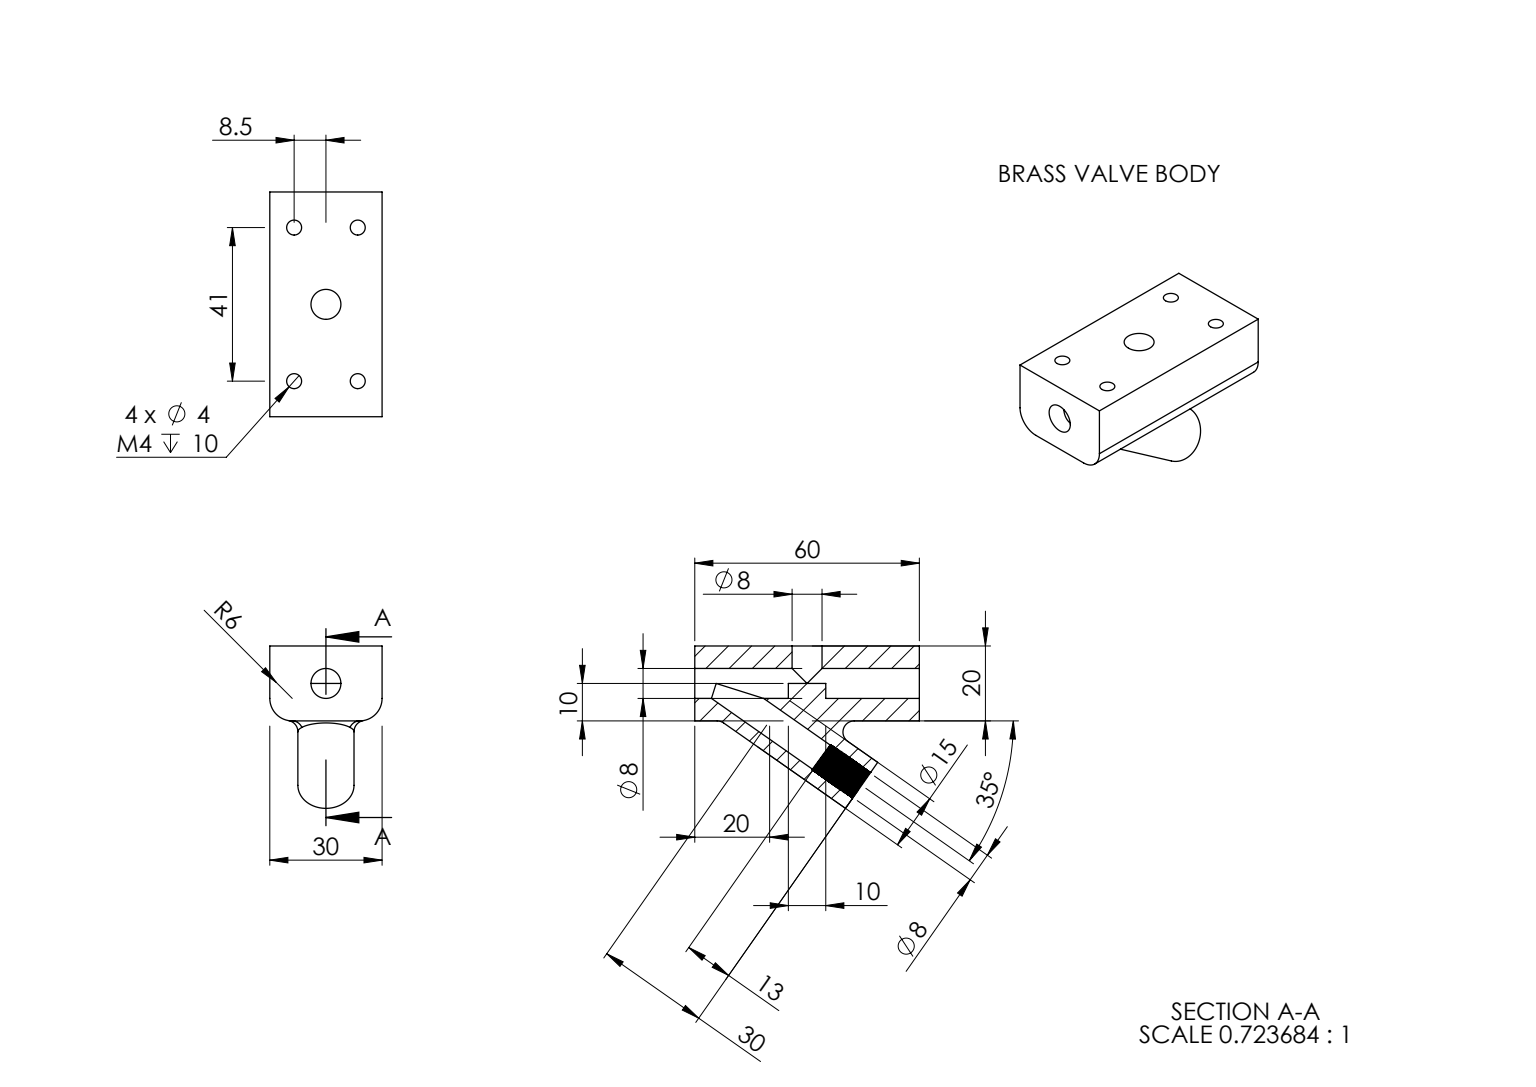
ISO-10303-21;
HEADER;
FILE_DESCRIPTION (('STEP AP214'),
    '1' );
FILE_NAME ('Brass Valve Body.step',
    '2026-10-25T16:39:07',
    ( '' ),
    ( '' ),
    'SwSTEP 2.0',
    'SolidWorks 2026',
    '' );
FILE_SCHEMA (( 'AUTOMOTIVE_DESIGN' ));
ENDSEC;

DATA;
#2=CARTESIAN_POINT ( 'NONE',  ( 2.000000000000004441, -20.45500799277048287, -10.97077568596606056 ) ) ;
#7=CARTESIAN_POINT ( 'NONE',  ( 9.986002763741593569, -9.918550557884699970, 7.302443594976057106 ) ) ;
#8=CARTESIAN_POINT ( 'NONE',  ( 2.121784821875004390, -19.91118585227123816, -10.56187548683408828 ) ) ;
#10=CARTESIAN_POINT ( 'NONE',  ( 3.579096709490575479E-14, -22.86967407583208711, -1.406012196336041020 ) ) ;
#12=ORIENTED_EDGE ( 'NONE', *, *, #11357, .T. ) ;
#15=EDGE_CURVE ( 'NONE', #13968, #17116, #3305, .T. ) ;
#18=FACE_OUTER_BOUND ( 'NONE', #18196, .T. ) ;
#22=CARTESIAN_POINT ( 'NONE',  ( 4.243569643750000786, -23.22272928460757413, -8.884014471503119736 ) ) ;
#27=CARTESIAN_POINT ( 'NONE',  ( -5.330712181944245322E-15, -26.55907985683728967, -5.105836667743160362 ) ) ;
#30=ADVANCED_FACE ( 'NONE', ( #12002 ), #4961, .F. ) ;
#35=CARTESIAN_POINT ( 'NONE',  ( -4.243569643750000786, -19.99636183013295820, -4.276284222377527477 ) ) ;
#38=ORIENTED_EDGE ( 'NONE', *, *, #726, .T. ) ;
#45=ORIENTED_EDGE ( 'NONE', *, *, #5518, .T. ) ;
#46=CARTESIAN_POINT ( 'NONE',  ( -4.243569643750000786, -20.54484429739364515, -5.059598364728879361 ) ) ;
#49=CARTESIAN_POINT ( 'NONE',  ( -2.121784821874996396, -23.22358977219849407, -15.29247854260303718 ) ) ;
#50=( BOUNDED_CURVE ( )  B_SPLINE_CURVE ( 2, ( #611, #13389, #3391, #8936, #1817, #3112, #11902, #16101, #955 ),
 .UNSPECIFIED., .F., .F. ) 
 B_SPLINE_CURVE_WITH_KNOTS ( ( 3, 2, 2, 2, 3 ),
 ( 0.3879310344827586188, 0.3908045977011494476, 0.3965517241379310498, 0.4022988505747126520, 0.4051724137931034808 ),
 .UNSPECIFIED. ) 
 CURVE ( )  GEOMETRIC_REPRESENTATION_ITEM ( )  RATIONAL_B_SPLINE_CURVE ( ( 0.9330127018922194093, 0.9330127018922194093, 1.000000000000000000, 0.8660254037844387076, 1.000000000000000000, 0.8660254037844387076, 1.000000000000000000, 0.9330127018922187432, 0.9330127018922194093 ) ) 
 REPRESENTATION_ITEM ( '' )  );
#53=DIRECTION ( 'NONE',  ( -0.000000000000000000, -0.5735764363510414965, -0.8191520442889950182 ) ) ;
#54=CARTESIAN_POINT ( 'NONE',  ( 4.243569643750003451, -22.48482328119956009, -12.10166559521431573 ) ) ;
#57=CARTESIAN_POINT ( 'NONE',  ( -1.999999999999996225, -18.15353254261686899, -7.683928109263233885 ) ) ;
#61=VECTOR ( 'NONE', #15535, 1000.000000000000000 ) ;
#62=EDGE_CURVE ( 'NONE', #4590, #2518, #8726, .T. ) ;
#63=AXIS2_PLACEMENT_3D ( 'NONE', #11586, #12802, #2984 ) ;
#64=CARTESIAN_POINT ( 'NONE',  ( 3.999999999999996447, -25.24891187463481046, -7.751385191667569785 ) ) ;
#66=EDGE_LOOP ( 'NONE', ( #4791, #2042, #17064, #10532, #9168 ) ) ;
#67=CARTESIAN_POINT ( 'NONE',  ( 2.121784821875004390, -20.71777771588989125, -11.71380804911548701 ) ) ;
#68=CARTESIAN_POINT ( 'NONE',  ( -4.000000000000000888, -26.36843755307278414, -13.37655146490396341 ) ) ;
#72=CARTESIAN_POINT ( 'NONE',  ( 1.071796769724485232, -23.37436616782919074, -2.126787201540221162 ) ) ;
#73=DIRECTION ( 'NONE',  ( -0.000000000000000000, 1.000000000000000000, -0.000000000000000000 ) ) ;
#74=AXIS2_PLACEMENT_3D ( 'NONE', #11287, #9899, #17353 ) ;
#78=CARTESIAN_POINT ( 'NONE',  ( 4.243569643749996345, -23.73478956620236957, -5.343822230353133307 ) ) ;
#79=ADVANCED_FACE ( 'NONE', ( #10984 ), #15448, .F. ) ;
#82=ORIENTED_EDGE ( 'NONE', *, *, #14672, .T. ) ;
#83=ORIENTED_EDGE ( 'NONE', *, *, #13971, .F. ) ;
#84=DIRECTION ( 'NONE',  ( -0.000000000000000000, 1.000000000000000000, -0.000000000000000000 ) ) ;
#89=CARTESIAN_POINT ( 'NONE',  ( 3.999999999999996447, -27.63642379165096941, -11.16110557702727668 ) ) ;
#93=CARTESIAN_POINT ( 'NONE',  ( 1.999999999999994449, -26.47440569391090648, -7.488412793402255296 ) ) ;
#94=VERTEX_POINT ( 'NONE', #4123 ) ;
#95=CARTESIAN_POINT ( 'NONE',  ( 0.000000000000000000, 5.977523610840987267, 32.81826849749789687 ) ) ;
#97=CARTESIAN_POINT ( 'NONE',  ( 9.570744302495992173, -9.974069202854233041, -0.5947597794661263482 ) ) ;
#98=CARTESIAN_POINT ( 'NONE',  ( -4.243569643749998122, -21.36634923031502353, -10.50431910885077791 ) ) ;
#101=CARTESIAN_POINT ( 'NONE',  ( 1.071796769724504328, -22.85814737511324424, -1.389550361680131685 ) ) ;
#102=CARTESIAN_POINT ( 'NONE',  ( 4.000000000000000888, -19.98022999250811793, -4.253245570628513939 ) ) ;
#103=EDGE_CURVE ( 'NONE', #5353, #12502, #9927, .T. ) ;
#104=ORIENTED_EDGE ( 'NONE', *, *, #5539, .F. ) ;
#105=EDGE_LOOP ( 'NONE', ( #9337, #11121, #10529, #10635, #17849 ) ) ;
#110=EDGE_LOOP ( 'NONE', ( #10063, #7100, #15621, #8878 ) ) ;
#112=CARTESIAN_POINT ( 'NONE',  ( 4.243569643750000786, -23.48083868096554028, -9.252632891433169249 ) ) ;
#116=CARTESIAN_POINT ( 'NONE',  ( 4.898587196589413815E-16, 2.700915433685006750, 35.11257424290206330 ) ) ;
#117=VECTOR ( 'NONE', #8182, 1000.000000000000000 ) ;
#118=CARTESIAN_POINT ( 'NONE',  ( -2.121784821874996396, -19.38421250137371388, -9.809279546143578443 ) ) ;
#119=CARTESIAN_POINT ( 'NONE',  ( -2.526502195916607629, -15.31622431266957207, -9.916727303590223030 ) ) ;
#120=CARTESIAN_POINT ( 'NONE',  ( -5.577813053751546416E-15, -24.16022105762193206, -3.249104295986281699 ) ) ;
#122=CARTESIAN_POINT ( 'NONE',  ( 4.243569643749996345, -22.92819770258371292, -4.191889668071731911 ) ) ;
#123=CARTESIAN_POINT ( 'NONE',  ( 1.071796769724485454, -21.36111765121935235, -13.19914471043622228 ) ) ;
#125=ORIENTED_EDGE ( 'NONE', *, *, #9998, .T. ) ;
#127=CARTESIAN_POINT ( 'NONE',  ( -5.577813053751546416E-15, -25.38624068961733826, -5.000041789647243107 ) ) ;
#129=CYLINDRICAL_SURFACE ( 'NONE', #10158, 6.000000000000000000 ) ;
#133=CARTESIAN_POINT ( 'NONE',  ( 2.121784821875004390, -17.62046495959427261, -7.290387009954915953 ) ) ;
#135=CARTESIAN_POINT ( 'NONE',  ( -4.000000000000000888, -19.85117529432912775, -4.068936360663492735 ) ) ;
#138=CARTESIAN_POINT ( 'NONE',  ( -4.243569643749998122, -23.17311500482080433, -13.08464804836111206 ) ) ;
#143=LINE ( 'NONE', #14051, #16513 ) ;
#144=CARTESIAN_POINT ( 'NONE',  ( 4.243569643749996345, -26.79983864795324422, -9.721165967022450616 ) ) ;
#146=CARTESIAN_POINT ( 'NONE',  ( -1.999999999999996225, -17.37920435354295989, -6.578072849473089789 ) ) ;
#150=EDGE_CURVE ( 'NONE', #12707, #13230, #14438, .T. ) ;
#151=CARTESIAN_POINT ( 'NONE',  ( 0.000000000000000000, 5.977523610840987267, 32.81826849749789687 ) ) ;
#157=CARTESIAN_POINT ( 'NONE',  ( -2.121784821874996396, -21.44908767223746437, -12.75822690558396033 ) ) ;
#159=VERTEX_POINT ( 'NONE', #2476 ) ;
#161=CARTESIAN_POINT ( 'NONE',  ( 3.999999999999995559, 2.343145750507624747, 2.343145750507618086 ) ) ;
#162=CARTESIAN_POINT ( 'NONE',  ( -5.577813053751546416E-15, -26.16056887869124381, -6.105897049437384538 ) ) ;
#163=CARTESIAN_POINT ( 'NONE',  ( 1.071796769724485232, -25.37471398889850605, -4.983579954991325778 ) ) ;
#164=CARTESIAN_POINT ( 'NONE',  ( -5.577813053751546416E-15, -29.06429958842333505, -10.25285427465718868 ) ) ;
#166=CARTESIAN_POINT ( 'NONE',  ( 2.121784821874994176, -23.98544242790896774, -3.566046559362932467 ) ) ;
#171=CYLINDRICAL_SURFACE ( 'NONE', #7169, 2.000000000000001776 ) ;
#172=LINE ( 'NONE', #7581, #17268 ) ;
#177=VERTEX_POINT ( 'NONE', #8106 ) ;
#179=CARTESIAN_POINT ( 'NONE',  ( -3.999999999999997335, -21.07824655387797819, -9.847693641197304615 ) ) ;
#180=ORIENTED_EDGE ( 'NONE', *, *, #14181, .F. ) ;
#184=CARTESIAN_POINT ( 'NONE',  ( -9.604277560388482016, -9.971758527880211886, 12.06915245473052778 ) ) ;
#185=CARTESIAN_POINT ( 'NONE',  ( 4.243569643750003451, -19.90372931761987019, -8.415481395913838369 ) ) ;
#194=CARTESIAN_POINT ( 'NONE',  ( 1.533898589781675205E-14, -27.70922525683905846, -8.317607569017670954 ) ) ;
#199=CARTESIAN_POINT ( 'NONE',  ( 4.730628863548789710E-15, -18.62809540513275408, -10.86517747810410306 ) ) ;
#203=FACE_OUTER_BOUND ( 'NONE', #11493, .T. ) ;
#205=DIRECTION ( 'NONE',  ( 0.000000000000000000, 0.8191520442889952403, -0.5735764363510413855 ) ) ;
#206=CARTESIAN_POINT ( 'NONE',  ( -4.243569643750005227, -25.11137301344485451, -7.309787136646725081 ) ) ;
#207=EDGE_CURVE ( 'NONE', #12141, #13551, #11942, .T. ) ;
#208=CYLINDRICAL_SURFACE ( 'NONE', #2997, 2.000000000000001776 ) ;
#211=CARTESIAN_POINT ( 'NONE',  ( -4.371749249414769167, -10.00000000000000178, -10.94697576041360954 ) ) ;
#212=DIRECTION ( 'NONE',  ( 0.000000000000000000, 0.8191520442889952403, -0.5735764363510413855 ) ) ;
#214=VECTOR ( 'NONE', #7659, 1000.000000000000000 ) ;
#215=CARTESIAN_POINT ( 'NONE',  ( 4.730628863548789710E-15, -16.82132963062697684, -8.284848538593767131 ) ) ;
#217=CARTESIAN_POINT ( 'NONE',  ( 2.000000000000004441, -17.68033198262726913, -7.008127672724814516 ) ) ;
#218=VERTEX_POINT ( 'NONE', #12642 ) ;
#220=CARTESIAN_POINT ( 'NONE',  ( 4.243569643749996345, -28.60660442245902146, -12.30149490653278121 ) ) ;
#223=CARTESIAN_POINT ( 'NONE',  ( -8.999999999999996447, -10.00000000000000000, 15.14468620625656925 ) ) ;
#224=DIRECTION ( 'NONE',  ( -6.162975822039154730E-33, 0.5735764363510414965, 0.8191520442889950182 ) ) ;
#227=ORIENTED_EDGE ( 'NONE', *, *, #6831, .F. ) ;
#228=CARTESIAN_POINT ( 'NONE',  ( 2.121784821875004390, -17.36235556323629936, -6.921768590024867329 ) ) ;
#230=CARTESIAN_POINT ( 'NONE',  ( 3.064182432158234271, -21.85725826261086624, -2.451265441397198153 ) ) ;
#233=CARTESIAN_POINT ( 'NONE',  ( 4.243569643749997233, -27.57416683702714622, -10.82702122681259205 ) ) ;
#235=CYLINDRICAL_SURFACE ( 'NONE', #4146, 4.000000000000000000 ) ;
#236=DIRECTION ( 'NONE',  ( 0.000000000000000000, 0.8191520442889952403, -0.5735764363510413855 ) ) ;
#237=CARTESIAN_POINT ( 'NONE',  ( -4.243569643750000786, -24.64233096457639505, -10.91141578111838584 ) ) ;
#240=CARTESIAN_POINT ( 'NONE',  ( -5.279047395330986450E-15, -24.40900471032784935, -2.525555542035599288 ) ) ;
#244=VERTEX_POINT ( 'NONE', #11334 ) ;
#246=FACE_OUTER_BOUND ( 'NONE', #4639, .T. ) ;
#248=CARTESIAN_POINT ( 'NONE',  ( 1.071796769724504328, -26.66526097068834034, -6.826672054641570675 ) ) ;
#251=CARTESIAN_POINT ( 'NONE',  ( 2.121784821874994176, -27.34086458056255964, -8.358086018453551702 ) ) ;
#257=CARTESIAN_POINT ( 'NONE',  ( 4.243569643750003451, -23.54952454117618288, -13.62221657742576397 ) ) ;
#259=CYLINDRICAL_SURFACE ( 'NONE', #5612, 4.000000000000000000 ) ;
#261=CARTESIAN_POINT ( 'NONE',  ( -4.243569643749997233, -19.84995652671195998, -8.338685891761748792 ) ) ;
#267=ADVANCED_FACE ( 'NONE', ( #8551 ), #11828, .T. ) ;
#269=VERTEX_POINT ( 'NONE', #1927 ) ;
#271=CARTESIAN_POINT ( 'NONE',  ( 4.898587196589413815E-16, 2.700915433685006750, 35.11257424290206330 ) ) ;
#280=CARTESIAN_POINT ( 'NONE',  ( -4.000000000000004441, -24.81872954737152170, -7.137021158450828295 ) ) ;
#281=ORIENTED_EDGE ( 'NONE', *, *, #17408, .F. ) ;
#285=CARTESIAN_POINT ( 'NONE',  ( -9.667409818421043965, -9.963321348641603237, 0.1620040674102612710 ) ) ;
#287=CARTESIAN_POINT ( 'NONE',  ( 4.243569643749997233, -22.92819770258370582, -4.191889668071731911 ) ) ;
#288=AXIS2_PLACEMENT_3D ( 'NONE', #11365, #11189, #12854 ) ;
#292=ORIENTED_EDGE ( 'NONE', *, *, #6272, .T. ) ;
#299=CARTESIAN_POINT ( 'NONE',  ( -1.071796769724494114, -29.59204508185809956, -11.00655294917319971 ) ) ;
#300=CARTESIAN_POINT ( 'NONE',  ( 4.730628863548789710E-15, -19.14431419784869348, -11.60241431796419853 ) ) ;
#305=CARTESIAN_POINT ( 'NONE',  ( -4.000000000000000888, -27.07823839235225094, -14.39025211870482934 ) ) ;
#306=CARTESIAN_POINT ( 'NONE',  ( 4.243569643750003451, -20.19410238852258743, -8.830177118335141628 ) ) ;
#307=DIRECTION ( 'NONE',  ( -0.000000000000000000, -0.5735764363510414965, -0.8191520442889950182 ) ) ;
#308=CARTESIAN_POINT ( 'NONE',  ( -4.193264170084745501, -10.00000000000000178, -2.677076674081568797 ) ) ;
#312=ORIENTED_EDGE ( 'NONE', *, *, #6152, .T. ) ;
#313=CARTESIAN_POINT ( 'NONE',  ( -5.330712181944245322E-15, -24.20383161507082193, -1.742193585881474771 ) ) ;
#315=FACE_OUTER_BOUND ( 'NONE', #13052, .T. ) ;
#316=DIRECTION ( 'NONE',  ( 0.000000000000000000, 0.000000000000000000, 1.000000000000000000 ) ) ;
#317=VERTEX_POINT ( 'NONE', #16194 ) ;
#320=CARTESIAN_POINT ( 'NONE',  ( 2.121784821874994176, -29.88969486959749844, -11.99819291526277532 ) ) ;
#324=CARTESIAN_POINT ( 'NONE',  ( 3.820650143297091184, -10.00000000000057376, -3.109998371641698345 ) ) ;
#326=CARTESIAN_POINT ( 'NONE',  ( -2.121784821874996396, -17.57744672686793308, -7.228950606633243403 ) ) ;
#329=CARTESIAN_POINT ( 'NONE',  ( 2.121784821874994176, -29.66384914778427628, -11.67565179782398310 ) ) ;
#330=( BOUNDED_CURVE ( )  B_SPLINE_CURVE ( 2, ( #8971, #16213, #4605, #6375, #1755, #13228, #14645, #544, #6189 ),
 .UNSPECIFIED., .F., .T. ) 
 B_SPLINE_CURVE_WITH_KNOTS ( ( 3, 2, 2, 2, 3 ),
 ( 0.2844827586206896686, 0.2873563218390804419, 0.2931034482758620441, 0.2988505747126437018, 0.3017241379310345306 ),
 .UNSPECIFIED. ) 
 CURVE ( )  GEOMETRIC_REPRESENTATION_ITEM ( )  RATIONAL_B_SPLINE_CURVE ( ( 0.9330127018922194093, 0.9330127018922200755, 1.000000000000000000, 0.8660254037844387076, 1.000000000000000000, 0.8660254037844387076, 1.000000000000000000, 0.9330127018922187432, 0.9330127018922194093 ) ) 
 REPRESENTATION_ITEM ( '' )  );
#332=CARTESIAN_POINT ( 'NONE',  ( 4.730628863548789710E-15, -20.95107997235447073, -14.18274325747453268 ) ) ;
#333=LINE ( 'NONE', #8939, #3459 ) ;
#336=CARTESIAN_POINT ( 'NONE',  ( 4.243569643750000786, -24.77138566275538523, -11.09572499108340793 ) ) ;
#337=EDGE_CURVE ( 'NONE', #1667, #17584, #9315, .T. ) ;
#339=CARTESIAN_POINT ( 'NONE',  ( -3.999999999999997335, -18.81978933645070384, -6.622282467816152263 ) ) ;
#342=EDGE_CURVE ( 'NONE', #5337, #15144, #10613, .T. ) ;
#349=ORIENTED_EDGE ( 'NONE', *, *, #16662, .F. ) ;
#350=CARTESIAN_POINT ( 'NONE',  ( 4.243569643749997233, -25.54155534070815392, -7.924151169863465682 ) ) ;
#352=ORIENTED_EDGE ( 'NONE', *, *, #16895, .T. ) ;
#355=CARTESIAN_POINT ( 'NONE',  ( -2.121784821875005722, -27.90010160600482081, -9.156759261635325942 ) ) ;
#357=CARTESIAN_POINT ( 'NONE',  ( -14.99999999999999645, 10.00000000000000000, -30.00000000000000000 ) ) ;
#358=CARTESIAN_POINT ( 'NONE',  ( 3.999999999999996447, -24.47458368556090491, -6.645529931877427465 ) ) ;
#359=CARTESIAN_POINT ( 'NONE',  ( -4.243569643749997233, -19.07562833763805088, -7.232830631971606472 ) ) ;
#362=DIRECTION ( 'NONE',  ( 0.000000000000000000, 0.8191520442889952403, -0.5735764363510413855 ) ) ;
#364=ORIENTED_EDGE ( 'NONE', *, *, #9762, .T. ) ;
#365=CARTESIAN_POINT ( 'NONE',  ( -3.999999999999997335, -18.56167994009273059, -6.253664047886104527 ) ) ;
#366=FACE_OUTER_BOUND ( 'NONE', #5608, .T. ) ;
#373=CARTESIAN_POINT ( 'NONE',  ( 4.713407268011036227E-15, -18.45518598442047420, -10.12789282444123451 ) ) ;
#381=CARTESIAN_POINT ( 'NONE',  ( 9.178358240570380744, -10.00000000000000000, -2.937375903338058869 ) ) ;
#383=CARTESIAN_POINT ( 'NONE',  ( -4.243569643750004339, -23.78856235711027267, -5.420617734505230878 ) ) ;
#387=ORIENTED_EDGE ( 'NONE', *, *, #14732, .T. ) ;
#397=CARTESIAN_POINT ( 'NONE',  ( -2.121784821875005722, -23.99619698609053842, -3.581405660193354379 ) ) ;
#400=CARTESIAN_POINT ( 'NONE',  ( 1.999999999999994449, -22.66729209833581749, -2.051291100440815640 ) ) ;
#402=CARTESIAN_POINT ( 'NONE',  ( 4.730628863548789710E-15, -18.91846847603547133, -11.27987320052540809 ) ) ;
#403=DIRECTION ( 'NONE',  ( -1.000000000000000000, 0.000000000000000000, 0.000000000000000000 ) ) ;
#405=VECTOR ( 'NONE', #13165, 1000.000000000000000 ) ;
#407=FACE_OUTER_BOUND ( 'NONE', #5763, .T. ) ;
#408=FACE_OUTER_BOUND ( 'NONE', #14459, .T. ) ;
#412=CARTESIAN_POINT ( 'NONE',  ( -6.938893903907228378E-15, 6.938893903907228378E-15, 30.00000000000000000 ) ) ;
#413=( NAMED_UNIT ( * ) SI_UNIT ( $, .STERADIAN. ) SOLID_ANGLE_UNIT ( ) );
#416=CARTESIAN_POINT ( 'NONE',  ( -2.121784821874996396, -22.44926158312459208, -14.18662328281289398 ) ) ;
#418=VECTOR ( 'NONE', #12172, 1000.000000000000000 ) ;
#419=DIRECTION ( 'NONE',  ( -0.000000000000000000, -0.5735764363510414965, -0.8191520442889950182 ) ) ;
#421=ORIENTED_EDGE ( 'NONE', *, *, #3365, .T. ) ;
#423=CARTESIAN_POINT ( 'NONE',  ( -2.121784821874996396, -24.03018163581715072, -16.44441110488443769 ) ) ;
#425=CARTESIAN_POINT ( 'NONE',  ( -4.243569643750004339, -27.66020330247980041, -10.94989403345594425 ) ) ;
#428=CARTESIAN_POINT ( 'NONE',  ( 4.730628863548789710E-15, -20.95107997235447073, -14.18274325747453268 ) ) ;
#430=CARTESIAN_POINT ( 'NONE',  ( -2.000000000000005773, -23.74274791649401095, -3.587201183482685352 ) ) ;
#432=ORIENTED_EDGE ( 'NONE', *, *, #4382, .T. ) ;
#434=CARTESIAN_POINT ( 'NONE',  ( -1.661723472263481630E-14, -21.09148155414254688, -12.81406445585025544 ) ) ;
#435=CARTESIAN_POINT ( 'NONE',  ( -1.999999999999996225, -22.79950167706030228, -14.31905966800409402 ) ) ;
#438=( BOUNDED_CURVE ( )  B_SPLINE_CURVE ( 2, ( #16331, #7967, #17558, #7596, #9268, #13622, #17653, #13255, #13442 ),
 .UNSPECIFIED., .F., .T. ) 
 B_SPLINE_CURVE_WITH_KNOTS ( ( 3, 2, 2, 2, 3 ),
 ( 0.5603448275862069616, 0.5632183908045976795, 0.5689655172413793371, 0.5747126436781608838, 0.5775862068965517127 ),
 .UNSPECIFIED. ) 
 CURVE ( )  GEOMETRIC_REPRESENTATION_ITEM ( )  RATIONAL_B_SPLINE_CURVE ( ( 0.9330127018922194093, 0.9330127018922206306, 1.000000000000000000, 0.8660254037844387076, 1.000000000000000000, 0.8660254037844387076, 1.000000000000000000, 0.9330127018922194093, 0.9330127018922194093 ) ) 
 REPRESENTATION_ITEM ( '' )  );
#439=ORIENTED_EDGE ( 'NONE', *, *, #5539, .T. ) ;
#440=CARTESIAN_POINT ( 'NONE',  ( -4.243569643750000786, -24.15837584640520674, -10.22025624374954766 ) ) ;
#446=CARTESIAN_POINT ( 'NONE',  ( -2.121784821875005722, -29.19064858779466221, -10.99985136128556462 ) ) ;
#447=CARTESIAN_POINT ( 'NONE',  ( -1.071796769724491671, -22.11239243885559347, -14.27207630091453261 ) ) ;
#448=DIRECTION ( 'NONE',  ( -0.000000000000000000, -0.5735764363510414965, -0.8191520442889950182 ) ) ;
#449=CARTESIAN_POINT ( 'NONE',  ( 2.000000000000004441, -19.68067980369657377, -9.864920426175917356 ) ) ;
#450=CARTESIAN_POINT ( 'NONE',  ( 2.121784821874994176, -24.75977061698287329, -4.671901819153075230 ) ) ;
#451=VERTEX_POINT ( 'NONE', #17514 ) ;
#453=CARTESIAN_POINT ( 'NONE',  ( 1.071796769724485232, -25.63282338525647575, -5.352198374921374402 ) ) ;
#455=ORIENTED_EDGE ( 'NONE', *, *, #6941, .T. ) ;
#457=DIRECTION ( 'NONE',  ( 0.000000000000000000, 0.8191520442889952403, -0.5735764363510413855 ) ) ;
#458=DIRECTION ( 'NONE',  ( 0.000000000000000000, 0.8191520442889952403, -0.5735764363510413855 ) ) ;
#463=ORIENTED_EDGE ( 'NONE', *, *, #2191, .T. ) ;
#465=CARTESIAN_POINT ( 'NONE',  ( -5.279047395330986450E-15, -26.40935253139716110, -5.382348295486703016 ) ) ;
#470=CARTESIAN_POINT ( 'NONE',  ( -4.243569643750000786, -21.28690881192279960, -6.119376322027766157 ) ) ;
#472=CARTESIAN_POINT ( 'NONE',  ( 1.071796769724495224, -16.65062116698148031, -6.471858545706086652 ) ) ;
#476=CARTESIAN_POINT ( 'NONE',  ( 4.253155871621279616, -10.96494312749350186, 19.45022984308079472 ) ) ;
#478=DIRECTION ( 'NONE',  ( -0.000000000000000000, -0.5735764363510414965, -0.8191520442889950182 ) ) ;
#479=CARTESIAN_POINT ( 'NONE',  ( 4.898587196589417759E-16, -3.999999999999993339, 25.54267522293723758 ) ) ;
#485=CARTESIAN_POINT ( 'NONE',  ( 4.730628863548789710E-15, -16.82132963062697684, -8.284848538593767131 ) ) ;
#488=CARTESIAN_POINT ( 'NONE',  ( 4.243569643749997233, -28.89697749336173871, -12.71619062895408803 ) ) ;
#489=CARTESIAN_POINT ( 'NONE',  ( -4.000000000000004441, -28.17415170002511360, -11.92906061754144886 ) ) ;
#491=ADVANCED_FACE ( 'NONE', ( #892 ), #2289, .F. ) ;
#492=CARTESIAN_POINT ( 'NONE',  ( -4.243569643750000786, -21.83539127918348299, -6.902690464379118040 ) ) ;
#495=CARTESIAN_POINT ( 'NONE',  ( -0.3267727178421339085, -10.00000000000000178, -5.052762561669631225 ) ) ;
#496=FACE_OUTER_BOUND ( 'NONE', #17631, .T. ) ;
#499=ORIENTED_EDGE ( 'NONE', *, *, #6216, .T. ) ;
#500=CARTESIAN_POINT ( 'NONE',  ( 2.121784821874994176, -22.92074116793234140, -2.045495577151484223 ) ) ;
#501=CARTESIAN_POINT ( 'NONE',  ( -6.428571428571423496, -11.73421655796351892, 14.25837509840161310 ) ) ;
#502=DIRECTION ( 'NONE',  ( -0.000000000000000000, 1.000000000000000000, -0.000000000000000000 ) ) ;
#503=ORIENTED_EDGE ( 'NONE', *, *, #11462, .F. ) ;
#505=( NAMED_UNIT ( * ) SI_UNIT ( $, .STERADIAN. ) SOLID_ANGLE_UNIT ( ) );
#506=EDGE_CURVE ( 'NONE', #17004, #8682, #13300, .T. ) ;
#507=CIRCLE ( 'NONE', #12335, 4.000000000000000000 ) ;
#508=CARTESIAN_POINT ( 'NONE',  ( -4.243569643750000786, -26.19098734272420614, -13.12312630069867225 ) ) ;
#511=CARTESIAN_POINT ( 'NONE',  ( 4.757769075324610242, -14.90261145393154862, -7.125238870422657911 ) ) ;
#514=CARTESIAN_POINT ( 'NONE',  ( 2.121784821875004390, -23.29887167946958115, -15.39999224841596437 ) ) ;
#517=CARTESIAN_POINT ( 'NONE',  ( 2.121784821875004390, -21.20173283406107956, -12.40496758648432518 ) ) ;
#519=CARTESIAN_POINT ( 'NONE',  ( -1.071796769724486786, -16.95020451169621722, -6.899707902313577002 ) ) ;
#522=CARTESIAN_POINT ( 'NONE',  ( -5.330712181944245322E-15, -27.81736316408238707, -6.902851464902143519 ) ) ;
#523=CARTESIAN_POINT ( 'NONE',  ( -5.577813053751546416E-15, -25.96698683212770931, -5.829433235496615850 ) ) ;
#529=CARTESIAN_POINT ( 'NONE',  ( 2.000000000000004441, -22.58441051342866857, -14.01187765139572150 ) ) ;
#530=CARTESIAN_POINT ( 'NONE',  ( 1.071796769724504328, -23.63247556418714979, -2.495405621470275559 ) ) ;
#534=CARTESIAN_POINT ( 'NONE',  ( 4.243569643750000786, -22.99688356279435197, -8.561473354064329300 ) ) ;
#536=ORIENTED_EDGE ( 'NONE', *, *, #1348, .T. ) ;
#540=CARTESIAN_POINT ( 'NONE',  ( -4.243569643749997233, -23.97970686843945742, -14.23658061064251257 ) ) ;
#541=CARTESIAN_POINT ( 'NONE',  ( 1.999999999999994449, -29.57171845020653222, -11.91183383256282724 ) ) ;
#542=DIRECTION ( 'NONE',  ( -1.000000000000000000, -0.000000000000000000, -0.000000000000000000 ) ) ;
#544=CARTESIAN_POINT ( 'NONE',  ( -1.071796769724486564, -28.23697075027383008, -9.071306243533678426 ) ) ;
#545=CARTESIAN_POINT ( 'NONE',  ( 4.243569643750000786, -20.15768020285669593, -4.506670734833804204 ) ) ;
#547=CARTESIAN_POINT ( 'NONE',  ( -4.000000000000000888, -23.52923419313512454, -9.321748845673438311 ) ) ;
#548=EDGE_CURVE ( 'NONE', #8360, #17559, #7326, .T. ) ;
#549=CARTESIAN_POINT ( 'NONE',  ( 4.000000000000000888, -22.88396070224021273, -8.400202795848317194 ) ) ;
#553=( BOUNDED_CURVE ( )  B_SPLINE_CURVE ( 2, ( #11093, #6833, #15203, #6742, #11181, #13792, #1101, #18087, #9699 ),
 .UNSPECIFIED., .F., .T. ) 
 B_SPLINE_CURVE_WITH_KNOTS ( ( 3, 2, 2, 2, 3 ),
 ( 0.9051724137931034253, 0.9080459770114942541, 0.9137931034482759118, 0.9195402298850574585, 0.9224137931034482873 ),
 .UNSPECIFIED. ) 
 CURVE ( )  GEOMETRIC_REPRESENTATION_ITEM ( )  RATIONAL_B_SPLINE_CURVE ( ( 0.9330127018922194093, 0.9330127018922194093, 1.000000000000000000, 0.8660254037844387076, 1.000000000000000000, 0.8660254037844387076, 1.000000000000000000, 0.9330127018922194093, 0.9330127018922194093 ) ) 
 REPRESENTATION_ITEM ( '' )  );
#556=DIRECTION ( 'NONE',  ( 0.000000000000000000, 0.8191520442889952403, -0.5735764363510413855 ) ) ;
#560=EDGE_CURVE ( 'NONE', #14256, #10497, #11069, .T. ) ;
#566=CARTESIAN_POINT ( 'NONE',  ( 4.713407268011036227E-15, -18.97140477713641005, -10.86512966430133176 ) ) ;
#570=CARTESIAN_POINT ( 'NONE',  ( 1.071796769724485454, -20.52226211235100806, -12.00113484465680358 ) ) ;
#571=CARTESIAN_POINT ( 'NONE',  ( -4.243569643749998122, -19.55958345580924629, -7.923990169340444645 ) ) ;
#574=CARTESIAN_POINT ( 'NONE',  ( 3.999999999999996447, -28.41075198072487140, -12.26696083681741989 ) ) ;
#576=ORIENTED_EDGE ( 'NONE', *, *, #8996, .F. ) ;
#577=CARTESIAN_POINT ( 'NONE',  ( 2.531783071939769592, -10.67720498481739355, 21.39218517664858510 ) ) ;
#578=CARTESIAN_POINT ( 'NONE',  ( 0.000000000000000000, 5.977523610840987267, 32.81826849749789687 ) ) ;
#581=ORIENTED_EDGE ( 'NONE', *, *, #2191, .F. ) ;
#584=CARTESIAN_POINT ( 'NONE',  ( 4.243569643749996345, -23.18630709894168263, -4.560508088001781424 ) ) ;
#587=CARTESIAN_POINT ( 'NONE',  ( 4.243569643749997233, -28.38075870064580286, -11.97895378909399078 ) ) ;
#588=CARTESIAN_POINT ( 'NONE',  ( 1.999999999999994449, -29.31360905384856608, -11.54321541263277950 ) ) ;
#589=VECTOR ( 'NONE', #2601, 1000.000000000000000 ) ;
#590=CARTESIAN_POINT ( 'NONE',  ( 2.121784821875004390, -18.13668375231020846, -8.027623849815011425 ) ) ;
#595=ORIENTED_EDGE ( 'NONE', *, *, #1110, .F. ) ;
#598=CARTESIAN_POINT ( 'NONE',  ( 4.299564228933482956E-15, -17.41342265533655009, -7.561251970840314307 ) ) ;
#600=ORIENTED_EDGE ( 'NONE', *, *, #8861, .F. ) ;
#604=CARTESIAN_POINT ( 'NONE',  ( 4.730628863548789710E-15, -22.24162695414431212, -16.02583535712476959 ) ) ;
#607=CARTESIAN_POINT ( 'NONE',  ( 2.121784821875004390, -22.00832469767973620, -13.55690014876572569 ) ) ;
#609=EDGE_CURVE ( 'NONE', #1376, #8485, #13946, .T. ) ;
#611=CARTESIAN_POINT ( 'NONE',  ( 4.299564228933482956E-15, -21.02695420434810814, -12.72190984986098172 ) ) ;
#613=CARTESIAN_POINT ( 'NONE',  ( 2.121784821874994176, -27.05049150965984595, -7.943390296032248443 ) ) ;
#615=ADVANCED_FACE ( 'NONE', ( #13762 ), #4118, .F. ) ;
#618=CARTESIAN_POINT ( 'NONE',  ( 4.243569643749996345, -25.25118226980542602, -7.509455447442161535 ) ) ;
#619=ORIENTED_EDGE ( 'NONE', *, *, #1520, .F. ) ;
#620=CYLINDRICAL_SURFACE ( 'NONE', #17533, 4.000000000000000000 ) ;
#621=CARTESIAN_POINT ( 'NONE',  ( 2.610817454768295409, -22.11373505648317916, -1.875566028523329098 ) ) ;
#625=DIRECTION ( 'NONE',  ( -0.000000000000000000, -0.5735764363510414965, -0.8191520442889950182 ) ) ;
#627=AXIS2_PLACEMENT_3D ( 'NONE', #9610, #15282, #8214 ) ;
#632=CARTESIAN_POINT ( 'NONE',  ( 4.243569643750000786, -22.48066477007841613, -7.824236514204232940 ) ) ;
#637=CARTESIAN_POINT ( 'NONE',  ( -4.243569643750005227, -26.91813878795063886, -9.890116076157061897 ) ) ;
#638=CARTESIAN_POINT ( 'NONE',  ( -6.158835246850665095E-15, -22.12391913957442213, -14.28853813557044639 ) ) ;
#639=B_SPLINE_CURVE_WITH_KNOTS ( 'NONE', 1,
 ( #5800, #5891 ),
 .UNSPECIFIED., .F., .F.,
 ( 2, 2 ),
 ( 0.000000000000000000, 1.000000000000000000 ),
 .UNSPECIFIED. ) ;
#640=AXIS2_PLACEMENT_3D ( 'NONE', #16166, #307, #1699 ) ;
#641=CARTESIAN_POINT ( 'NONE',  ( 7.381087143211832569, -10.35722647083040826, 4.976872143527621084 ) ) ;
#642=CARTESIAN_POINT ( 'NONE',  ( -4.243569643750000786, -26.96531553179811169, -14.22898156048881724 ) ) ;
#643=ORIENTED_EDGE ( 'NONE', *, *, #13613, .T. ) ;
#645=CARTESIAN_POINT ( 'NONE',  ( 1.999999999999994449, -26.02271425098940938, -6.843330559531437984 ) ) ;
#647=ORIENTED_EDGE ( 'NONE', *, *, #2644, .T. ) ;
#649=CYLINDRICAL_SURFACE ( 'NONE', #8066, 4.000000000000000000 ) ;
#656=CARTESIAN_POINT ( 'NONE',  ( -2.000000000000005773, -24.45254875577348130, -4.600901837283550400 ) ) ;
#657=ORIENTED_EDGE ( 'NONE', *, *, #883, .F. ) ;
#661=CARTESIAN_POINT ( 'NONE',  ( -2.121784821875005722, -23.22186879701663642, -2.475550400403212503 ) ) ;
#662=( BOUNDED_CURVE ( )  B_SPLINE_CURVE ( 2, ( #13922, #1231, #6865, #12609, #13733, #12521, #9559, #14007, #12431 ),
 .UNSPECIFIED., .F., .F. ) 
 B_SPLINE_CURVE_WITH_KNOTS ( ( 3, 2, 2, 2, 3 ),
 ( 0.3534482758620690057, 0.3563218390804597790, 0.3620689655172413812, 0.3678160919540229834, 0.3706896551724138122 ),
 .UNSPECIFIED. ) 
 CURVE ( )  GEOMETRIC_REPRESENTATION_ITEM ( )  RATIONAL_B_SPLINE_CURVE ( ( 0.9330127018922194093, 0.9330127018922200755, 1.000000000000000000, 0.8660254037844387076, 1.000000000000000000, 0.8660254037844387076, 1.000000000000000000, 0.9330127018922187432, 0.9330127018922194093 ) ) 
 REPRESENTATION_ITEM ( '' )  );
#663=CARTESIAN_POINT ( 'NONE',  ( 2.121784821874994176, -27.34086458056255964, -8.358086018453551702 ) ) ;
#665=CARTESIAN_POINT ( 'NONE',  ( 2.170367169212293224, -29.75460566901168491, -12.32900594437920816 ) ) ;
#666=EDGE_LOOP ( 'NONE', ( #3881, #11701, #9259, #14886 ) ) ;
#667=CARTESIAN_POINT ( 'NONE',  ( -4.772237607920192026, -11.09252097142725901, 18.58920227068528419 ) ) ;
#670=CARTESIAN_POINT ( 'NONE',  ( 2.121784821875004390, -24.07319986854348670, -16.50584750820610580 ) ) ;
#671=EDGE_LOOP ( 'NONE', ( #1237, #16466, #3525, #5028 ) ) ;
#673=CARTESIAN_POINT ( 'NONE',  ( 3.939448708636003271, -26.33660243321148897, -14.75747596281047436 ) ) ;
#674=CARTESIAN_POINT ( 'NONE',  ( -5.330712181944245322E-15, -24.97815980414473103, -2.848048845671618423 ) ) ;
#679=CARTESIAN_POINT ( 'NONE',  ( -4.243569643750000786, -26.99757920634285924, -14.27505886298007276 ) ) ;
#680=CARTESIAN_POINT ( 'NONE',  ( -2.000000000000005773, -28.58229909750097875, -10.49879655616431506 ) ) ;
#682=CARTESIAN_POINT ( 'NONE',  ( 4.243569643750000786, -21.96444597736247673, -7.086999674344137468 ) ) ;
#684=EDGE_CURVE ( 'NONE', #10458, #6378, #13728, .T. ) ;
#687=CARTESIAN_POINT ( 'NONE',  ( 3.999999999999997780, -28.14205403674597861, -13.39922821167334810 ) ) ;
#689=CARTESIAN_POINT ( 'NONE',  ( 1.999999999999994449, -25.50649545827347353, -6.106093719671341624 ) ) ;
#690=ORIENTED_EDGE ( 'NONE', *, *, #8744, .T. ) ;
#691=EDGE_LOOP ( 'NONE', ( #11697, #16402, #8918, #16963 ) ) ;
#693=CARTESIAN_POINT ( 'NONE',  ( 4.000000000000003553, -18.84129845210892640, -6.653000668470220980 ) ) ;
#695=ORIENTED_EDGE ( 'NONE', *, *, #6775, .F. ) ;
#697=CARTESIAN_POINT ( 'NONE',  ( 4.243569643750003451, -23.00104207391549593, -12.83890243507441120 ) ) ;
#700=CARTESIAN_POINT ( 'NONE',  ( -0.5181399714674771451, -9.999999999997587707, -3.173488174254735839 ) ) ;
#701=CIRCLE ( 'NONE', #17888, 2.000000000000001776 ) ;
#702=CARTESIAN_POINT ( 'NONE',  ( -4.243569643750000786, -25.19081343183707844, -11.69472992346973861 ) ) ;
#703=CARTESIAN_POINT ( 'NONE',  ( 2.121784821874994176, -27.30860090601781209, -8.312008715962296179 ) ) ;
#704=CARTESIAN_POINT ( 'NONE',  ( -6.938893903907228378E-15, 6.938893903907228378E-15, -4.999999999999997335 ) ) ;
#705=CARTESIAN_POINT ( 'NONE',  ( -4.000000000000004441, -22.04405353722830085, -3.174373145209581804 ) ) ;
#707=CARTESIAN_POINT ( 'NONE',  ( -2.121784821875005722, -26.31918155331226217, -6.898971439563784003 ) ) ;
#710=CARTESIAN_POINT ( 'NONE',  ( -3.999999999999997335, -17.78735175101882859, -5.147808788095962207 ) ) ;
#712=EDGE_LOOP ( 'NONE', ( #2767, #16521, #3729, #8436, #3326, #6869 ) ) ;
#714=CARTESIAN_POINT ( 'NONE',  ( 4.000000000000000888, -23.91639828767208442, -9.874676475568506362 ) ) ;
#715=ADVANCED_FACE ( 'NONE', ( #15445, #17962, #11152, #8375, #10887, #18056 ), #6533, .F. ) ;
#717=CARTESIAN_POINT ( 'NONE',  ( 9.000000000000005329, -12.99999999999999822, -3.713574246709343996 ) ) ;
#718=EDGE_CURVE ( 'NONE', #4345, #7195, #15626, .T. ) ;
#720=CARTESIAN_POINT ( 'NONE',  ( 2.121784821874994176, -25.53409880605677884, -5.777757078943218438 ) ) ;
#726=EDGE_CURVE ( 'NONE', #17169, #13482, #4570, .T. ) ;
#727=CARTESIAN_POINT ( 'NONE',  ( 3.999999999999996447, -23.44214610012902966, -5.171056252157234745 ) ) ;
#731=CARTESIAN_POINT ( 'NONE',  ( 7.143010269575600368, -13.70175065102395706, 0.6871907070005838225 ) ) ;
#733=CARTESIAN_POINT ( 'NONE',  ( 2.121784821875004390, -17.10424616687832966, -6.553150170094818705 ) ) ;
#737=CARTESIAN_POINT ( 'NONE',  ( 2.000000000000004441, -20.26142594620695192, -10.69431187202529010 ) ) ;
#740=CARTESIAN_POINT ( 'NONE',  ( -4.000000000000000888, -21.39983167247694240, -6.280646880243780039 ) ) ;
#748=CARTESIAN_POINT ( 'NONE',  ( -5.279047395330986450E-15, -25.89313373868122881, -4.645111455626608432 ) ) ;
#749=ORIENTED_EDGE ( 'NONE', *, *, #8614, .F. ) ;
#750=LINE ( 'NONE', #16234, #7968 ) ;
#753=CARTESIAN_POINT ( 'NONE',  ( -2.121784821874996396, -16.77085486324927999, -6.077018044351843784 ) ) ;
#754=CARTESIAN_POINT ( 'NONE',  ( 2.121784821875004390, -21.23399650860583066, -12.45104488897558248 ) ) ;
#755=EDGE_CURVE ( 'NONE', #12418, #4334, #3095, .T. ) ;
#756=CARTESIAN_POINT ( 'NONE',  ( 3.999999999999993339, 7.428752623566170548E-15, -30.00000000000000000 ) ) ;
#758=CARTESIAN_POINT ( 'NONE',  ( -2.978814741686234946, -10.00000000000083844, 22.09987478886784018 ) ) ;
#761=CARTESIAN_POINT ( 'NONE',  ( 4.243569643749996345, -28.38075870064580286, -11.97895378909399078 ) ) ;
#762=ORIENTED_EDGE ( 'NONE', *, *, #13111, .F. ) ;
#765=CARTESIAN_POINT ( 'NONE',  ( 4.243569643750003451, -19.64561992126190049, -8.046862975983790633 ) ) ;
#768=CARTESIAN_POINT ( 'NONE',  ( 4.243569643750003451, -23.80763393753414903, -13.99083499735581171 ) ) ;
#769=CARTESIAN_POINT ( 'NONE',  ( 3.999999999999996447, -27.83000583821450036, -11.43756939096804714 ) ) ;
#770=CARTESIAN_POINT ( 'NONE',  ( 4.243569643750000786, -21.19011778828857118, -5.981144414553994260 ) ) ;
#773=CARTESIAN_POINT ( 'NONE',  ( 4.000000000000000888, -26.94918369417327142, -14.20594290873980192 ) ) ;
#774=FACE_OUTER_BOUND ( 'NONE', #8330, .T. ) ;
#778=EDGE_CURVE ( 'NONE', #16888, #7294, #3002, .T. ) ;
#780=CARTESIAN_POINT ( 'NONE',  ( 6.428571428571432378, -14.26578344203647752, -2.827263138854379410 ) ) ;
#781=ORIENTED_EDGE ( 'NONE', *, *, #883, .T. ) ;
#783=CARTESIAN_POINT ( 'NONE',  ( -2.121784821874996396, -21.93304279040865623, -13.44938644295279850 ) ) ;
#787=CARTESIAN_POINT ( 'NONE',  ( 5.562324373799151900, -10.00000000000000000, -9.830817939999416666 ) ) ;
#788=CARTESIAN_POINT ( 'NONE',  ( -2.121784821874996396, -22.73963465402730577, -14.60131900523419901 ) ) ;
#792=CARTESIAN_POINT ( 'NONE',  ( -1.071796769724496334, -29.52751773206367147, -10.91439834318392244 ) ) ;
#794=AXIS2_PLACEMENT_3D ( 'NONE', #18164, #18343, #14049 ) ;
#795=CARTESIAN_POINT ( 'NONE',  ( 4.243569643750000786, -23.73894807732350998, -9.621251311363216985 ) ) ;
#796=ORIENTED_EDGE ( 'NONE', *, *, #7337, .T. ) ;
#803=CARTESIAN_POINT ( 'NONE',  ( -2.000000000000005773, -22.90389237762567021, -2.389191317703265316 ) ) ;
#807=CARTESIAN_POINT ( 'NONE',  ( -4.243569643749998122, -20.10806592306992613, -8.707304311691796528 ) ) ;
#810=ORIENTED_EDGE ( 'NONE', *, *, #506, .F. ) ;
#813=EDGE_CURVE ( 'NONE', #18256, #8328, #1525, .T. ) ;
#814=CARTESIAN_POINT ( 'NONE',  ( -2.072127310227394492, -24.23032511484031915, -16.43161913306204980 ) ) ;
#815=CARTESIAN_POINT ( 'NONE',  ( 7.710291887657668930, -10.24552755907163970, 9.424636009669162817 ) ) ;
#816=CARTESIAN_POINT ( 'NONE',  ( -2.000000000000005773, -24.51707610556791650, -4.693056443272829448 ) ) ;
#817=CARTESIAN_POINT ( 'NONE',  ( 2.121784821874994176, -23.21111423883506220, -2.460191299572788814 ) ) ;
#819=ORIENTED_EDGE ( 'NONE', *, *, #9426, .F. ) ;
#821=CARTESIAN_POINT ( 'NONE',  ( -4.000000000000004441, -24.36703810445001750, -6.491938924580010983 ) ) ;
#825=CIRCLE ( 'NONE', #3186, 2.000000000000001776 ) ;
#826=ORIENTED_EDGE ( 'NONE', *, *, #2587, .F. ) ;
#834=CARTESIAN_POINT ( 'NONE',  ( -5.279047395330986450E-15, -24.60258675689138386, -2.802019355976369752 ) ) ;
#836=TOROIDAL_SURFACE ( 'NONE', #2897, 4.400000000000002132, 0.4000000000000000222 ) ;
#840=ADVANCED_FACE ( 'NONE', ( #315 ), #18327, .F. ) ;
#841=DIRECTION ( 'NONE',  ( -0.3258630558627232943, 0.000000000000000000, 0.9454169814551713902 ) ) ;
#843=CARTESIAN_POINT ( 'NONE',  ( 4.243569643750003451, -18.61318233583002879, -6.572389296263599689 ) ) ;
#845=CARTESIAN_POINT ( 'NONE',  ( 4.243569643750003451, -22.77519635210228088, -12.51636131763562076 ) ) ;
#846=CARTESIAN_POINT ( 'NONE',  ( 4.299564228933482956E-15, -23.15635672500629738, -15.76301181529063555 ) ) ;
#848=CARTESIAN_POINT ( 'NONE',  ( 6.903430137609765538, -10.00000000000000178, 15.77881270003217828 ) ) ;
#850=FACE_OUTER_BOUND ( 'NONE', #998, .T. ) ;
#851=VERTEX_POINT ( 'NONE', #6424 ) ;
#853=AXIS2_PLACEMENT_3D ( 'NONE', #2448, #17847, #13464 ) ;
#854=CARTESIAN_POINT ( 'NONE',  ( -4.243569643750000786, -20.51258062284889760, -5.013521062237622949 ) ) ;
#857=CARTESIAN_POINT ( 'NONE',  ( 2.000000000000004441, -22.00366437091829397, -13.18248620554634698 ) ) ;
#858=ORIENTED_EDGE ( 'NONE', *, *, #7727, .T. ) ;
#859=CARTESIAN_POINT ( 'NONE',  ( -4.243569643749997233, -19.84995652671195998, -8.338685891761748792 ) ) ;
#865=CARTESIAN_POINT ( 'NONE',  ( 1.071796769724485232, -25.95546013140888064, -5.812971400840699410 ) ) ;
#869=CARTESIAN_POINT ( 'NONE',  ( 3.579096709490575479E-14, -24.93454924669583406, -4.354959555776423130 ) ) ;
#874=SURFACE_SIDE_STYLE ('',( #12074 ) ) ;
#875=CARTESIAN_POINT ( 'NONE',  ( -4.243569643749997233, -22.65689621210486138, -12.34741120850101836 ) ) ;
#880=CARTESIAN_POINT ( 'NONE',  ( -1.006530391518317247, -10.00000000000122213, -4.211315095027532429 ) ) ;
#881=CARTESIAN_POINT ( 'NONE',  ( -4.243569643750000786, -25.70703222455301784, -12.43196676332983408 ) ) ;
#883=EDGE_CURVE ( 'NONE', #15966, #8825, #1892, .T. ) ;
#886=CARTESIAN_POINT ( 'NONE',  ( -4.000000000000000888, -20.17381204048153265, -4.529709386582819519 ) ) ;
#887=DIRECTION ( 'NONE',  ( -0.000000000000000000, 1.000000000000000000, -0.000000000000000000 ) ) ;
#888=CARTESIAN_POINT ( 'NONE',  ( -4.243569643749997233, -20.85013043759908413, -9.767082268990684213 ) ) ;
#890=ADVANCED_FACE ( 'NONE', ( #11889 ), #10502, .F. ) ;
#892=FACE_OUTER_BOUND ( 'NONE', #14880, .T. ) ;
#899=DIRECTION ( 'NONE',  ( 0.000000000000000000, 0.8191520442889952403, -0.5735764363510413855 ) ) ;
#901=CARTESIAN_POINT ( 'NONE',  ( 4.730628863548789710E-15, -19.17657787239343747, -11.64849162045545405 ) ) ;
#911=CARTESIAN_POINT ( 'NONE',  ( 4.730628863548789710E-15, -23.01595514321822122, -17.13169061691491279 ) ) ;
#913=CARTESIAN_POINT ( 'NONE',  ( 2.000000000000004441, -20.51953534256492162, -11.06293029195533784 ) ) ;
#916=ORIENTED_EDGE ( 'NONE', *, *, #8515, .T. ) ;
#918=CARTESIAN_POINT ( 'NONE',  ( -5.577813053751546416E-15, -28.80619019206536535, -9.884235854727139170 ) ) ;
#925=CARTESIAN_POINT ( 'NONE',  ( 4.000000000000003553, -18.58318905575096025, -6.284382248540171467 ) ) ;
#926=ORIENTED_EDGE ( 'NONE', *, *, #4785, .F. ) ;
#930=( BOUNDED_CURVE ( )  B_SPLINE_CURVE ( 2, ( #9246, #10541, #11939, #16216, #3511, #3596, #2401, #14834, #16403 ),
 .UNSPECIFIED., .F., .T. ) 
 B_SPLINE_CURVE_WITH_KNOTS ( ( 3, 2, 2, 2, 3 ),
 ( 0.5086206896551724865, 0.5114942528735632044, 0.5172413793103448620, 0.5229885057471264087, 0.5258620689655172376 ),
 .UNSPECIFIED. ) 
 CURVE ( )  GEOMETRIC_REPRESENTATION_ITEM ( )  RATIONAL_B_SPLINE_CURVE ( ( 0.9330127018922194093, 0.9330127018922206306, 1.000000000000000000, 0.8660254037844387076, 1.000000000000000000, 0.8660254037844387076, 1.000000000000000000, 0.9330127018922194093, 0.9330127018922194093 ) ) 
 REPRESENTATION_ITEM ( '' )  );
#931=LINE ( 'NONE', #5180, #9055 ) ;
#932=CARTESIAN_POINT ( 'NONE',  ( 4.243569643750000786, -20.64163532102788778, -5.197830272202643265 ) ) ;
#933=CARTESIAN_POINT ( 'NONE',  ( 4.243569643749996345, -26.57399292614002562, -9.398624849583658403 ) ) ;
#934=CARTESIAN_POINT ( 'NONE',  ( 2.659568448039375088, -29.44477373260542663, -12.53330527340647471 ) ) ;
#937=CARTESIAN_POINT ( 'NONE',  ( -3.772879157352762913, -10.00000000000000178, -12.59063537424807677 ) ) ;
#938=CARTESIAN_POINT ( 'NONE',  ( -2.000000000000005773, -25.48498634120535655, -6.075375517003743120 ) ) ;
#939=CARTESIAN_POINT ( 'NONE',  ( -4.000000000000004441, -24.62514750080798720, -6.860557344510057831 ) ) ;
#943=CARTESIAN_POINT ( 'NONE',  ( 2.000000000000004441, -24.13306689157648321, -16.22358817097600436 ) ) ;
#947=EDGE_CURVE ( 'NONE', #14660, #16355, #5656, .T. ) ;
#948=CARTESIAN_POINT ( 'NONE',  ( -4.000000000000000888, -24.49714442877256459, -10.70406791940435198 ) ) ;
#949=ORIENTED_EDGE ( 'NONE', *, *, #17401, .F. ) ;
#950=EDGE_CURVE ( 'NONE', #1446, #1376, #14215, .T. ) ;
#951=CARTESIAN_POINT ( 'NONE',  ( 4.243569643749996345, -21.92802379169658877, -2.763493290842798267 ) ) ;
#955=CARTESIAN_POINT ( 'NONE',  ( 1.533898589781675205E-14, -27.45111586048108521, -7.948989149087622330 ) ) ;
#961=EDGE_LOOP ( 'NONE', ( #16910, #10250, #7255 ) ) ;
#962=ORIENTED_EDGE ( 'NONE', *, *, #14291, .T. ) ;
#967=CARTESIAN_POINT ( 'NONE',  ( 7.406012110500714840, -12.49260087798120367, 8.584195667863683710 ) ) ;
#971=CARTESIAN_POINT ( 'NONE',  ( 4.243569643750003451, -22.74293267755752623, -12.47028401514436169 ) ) ;
#975=CYLINDRICAL_SURFACE ( 'NONE', #13734, 4.000000000000000000 ) ;
#977=CARTESIAN_POINT ( 'NONE',  ( 4.243569643750000786, -26.09419631908997772, -12.98489439322490213 ) ) ;
#983=CARTESIAN_POINT ( 'NONE',  ( 4.243569643750003451, -19.38751052490393434, -7.678244556053742897 ) ) ;
#985=VERTEX_POINT ( 'NONE', #501 ) ;
#986=CARTESIAN_POINT ( 'NONE',  ( -1.071796769724487675, -23.59652146720896582, -16.39163221450554531 ) ) ;
#988=CARTESIAN_POINT ( 'NONE',  ( 3.064181913176683203, -21.66367673124435100, -2.174801284911689336 ) ) ;
#994=FACE_OUTER_BOUND ( 'NONE', #4572, .T. ) ;
#995=ORIENTED_EDGE ( 'NONE', *, *, #17161, .F. ) ;
#996=CARTESIAN_POINT ( 'NONE',  ( -2.121784821874996396, -18.09366551958387248, -7.966187446493337987 ) ) ;
#998=EDGE_LOOP ( 'NONE', ( #10590, #3435, #5889, #4242 ) ) ;
#1000=CARTESIAN_POINT ( 'NONE',  ( 4.243569643750003451, -25.06591724477924288, -15.78784979451479309 ) ) ;
#1001=CARTESIAN_POINT ( 'NONE',  ( 3.220835151890553583, -25.02781588011482938, -15.95816000315516270 ) ) ;
#1003=CARTESIAN_POINT ( 'NONE',  ( 10.00272540370463226, -9.915619283365160186, 6.515181925709914168 ) ) ;
#1005=CARTESIAN_POINT ( 'NONE',  ( 2.121784821875004390, -23.78282679764076590, -16.09115178578480254 ) ) ;
#1008=CARTESIAN_POINT ( 'NONE',  ( -4.000000000000004441, -24.10892870809205135, -6.123320504649964136 ) ) ;
#1012=CARTESIAN_POINT ( 'NONE',  ( -1.071796769724486786, -17.91811474733365372, -8.282026976044495115 ) ) ;
#1019=EDGE_CURVE ( 'NONE', #5846, #2315, #17393, .T. ) ;
#1020=CARTESIAN_POINT ( 'NONE',  ( -4.000000000000004441, -22.49574498014980151, -3.819455379080400004 ) ) ;
#1024=DIRECTION ( 'NONE',  ( 0.000000000000000000, 0.000000000000000000, 1.000000000000000000 ) ) ;
#1025=CARTESIAN_POINT ( 'NONE',  ( 4.730628863548789710E-15, -16.30511083791103744, -7.547611698733672547 ) ) ;
#1026=CARTESIAN_POINT ( 'NONE',  ( -4.243569643750005227, -24.33704482437095251, -6.203931876856584537 ) ) ;
#1035=CARTESIAN_POINT ( 'NONE',  ( -1.999999999999996225, -24.09004865885014723, -16.16215176765433270 ) ) ;
#1039=CARTESIAN_POINT ( 'NONE',  ( 4.000000000000003553, -23.22915819019439709, -12.91951380728103160 ) ) ;
#1040=( BOUNDED_CURVE ( )  B_SPLINE_CURVE ( 2, ( #17747, #2068, #2251, #9184, #3626, #939, #15037, #13627, #3540 ),
 .UNSPECIFIED., .F., .T. ) 
 B_SPLINE_CURVE_WITH_KNOTS ( ( 3, 2, 2, 2, 3 ),
 ( 0.5603448275862069616, 0.5632183908045976795, 0.5689655172413793371, 0.5747126436781608838, 0.5775862068965517127 ),
 .UNSPECIFIED. ) 
 CURVE ( )  GEOMETRIC_REPRESENTATION_ITEM ( )  RATIONAL_B_SPLINE_CURVE ( ( 0.9330127018922194093, 0.9330127018922206306, 1.000000000000000000, 0.8660254037844387076, 1.000000000000000000, 0.8660254037844387076, 1.000000000000000000, 0.9330127018922194093, 0.9330127018922194093 ) ) 
 REPRESENTATION_ITEM ( '' )  );
#1042=CARTESIAN_POINT ( 'NONE',  ( -4.243569643749997233, -18.30130014856414533, -6.126975372181463264 ) ) ;
#1044=CARTESIAN_POINT ( 'NONE',  ( 8.500000000000019540, 0.000000000000000000, -20.49999999999998934 ) ) ;
#1045=CARTESIAN_POINT ( 'NONE',  ( -5.330712181944246111E-15, -28.33358195679832292, -7.640088304762238103 ) ) ;
#1046=CARTESIAN_POINT ( 'NONE',  ( 1.999999999999994449, -29.05549965749059638, -11.17459699270273354 ) ) ;
#1047=EDGE_CURVE ( 'NONE', #3748, #10497, #9446, .T. ) ;
#1048=ADVANCED_FACE ( 'NONE', ( #15059 ), #13745, .F. ) ;
#1049=CARTESIAN_POINT ( 'NONE',  ( 3.999999999999996447, -23.24856405356550226, -4.894592438216466057 ) ) ;
#1051=CARTESIAN_POINT ( 'NONE',  ( 0.000000000000000000, 5.977523610840987267, 32.81826849749789687 ) ) ;
#1052=VERTEX_POINT ( 'NONE', #12255 ) ;
#1057=CARTESIAN_POINT ( 'NONE',  ( 3.999999999999996447, -26.02324006370871956, -8.857240451457712993 ) ) ;
#1060=CARTESIAN_POINT ( 'NONE',  ( 2.121784821875004390, -21.45984223041904926, -12.77358600641437469 ) ) ;
#1064=DIRECTION ( 'NONE',  ( -0.000000000000000000, -0.5735764363510414965, -0.8191520442889950182 ) ) ;
#1066=CARTESIAN_POINT ( 'NONE',  ( -2.121784821875005722, -27.38388281328888141, -8.419522421775232246 ) ) ;
#1069=CARTESIAN_POINT ( 'NONE',  ( -1.071796769724505882, -17.46642330441216018, -7.636944742173667144 ) ) ;
#1072=CARTESIAN_POINT ( 'NONE',  ( 2.121784821875004390, -19.39496705955529876, -9.824638646973991030 ) ) ;
#1084=CARTESIAN_POINT ( 'NONE',  ( -5.330712181944246111E-15, -25.52664227140541087, -3.631362988022969862 ) ) ;
#1087=DIRECTION ( 'NONE',  ( -0.000000000000000000, -0.5735764363510414965, -0.8191520442889950182 ) ) ;
#1089=CARTESIAN_POINT ( 'NONE',  ( 4.243569643749997233, -28.60660442245902502, -12.30149490653278121 ) ) ;
#1090=FACE_OUTER_BOUND ( 'NONE', #15810, .T. ) ;
#1092=CARTESIAN_POINT ( 'NONE',  ( -4.243569643750005227, -28.43453149155370241, -12.05574929324608924 ) ) ;
#1094=FACE_OUTER_BOUND ( 'NONE', #5867, .T. ) ;
#1095=CARTESIAN_POINT ( 'NONE',  ( 1.999999999999994449, -25.24838606191550028, -5.737475299741293888 ) ) ;
#1097=ORIENTED_EDGE ( 'NONE', *, *, #8515, .F. ) ;
#1098=CARTESIAN_POINT ( 'NONE',  ( 1.071796769724495224, -22.90977402936716345, -15.41085523001650515 ) ) ;
#1101=CARTESIAN_POINT ( 'NONE',  ( -2.000000000000005773, -23.16200177398363991, -2.757809737633313940 ) ) ;
#1105=CARTESIAN_POINT ( 'NONE',  ( 4.243569643749997233, -27.34832111521393117, -10.50448010937379983 ) ) ;
#1107=CARTESIAN_POINT ( 'NONE',  ( 4.000000000000000888, -21.27077697429796288, -6.096337670278750842 ) ) ;
#1110=EDGE_CURVE ( 'NONE', #3352, #16039, #15735, .T. ) ;
#1116=CARTESIAN_POINT ( 'NONE',  ( -2.121784821875005722, -26.09333583149904001, -6.576430322124992678 ) ) ;
#1117=EDGE_CURVE ( 'NONE', #15867, #2086, #9221, .T. ) ;
#1120=ORIENTED_EDGE ( 'NONE', *, *, #4909, .T. ) ;
#1121=CARTESIAN_POINT ( 'NONE',  ( 4.000000000000000888, -24.17450768403005767, -10.24329489549855410 ) ) ;
#1122=DIRECTION ( 'NONE',  ( -1.000000000000000000, -0.000000000000000000, 8.673617379884034239E-17 ) ) ;
#1124=ADVANCED_FACE ( 'NONE', ( #3731 ), #12345, .F. ) ;
#1128=CARTESIAN_POINT ( 'NONE',  ( 4.243569643750000786, -20.12541652831194838, -4.460593432342547793 ) ) ;
#1131=VECTOR ( 'NONE', #12180, 1000.000000000000000 ) ;
#1132=CARTESIAN_POINT ( 'NONE',  ( 4.000000000000000888, -24.36808973059358863, -10.51975870943932456 ) ) ;
#1133=ORIENTED_EDGE ( 'NONE', *, *, #8853, .T. ) ;
#1134=CARTESIAN_POINT ( 'NONE',  ( 4.243569643749996345, -22.44424258441252817, -3.500730130702893739 ) ) ;
#1137=CARTESIAN_POINT ( 'NONE',  ( 4.243569643749997233, -26.02551045887933867, -8.615310707232305631 ) ) ;
#1139=CARTESIAN_POINT ( 'NONE',  ( 1.999999999999994449, -24.21594847648362858, -4.263001620021102944 ) ) ;
#1142=EDGE_LOOP ( 'NONE', ( #18109, #926 ) ) ;
#1145=CARTESIAN_POINT ( 'NONE',  ( -5.000000000000001776, 0.000000000000000000, -4.999999999999999112 ) ) ;
#1146=CARTESIAN_POINT ( 'NONE',  ( 1.743066579297358403E-15, -23.41446612136426708, -16.13163023522068684 ) ) ;
#1149=CARTESIAN_POINT ( 'NONE',  ( 4.243569643749996345, -26.02551045887933867, -8.615310707232305631 ) ) ;
#1151=( BOUNDED_CURVE ( )  B_SPLINE_CURVE ( 2, ( #12526, #8775, #13048, #4610, #15508, #1758, #16816, #5484, #4088 ),
 .UNSPECIFIED., .F., .F. ) 
 B_SPLINE_CURVE_WITH_KNOTS ( ( 3, 2, 2, 2, 3 ),
 ( 0.8189655172413793371, 0.8218390804597701660, 0.8275862068965517127, 0.8333333333333333703, 0.8362068965517241992 ),
 .UNSPECIFIED. ) 
 CURVE ( )  GEOMETRIC_REPRESENTATION_ITEM ( )  RATIONAL_B_SPLINE_CURVE ( ( 0.9330127018922194093, 0.9330127018922194093, 1.000000000000000000, 0.8660254037844387076, 1.000000000000000000, 0.8660254037844387076, 1.000000000000000000, 0.9330127018922180770, 0.9330127018922194093 ) ) 
 REPRESENTATION_ITEM ( '' )  );
#1155=CARTESIAN_POINT ( 'NONE',  ( 4.243569643749996345, -26.31588352978205592, -9.030006429653610667 ) ) ;
#1158=CARTESIAN_POINT ( 'NONE',  ( -0.6435590302262776952, -15.45066141473203203, -10.82404826198590797 ) ) ;
#1159=CARTESIAN_POINT ( 'NONE',  ( -6.158835246850665095E-15, -22.31750118613795664, -14.56500194951122218 ) ) ;
#1163=CARTESIAN_POINT ( 'NONE',  ( 4.730628863548789710E-15, -17.59565781970087883, -9.390703798383910339 ) ) ;
#1164=CARTESIAN_POINT ( 'NONE',  ( -4.000000000000000888, -26.82012899599428124, -14.02163369877478161 ) ) ;
#1170=CARTESIAN_POINT ( 'NONE',  ( -1.071796769724505882, -16.88567716190178913, -6.807553296324296177 ) ) ;
#1174=CARTESIAN_POINT ( 'NONE',  ( -4.243569643750000786, -20.80295369375161130, -5.428216784658927985 ) ) ;
#1176=EDGE_CURVE ( 'NONE', #10810, #317, #16342, .T. ) ;
#1180=CARTESIAN_POINT ( 'NONE',  ( 9.184850993605147944E-16, -10.54254386713301628, 22.30101802474215589 ) ) ;
#1185=CARTESIAN_POINT ( 'NONE',  ( 4.000000000000003553, -24.51970517198423849, -14.76260590693127028 ) ) ;
#1187=CARTESIAN_POINT ( 'NONE',  ( 4.243569643750000786, -26.06193264454523018, -12.93881709073364661 ) ) ;
#1188=ORIENTED_EDGE ( 'NONE', *, *, #10509, .T. ) ;
#1190=CARTESIAN_POINT ( 'NONE',  ( -1.999999999999996225, -18.92786073169077454, -8.789783369053376205 ) ) ;
#1193=DIRECTION ( 'NONE',  ( -0.000000000000000000, -0.000000000000000000, -1.000000000000000000 ) ) ;
#1198=AXIS2_PLACEMENT_3D ( 'NONE', #6842, #12492, #1297 ) ;
#1201=CARTESIAN_POINT ( 'NONE',  ( -2.121784821875005722, -28.67442979507872636, -10.26261452142547093 ) ) ;
#1203=CARTESIAN_POINT ( 'NONE',  ( -1.999999999999996225, -17.31467700374852470, -6.485918243483816958 ) ) ;
#1206=CARTESIAN_POINT ( 'NONE',  ( 9.184850993605147944E-16, -8.516114662390016576, 25.19505885429991565 ) ) ;
#1210=CARTESIAN_POINT ( 'NONE',  ( -4.243569643750000786, -22.60971946825739209, -8.008545724169261248 ) ) ;
#1211=ORIENTED_EDGE ( 'NONE', *, *, #1576, .T. ) ;
#1214=CARTESIAN_POINT ( 'NONE',  ( 4.713407268011036227E-15, -20.32647910872069730, -12.80037636994084416 ) ) ;
#1220=CARTESIAN_POINT ( 'NONE',  ( 2.121784821874994176, -22.92074116793234140, -2.045495577151484223 ) ) ;
#1225=CARTESIAN_POINT ( 'NONE',  ( -3.999999999999997335, -23.40123112109970194, -13.16525942056773246 ) ) ;
#1226=ORIENTED_EDGE ( 'NONE', *, *, #6652, .T. ) ;
#1228=CARTESIAN_POINT ( 'NONE',  ( -4.000000000000000888, -25.59410936399887504, -12.27069620511382197 ) ) ;
#1231=CARTESIAN_POINT ( 'NONE',  ( -1.071796769724496334, -21.07995485342371822, -12.79760262119433634 ) ) ;
#1232=CARTESIAN_POINT ( 'NONE',  ( -4.243569643750000786, -22.31934639735467840, -7.593850001747957990 ) ) ;
#1237=ORIENTED_EDGE ( 'NONE', *, *, #11288, .F. ) ;
#1241=CARTESIAN_POINT ( 'NONE',  ( 5.810221930991194676E-16, -23.67257551772224033, -16.50024865515073458 ) ) ;
#1244=CARTESIAN_POINT ( 'NONE',  ( -4.243569643750005227, -26.62776571704792161, -9.475420353735755086 ) ) ;
#1247=AXIS2_PLACEMENT_3D ( 'NONE', #6874, #3823, #12532 ) ;
#1251=CARTESIAN_POINT ( 'NONE',  ( 4.243569643750003451, -22.00086816302836823, -11.41050605784547578 ) ) ;
#1253=CARTESIAN_POINT ( 'NONE',  ( 0.2621597573826395799, -10.00000000000313527, -3.075850967169316164 ) ) ;
#1257=( BOUNDED_CURVE ( )  B_SPLINE_CURVE ( 2, ( #7907, #5128, #10784, #13475, #10511, #6434, #13296, #13562, #10602 ),
 .UNSPECIFIED., .F., .T. ) 
 B_SPLINE_CURVE_WITH_KNOTS ( ( 3, 2, 2, 2, 3 ),
 ( 0.4224137931034482873, 0.4252873563218390607, 0.4310344827586206629, 0.4367816091954023205, 0.4396551724137931494 ),
 .UNSPECIFIED. ) 
 CURVE ( )  GEOMETRIC_REPRESENTATION_ITEM ( )  RATIONAL_B_SPLINE_CURVE ( ( 0.9330127018922194093, 0.9330127018922200755, 1.000000000000000000, 0.8660254037844387076, 1.000000000000000000, 0.8660254037844387076, 1.000000000000000000, 0.9330127018922187432, 0.9330127018922194093 ) ) 
 REPRESENTATION_ITEM ( '' )  );
#1258=CARTESIAN_POINT ( 'NONE',  ( 2.121784821874994176, -25.24372573515406515, -5.363061356521914291 ) ) ;
#1259=CARTESIAN_POINT ( 'NONE',  ( -2.000000000000005773, -24.77518550192588620, -5.061674863202877184 ) ) ;
#1262=CARTESIAN_POINT ( 'NONE',  ( 2.000000000000004441, -17.61580463283282683, -6.915973066735536356 ) ) ;
#1268=CARTESIAN_POINT ( 'NONE',  ( -4.243569643749998122, -19.07562833763805443, -7.232830631971606472 ) ) ;
#1272=CARTESIAN_POINT ( 'NONE',  ( -4.243569643750000786, -26.96531553179811169, -14.22898156048881724 ) ) ;
#1273=DIRECTION ( 'NONE',  ( -0.000000000000000000, 1.000000000000000000, -0.000000000000000000 ) ) ;
#1276=CARTESIAN_POINT ( 'NONE',  ( 2.121784821875004390, -22.49227981585092095, -14.24805968613456564 ) ) ;
#1281=CARTESIAN_POINT ( 'NONE',  ( 4.000000000000000888, -21.59341372045036778, -6.557110696198077626 ) ) ;
#1284=ADVANCED_FACE ( 'NONE', ( #18 ), #3076, .F. ) ;
#1286=CARTESIAN_POINT ( 'NONE',  ( 4.000000000000003553, -24.32612312542070754, -14.48614209299050160 ) ) ;
#1289=DIRECTION ( 'NONE',  ( -0.000000000000000000, 1.000000000000000000, -0.000000000000000000 ) ) ;
#1292=CARTESIAN_POINT ( 'NONE',  ( 4.243569643750000786, -25.06175873365810247, -11.51042071350471119 ) ) ;
#1295=ORIENTED_EDGE ( 'NONE', *, *, #5587, .F. ) ;
#1297=DIRECTION ( 'NONE',  ( 0.000000000000000000, 0.000000000000000000, -1.000000000000000000 ) ) ;
#1298=AXIS2_PLACEMENT_3D ( 'NONE', #17832, #10842, #2608 ) ;
#1299=CARTESIAN_POINT ( 'NONE',  ( -6.428571428571425272, -14.26578344203648285, -2.827263138854410496 ) ) ;
#1301=CARTESIAN_POINT ( 'NONE',  ( -4.243569643750000786, -22.86782886461536179, -8.377164144099308984 ) ) ;
#1304=ORIENTED_EDGE ( 'NONE', *, *, #755, .F. ) ;
#1305=CARTESIAN_POINT ( 'NONE',  ( 2.000000000000004441, -21.81008232435476657, -12.90602239160557829 ) ) ;
#1306=CARTESIAN_POINT ( 'NONE',  ( -7.056670106005028309, -10.00000000000000178, -9.351700598554243626 ) ) ;
#1307=VECTOR ( 'NONE', #10874, 1000.000000000000000 ) ;
#1312=CARTESIAN_POINT ( 'NONE',  ( 4.000000000000003553, -24.58423252177867369, -14.85476051292054578 ) ) ;
#1315=CARTESIAN_POINT ( 'NONE',  ( -4.000000000000000888, -23.72281623969865905, -9.598212659614208775 ) ) ;
#1316=ORIENTED_EDGE ( 'NONE', *, *, #9101, .F. ) ;
#1317=CARTESIAN_POINT ( 'NONE',  ( -4.243569643749997233, -17.78508135584820948, -5.389738532321366904 ) ) ;
#1320=CARTESIAN_POINT ( 'NONE',  ( 2.121784821874994176, -25.24372573515406515, -5.363061356521914291 ) ) ;
#1321=EDGE_CURVE ( 'NONE', #16039, #851, #11329, .T. ) ;
#1329=CARTESIAN_POINT ( 'NONE',  ( -4.000000000000000888, -21.91605046519287825, -7.017883720103874623 ) ) ;
#1330=CARTESIAN_POINT ( 'NONE',  ( -2.000000000000005773, -24.25896670920994680, -4.324438023342780824 ) ) ;
#1331=CARTESIAN_POINT ( 'NONE',  ( 4.299564228933482956E-15, -23.34993877156982833, -16.03947562923141135 ) ) ;
#1334=CARTESIAN_POINT ( 'NONE',  ( -4.243569643750000786, -22.57745579371264455, -7.962468421678005726 ) ) ;
#1337=CARTESIAN_POINT ( 'NONE',  ( -1.999999999999996225, -18.41164193897483869, -8.052546529193282510 ) ) ;
#1338=FACE_OUTER_BOUND ( 'NONE', #14567, .T. ) ;
#1339=CARTESIAN_POINT ( 'NONE',  ( 2.121784821875004390, -20.97588711224786095, -12.08242646904553474 ) ) ;
#1340=CARTESIAN_POINT ( 'NONE',  ( -2.237551826324946980, -10.00000000000000178, -12.18738508574780788 ) ) ;
#1343=CARTESIAN_POINT ( 'NONE',  ( -2.121784821875005722, -24.25430638244851167, -3.950024080123402559 ) ) ;
#1345=CARTESIAN_POINT ( 'NONE',  ( 0.000000000000000000, -27.20729309053124112, -14.57456132866985499 ) ) ;
#1348=EDGE_CURVE ( 'NONE', #13645, #17584, #18248, .T. ) ;
#1349=CARTESIAN_POINT ( 'NONE',  ( 4.000000000000000888, -23.40017949495614857, -9.137439635708412666 ) ) ;
#1354=CARTESIAN_POINT ( 'NONE',  ( 4.730628863548789710E-15, -17.62792149424562993, -9.436781100875167638 ) ) ;
#1357=CARTESIAN_POINT ( 'NONE',  ( 4.730628863548789710E-15, -23.01595514321822122, -17.13169061691491279 ) ) ;
#1358=( BOUNDED_SURFACE ( )  B_SPLINE_SURFACE ( 3, 2, ( 
 ( #8163, #7221, #8517 ),
 ( #15960, #11481, #15767 ),
 ( #3253, #11575, #17175 ),
 ( #11302, #14476, #5929 ),
 ( #285, #1494, #17270 ),
 ( #1587, #4352, #12791 ),
 ( #12877, #4629, #7408 ),
 ( #8892, #10278, #4542 ),
 ( #10184, #10002, #11671 ),
 ( #15861, #3158, #12970 ),
 ( #8795, #1872, #3066 ),
 ( #184, #8605, #14570 ),
 ( #1777, #2885, #12699 ),
 ( #5658, #4449, #15583 ) ),
 .UNSPECIFIED., .F., .F., .F. ) 
 B_SPLINE_SURFACE_WITH_KNOTS ( ( 4, 2, 2, 2, 2, 2, 4 ),
 ( 3, 3 ),
 ( -6.505213034913026604E-18, 0.002393516659216048982, 0.004787033318432104903, 0.007180549977648160824, 0.009574066636864216745, 0.01436109995529632859, 0.01914813327372844043 ),
 ( 0.000000000000000000, 1.000000000000000000 ),
 .UNSPECIFIED. ) 
 GEOMETRIC_REPRESENTATION_ITEM ( )  RATIONAL_B_SPLINE_SURFACE ( (
 ( 1.000000000000000000, 0.5376207706124455088, 1.000000000000000000),
 ( 1.000000000000000000, 0.5651826551449234959, 1.000000000000000000),
 ( 1.000000000000000000, 0.5897230234043094876, 1.000000000000000000),
 ( 1.000000000000000000, 0.6342462738084541085, 1.000000000000000000),
 ( 1.000000000000000000, 0.6542286737548208553, 1.000000000000000000),
 ( 1.000000000000000000, 0.6905470569484681853, 1.000000000000000000),
 ( 1.000000000000000000, 0.7068761916927887023, 1.000000000000000000),
 ( 1.000000000000000000, 0.7364394504874743896, 1.000000000000000000),
 ( 1.000000000000000000, 0.7497141571645004055, 1.000000000000000000),
 ( 1.000000000000000000, 0.7850493443857002873, 1.000000000000000000),
 ( 1.000000000000000000, 0.8026900302402008025, 1.000000000000000000),
 ( 1.000000000000000000, 0.8290821779924412160, 1.000000000000000000),
 ( 1.000000000000000000, 0.8377883503405891830, 1.000000000000000000),
 ( 1.000000000000000000, 0.8431867568967628124, 1.000000000000000000) ) ) 
 REPRESENTATION_ITEM ( '' )  SURFACE ( )  );
#1363=CARTESIAN_POINT ( 'NONE',  ( -5.330712181944245322E-15, -30.39845712766207342, -10.58903566420261910 ) ) ;
#1364=ORIENTED_EDGE ( 'NONE', *, *, #17337, .T. ) ;
#1366=CARTESIAN_POINT ( 'NONE',  ( -5.279047395330986450E-15, -25.69955169211769785, -4.368647641685837968 ) ) ;
#1373=CARTESIAN_POINT ( 'NONE',  ( 1.071796769724495224, -20.00604331963507221, -11.26389800479670633 ) ) ;
#1375=AXIS2_PLACEMENT_3D ( 'NONE', #18143, #16652, #18230 ) ;
#1376=VERTEX_POINT ( 'NONE', #4637 ) ;
#1377=CARTESIAN_POINT ( 'NONE',  ( 4.243569643750000786, -26.09419631908997772, -12.98489439322490213 ) ) ;
#1379=AXIS2_PLACEMENT_3D ( 'NONE', #16611, #13985, #13803 ) ;
#1387=CARTESIAN_POINT ( 'NONE',  ( 2.121784821874994176, -26.30842699513068439, -6.883612338733362535 ) ) ;
#1390=ORIENTED_EDGE ( 'NONE', *, *, #6483, .T. ) ;
#1391=VECTOR ( 'NONE', #1629, 1000.000000000000000 ) ;
#1392=CARTESIAN_POINT ( 'NONE',  ( -4.000000000000004441, -26.17380387895579830, -9.072267864090346023 ) ) ;
#1398=CARTESIAN_POINT ( 'NONE',  ( 3.999999999999996447, -28.41075198072487851, -12.26696083681741989 ) ) ;
#1401=CARTESIAN_POINT ( 'NONE',  ( -2.000000000000005773, -26.77553332299520150, -7.918467616653980024 ) ) ;
#1405=FACE_OUTER_BOUND ( 'NONE', #13425, .T. ) ;
#1406=ADVANCED_FACE ( 'NONE', ( #7601 ), #11772, .F. ) ;
#1409=CARTESIAN_POINT ( 'NONE',  ( 3.999999999999993339, 0.000000000000000000, 5.000000000000000888 ) ) ;
#1410=CARTESIAN_POINT ( 'NONE',  ( -2.121784821875005722, -25.80296276059631921, -6.161734599703687643 ) ) ;
#1412=CARTESIAN_POINT ( 'NONE',  ( 4.000000000000000888, -22.30321455972984168, -7.570811349998943562 ) ) ;
#1415=ORIENTED_EDGE ( 'NONE', *, *, #14028, .F. ) ;
#1420=CARTESIAN_POINT ( 'NONE',  ( 4.299564228933482956E-15, -17.73605940148895854, -8.022024996759636650 ) ) ;
#1426=CARTESIAN_POINT ( 'NONE',  ( 4.243569643750000786, -22.70651049189163828, -8.146777631643026041 ) ) ;
#1429=CARTESIAN_POINT ( 'NONE',  ( -1.071796769724505882, -17.98264209712809958, -8.374181582033761728 ) ) ;
#1431=CARTESIAN_POINT ( 'NONE',  ( 2.121784821874994176, -25.79220820241474854, -6.146375498873266174 ) ) ;
#1433=CARTESIAN_POINT ( 'NONE',  ( 2.599319604203554679, -24.48737926485759431, -15.99075565718284153 ) ) ;
#1434=EDGE_CURVE ( 'NONE', #7294, #8864, #1775, .T. ) ;
#1437=CARTESIAN_POINT ( 'NONE',  ( -5.330712181944245322E-15, -24.97815980414473103, -2.848048845671618423 ) ) ;
#1444=PLANE ( 'NONE',  #8387 ) ;
#1445=DIRECTION ( 'NONE',  ( 1.000000000000000000, 0.000000000000000000, 0.000000000000000000 ) ) ;
#1446=VERTEX_POINT ( 'NONE', #7416 ) ;
#1447=CARTESIAN_POINT ( 'NONE',  ( 4.243569643750000786, -20.15768020285669593, -4.506670734833804204 ) ) ;
#1451=CARTESIAN_POINT ( 'NONE',  ( 2.121784821875004390, -22.49227981585092095, -14.24805968613456564 ) ) ;
#1457=CARTESIAN_POINT ( 'NONE',  ( -2.121784821875005722, -27.35161913874413386, -8.373445119283974947 ) ) ;
#1458=VERTEX_POINT ( 'NONE', #15872 ) ;
#1460=CARTESIAN_POINT ( 'NONE',  ( 1.999999999999994449, -23.18351089105175333, -2.788527940300912444 ) ) ;
#1462=EDGE_LOOP ( 'NONE', ( #3760, #12477, #9504, #5010 ) ) ;
#1463=CARTESIAN_POINT ( 'NONE',  ( 3.276967058447619152, -25.10900663730464188, -15.57833582608148326 ) ) ;
#1469=CARTESIAN_POINT ( 'NONE',  ( 4.243569643749997233, -26.57399292614001851, -9.398624849583658403 ) ) ;
#1472=ORIENTED_EDGE ( 'NONE', *, *, #17613, .F. ) ;
#1474=FACE_OUTER_BOUND ( 'NONE', #8392, .T. ) ;
#1476=CARTESIAN_POINT ( 'NONE',  ( -4.243569643750005227, -23.82082603165501666, -5.466695036996486401 ) ) ;
#1477=ORIENTED_EDGE ( 'NONE', *, *, #3659, .F. ) ;
#1479=ORIENTED_EDGE ( 'NONE', *, *, #10509, .F. ) ;
#1480=EDGE_LOOP ( 'NONE', ( #17026, #9744, #18292, #16872 ) ) ;
#1486=CARTESIAN_POINT ( 'NONE',  ( -1.999999999999996225, -23.83193926249218109, -15.79353334772428497 ) ) ;
#1489=CARTESIAN_POINT ( 'NONE',  ( -1.999999999999996225, -20.92820855276008629, -11.64657612250448437 ) ) ;
#1490=ORIENTED_EDGE ( 'NONE', *, *, #1047, .F. ) ;
#1492=FACE_OUTER_BOUND ( 'NONE', #1480, .T. ) ;
#1494=CARTESIAN_POINT ( 'NONE',  ( -6.270298154903644949, -10.34439663368850937, 0.7558933527348972170 ) ) ;
#1495=CARTESIAN_POINT ( 'NONE',  ( 2.121784821875004390, -19.65307645591326846, -10.19325706690404054 ) ) ;
#1497=CARTESIAN_POINT ( 'NONE',  ( -1.071796769724496334, -23.13931017290888903, -1.791092450922006529 ) ) ;
#1502=CARTESIAN_POINT ( 'NONE',  ( -2.000000000000005773, -26.00120513392129240, -6.812612356863837704 ) ) ;
#1510=CARTESIAN_POINT ( 'NONE',  ( -2.121784821875005722, -25.54485336423835307, -5.793116179773641683 ) ) ;
#1515=CARTESIAN_POINT ( 'NONE',  ( 3.999999999999996447, -26.86209560257706030, -10.05525031723713347 ) ) ;
#1516=EDGE_CURVE ( 'NONE', #8485, #2986, #3660, .T. ) ;
#1517=CARTESIAN_POINT ( 'NONE',  ( 4.243569643749996345, -23.99289896256033572, -5.712440650283179266 ) ) ;
#1519=( BOUNDED_CURVE ( )  B_SPLINE_CURVE ( 3, ( #14527, #7181, #8944, #5886 ),
 .UNSPECIFIED., .F., .F. ) 
 B_SPLINE_CURVE_WITH_KNOTS ( ( 4, 4 ),
 ( 0.000000000000000000, 1.029696800837752058 ),
 .UNSPECIFIED. ) 
 CURVE ( )  GEOMETRIC_REPRESENTATION_ITEM ( )  RATIONAL_B_SPLINE_CURVE ( ( 1.000000000000000000, 0.9135782535825734962, 0.9135782535825734962, 1.000000000000000000 ) ) 
 REPRESENTATION_ITEM ( '' )  );
#1520=EDGE_CURVE ( 'NONE', #6047, #10458, #5547, .T. ) ;
#1521=CARTESIAN_POINT ( 'NONE',  ( -8.511038526056534437, -10.00000000000000178, -5.033916384140056266 ) ) ;
#1523=CARTESIAN_POINT ( 'NONE',  ( -14.99999999999999645, 10.00000000000000000, 30.00000000000000000 ) ) ;
#1524=CARTESIAN_POINT ( 'NONE',  ( 2.121784821875004390, -17.58820128504952152, -7.244309707463659542 ) ) ;
#1525=LINE ( 'NONE', #7342, #6209 ) ;
#1527=EDGE_LOOP ( 'NONE', ( #16504, #13644, #6239, #8457 ) ) ;
#1529=CARTESIAN_POINT ( 'NONE',  ( 2.121784821874994176, -29.63158547323952874, -11.62957449533272580 ) ) ;
#1535=CARTESIAN_POINT ( 'NONE',  ( 2.121784821874994176, -23.21111423883506220, -2.460191299572788814 ) ) ;
#1537=CARTESIAN_POINT ( 'NONE',  ( 4.243569643749996345, -28.89697749336173871, -12.71619062895408803 ) ) ;
#1539=CARTESIAN_POINT ( 'NONE',  ( 4.730628863548789710E-15, -21.98351755778634953, -15.65721693719472185 ) ) ;
#1542=CARTESIAN_POINT ( 'NONE',  ( -1.661723472263481630E-14, -21.34959095050052014, -13.18268287578030318 ) ) ;
#1543=DIRECTION ( 'NONE',  ( 0.000000000000000000, 0.000000000000000000, 1.000000000000000000 ) ) ;
#1544=CARTESIAN_POINT ( 'NONE',  ( -4.243569643750005227, -26.11154692433198576, -8.738183513875661390 ) ) ;
#1545=DIRECTION ( 'NONE',  ( -0.000000000000000000, -0.5735764363510414965, -0.8191520442889950182 ) ) ;
#1546=CARTESIAN_POINT ( 'NONE',  ( 4.000000000000003553, -18.38960700918742575, -6.007918434599401891 ) ) ;
#1548=VERTEX_POINT ( 'NONE', #2430 ) ;
#1555=CARTESIAN_POINT ( 'NONE',  ( -2.121784821874996396, -20.67475948316355883, -11.65237164579381535 ) ) ;
#1558=ORIENTED_EDGE ( 'NONE', *, *, #10050, .T. ) ;
#1562=VECTOR ( 'NONE', #1193, 1000.000000000000000 ) ;
#1563=CARTESIAN_POINT ( 'NONE',  ( -1.999999999999996225, -23.05761107341827199, -14.68767808793413998 ) ) ;
#1566=CARTESIAN_POINT ( 'NONE',  ( -2.121784821874996396, -18.09366551958387248, -7.966187446493337987 ) ) ;
#1570=ORIENTED_EDGE ( 'NONE', *, *, #1434, .T. ) ;
#1571=ORIENTED_EDGE ( 'NONE', *, *, #3061, .F. ) ;
#1576=EDGE_CURVE ( 'NONE', #17808, #9317, #9237, .T. ) ;
#1582=CARTESIAN_POINT ( 'NONE',  ( 4.713407268011036227E-15, -19.22951417349437619, -11.23374808423137949 ) ) ;
#1584=CARTESIAN_POINT ( 'NONE',  ( 0.000000000000000000, 5.977523610840987267, 32.81826849749789687 ) ) ;
#1587=CARTESIAN_POINT ( 'NONE',  ( -9.829077985114366811, -9.943001520064436605, 1.739096673092067613 ) ) ;
#1588=CARTESIAN_POINT ( 'NONE',  ( 4.730628863548789710E-15, -18.36998600877478793, -10.49655905817405355 ) ) ;
#1591=VERTEX_POINT ( 'NONE', #11027 ) ;
#1594=CARTESIAN_POINT ( 'NONE',  ( 4.299564228933482956E-15, -19.99451661891623289, -11.24743617014079078 ) ) ;
#1596=CARTESIAN_POINT ( 'NONE',  ( -1.999999999999996225, -18.66975133533280484, -8.421164949123328469 ) ) ;
#1599=CARTESIAN_POINT ( 'NONE',  ( 4.243569643749996345, -24.21874468437355432, -6.034981767721971480 ) ) ;
#1605=CARTESIAN_POINT ( 'NONE',  ( -4.243569643749997233, -21.14050350850180138, -10.18177799141198747 ) ) ;
#1606=DIRECTION ( 'NONE',  ( -0.000000000000000000, -0.5735764363510414965, -0.8191520442889950182 ) ) ;
#1609=CARTESIAN_POINT ( 'NONE',  ( -3.973088838427990765, -15.08697326462699095, -8.369503528064965892 ) ) ;
#1611=CARTESIAN_POINT ( 'NONE',  ( -4.000000000000004441, -26.62549532187730250, -9.717350097961160671 ) ) ;
#1612=CARTESIAN_POINT ( 'NONE',  ( 2.121784821875004390, -17.33009188869154826, -6.875691287533610918 ) ) ;
#1613=DIRECTION ( 'NONE',  ( 0.000000000000000000, 0.5150380737757255245, 0.8571673013836856869 ) ) ;
#1617=CARTESIAN_POINT ( 'NONE',  ( -4.243569643750005227, -28.69264088791166856, -12.42436771317613875 ) ) ;
#1620=CARTESIAN_POINT ( 'NONE',  ( 6.428571428571432378, -14.26578344203647930, -2.827263138854372748 ) ) ;
#1622=CARTESIAN_POINT ( 'NONE',  ( 4.243569643749997233, -22.18613318805455847, -3.132111710772846891 ) ) ;
#1624=CARTESIAN_POINT ( 'NONE',  ( 4.243569643750003451, -25.09818091932399398, -15.83392709700605039 ) ) ;
#1625=( BOUNDED_CURVE ( )  B_SPLINE_CURVE ( 2, ( #4738, #13167, #10097, #5937, #11680, #4638, #6123, #10289, #11587 ),
 .UNSPECIFIED., .F., .T. ) 
 B_SPLINE_CURVE_WITH_KNOTS ( ( 3, 2, 2, 2, 3 ),
 ( 0.07758620689655172653, 0.08045977011494252762, 0.08620689655172414367, 0.09195402298850574585, 0.09482758620689656082 ),
 .UNSPECIFIED. ) 
 CURVE ( )  GEOMETRIC_REPRESENTATION_ITEM ( )  RATIONAL_B_SPLINE_CURVE ( ( 0.9330127018922194093, 0.9330127018922194093, 1.000000000000000000, 0.8660254037844387076, 1.000000000000000000, 0.8660254037844387076, 1.000000000000000000, 0.9330127018922191873, 0.9330127018922194093 ) ) 
 REPRESENTATION_ITEM ( '' )  );
#1626=EDGE_CURVE ( 'NONE', #13968, #11829, #7434, .T. ) ;
#1627=EDGE_CURVE ( 'NONE', #14839, #14660, #13202, .T. ) ;
#1628=CARTESIAN_POINT ( 'NONE',  ( 2.121784821875004390, -23.26660800492483006, -15.35391494592470885 ) ) ;
#1629=DIRECTION ( 'NONE',  ( -0.000000000000000000, -0.5735764363510414965, -0.8191520442889950182 ) ) ;
#1630=CARTESIAN_POINT ( 'NONE',  ( -3.999999999999997335, -22.69143028182022803, -12.15155876676686830 ) ) ;
#1632=CARTESIAN_POINT ( 'NONE',  ( -2.121784821875005722, -27.60972853510210001, -8.742063539214022683 ) ) ;
#1633=CARTESIAN_POINT ( 'NONE',  ( -5.577813053751546416E-15, -28.74166284227092305, -9.792081248737861898 ) ) ;
#1634=CARTESIAN_POINT ( 'NONE',  ( -5.279047395330986450E-15, -24.66711410668581550, -2.894173961965647912 ) ) ;
#1636=ORIENTED_EDGE ( 'NONE', *, *, #15905, .T. ) ;
#1638=DIRECTION ( 'NONE',  ( 0.000000000000000000, 0.000000000000000000, 1.000000000000000000 ) ) ;
#1640=CARTESIAN_POINT ( 'NONE',  ( 4.299564228933482956E-15, -19.99451661891623289, -11.24743617014079078 ) ) ;
#1644=CARTESIAN_POINT ( 'NONE',  ( -5.330712181944246111E-15, -28.36584563134307047, -7.686165607253494514 ) ) ;
#1649=CARTESIAN_POINT ( 'NONE',  ( 4.000000000000000888, -22.81943335244577398, -8.308048189859038146 ) ) ;
#1650=CARTESIAN_POINT ( 'NONE',  ( 2.121784821874994176, -28.11519276963646519, -9.463941278243694910 ) ) ;
#1654=CARTESIAN_POINT ( 'NONE',  ( 4.243569643750003451, -19.67788359580665869, -8.092940278475046156 ) ) ;
#1656=CARTESIAN_POINT ( 'NONE',  ( 0.000000000000000000, 9.254131787996968228, 30.52396275209373044 ) ) ;
#1659=AXIS2_PLACEMENT_3D ( 'NONE', #14303, #16924, #205 ) ;
#1660=CARTESIAN_POINT ( 'NONE',  ( -1.071796769724486786, -17.20831390805418337, -7.268326322243626514 ) ) ;
#1665=AXIS2_PLACEMENT_3D ( 'NONE', #17115, #2921, #11522 ) ;
#1667=VERTEX_POINT ( 'NONE', #15754 ) ;
#1669=ADVANCED_FACE ( 'NONE', ( #8685 ), #18281, .F. ) ;
#1670=CARTESIAN_POINT ( 'NONE',  ( -5.279047395330986450E-15, -27.18368072047107020, -6.488203555276846224 ) ) ;
#1671=VERTEX_POINT ( 'NONE', #4813 ) ;
#1672=EDGE_CURVE ( 'NONE', #11075, #3556, #12208, .T. ) ;
#1676=CARTESIAN_POINT ( 'NONE',  ( 2.121784821874994176, -24.21128814972218990, -3.888587676801722903 ) ) ;
#1685=CARTESIAN_POINT ( 'NONE',  ( -2.000000000000005773, -28.90493584365338720, -10.95956958208364007 ) ) ;
#1688=EDGE_LOOP ( 'NONE', ( #4787, #12072, #16035, #6829 ) ) ;
#1691=CARTESIAN_POINT ( 'NONE',  ( -2.121784821874996396, -19.86816761954490573, -10.50043908351241662 ) ) ;
#1695=CARTESIAN_POINT ( 'NONE',  ( -2.121784821874996396, -23.51396284310121487, -15.70717426502434044 ) ) ;
#1697=CARTESIAN_POINT ( 'NONE',  ( -3.999999999999997335, -25.20799689560547918, -15.74558836007806839 ) ) ;
#1698=CARTESIAN_POINT ( 'NONE',  ( -4.243569643750005227, -24.85326361708688836, -6.941168716716678233 ) ) ;
#1699=DIRECTION ( 'NONE',  ( 0.000000000000000000, 0.8191520442889952403, -0.5735764363510413855 ) ) ;
#1700=EDGE_CURVE ( 'NONE', #8879, #3333, #8420, .T. ) ;
#1702=CARTESIAN_POINT ( 'NONE',  ( -2.220605816132459776, -15.34963770581800624, -10.14223552587114874 ) ) ;
#1707=CARTESIAN_POINT ( 'NONE',  ( 4.243569643750003451, -18.09696354311409294, -5.835152456403505106 ) ) ;
#1708=CARTESIAN_POINT ( 'NONE',  ( 2.000000000000004441, -21.81008232435476657, -12.90602239160557829 ) ) ;
#1709=CARTESIAN_POINT ( 'NONE',  ( 4.299564228933482956E-15, -19.47829782620029704, -10.51019933028069708 ) ) ;
#1712=CARTESIAN_POINT ( 'NONE',  ( -5.330712181944245322E-15, -30.39845712766207342, -10.58903566420261910 ) ) ;
#1715=DIRECTION ( 'NONE',  ( -1.000000000000000000, 0.000000000000000000, 0.000000000000000000 ) ) ;
#1716=CARTESIAN_POINT ( 'NONE',  ( 4.193264170086575149, -10.00000000000000533, -2.677076674082570218 ) ) ;
#1718=CARTESIAN_POINT ( 'NONE',  ( 2.121784821874994176, -22.95300484247709250, -2.091572879642740634 ) ) ;
#1721=CARTESIAN_POINT ( 'NONE',  ( -4.243569643750005227, -28.72490456245641965, -12.47044501566739427 ) ) ;
#1722=AXIS2_PLACEMENT_3D ( 'NONE', #17321, #4585, #17511 ) ;
#1723=CARTESIAN_POINT ( 'NONE',  ( -1.999999999999996225, -22.28328288434436644, -13.58182282814399855 ) ) ;
#1724=CARTESIAN_POINT ( 'NONE',  ( -4.243569643749998122, -23.94744319389470988, -14.19050330815125704 ) ) ;
#1725=CARTESIAN_POINT ( 'NONE',  ( 1.999999999999994449, -22.60276474854137874, -1.959136494451539035 ) ) ;
#1728=CARTESIAN_POINT ( 'NONE',  ( 4.730628863548789710E-15, -20.17675178328056873, -13.07688799768438948 ) ) ;
#1730=CARTESIAN_POINT ( 'NONE',  ( -5.279047395330986450E-15, -24.15089531396988320, -2.156937122105551108 ) ) ;
#1740=( BOUNDED_CURVE ( )  B_SPLINE_CURVE ( 2, ( #10773, #865, #689, #6334, #6420, #12159, #6604, #9107, #15143 ),
 .UNSPECIFIED., .F., .T. ) 
 B_SPLINE_CURVE_WITH_KNOTS ( ( 3, 2, 2, 2, 3 ),
 ( 0.5775862068965517127, 0.5804597701149425415, 0.5862068965517240882, 0.5919540229885057459, 0.5948275862068965747 ),
 .UNSPECIFIED. ) 
 CURVE ( )  GEOMETRIC_REPRESENTATION_ITEM ( )  RATIONAL_B_SPLINE_CURVE ( ( 0.9330127018922194093, 0.9330127018922194093, 1.000000000000000000, 0.8660254037844387076, 1.000000000000000000, 0.8660254037844387076, 1.000000000000000000, 0.9330127018922194093, 0.9330127018922194093 ) ) 
 REPRESENTATION_ITEM ( '' )  );
#1741=ORIENTED_EDGE ( 'NONE', *, *, #14309, .T. ) ;
#1743=CARTESIAN_POINT ( 'NONE',  ( -4.243569643750004339, -26.14381059887672976, -8.784260816366916913 ) ) ;
#1744=EDGE_CURVE ( 'NONE', #11984, #10307, #172, .T. ) ;
#1751=CARTESIAN_POINT ( 'NONE',  ( -3.999999999999997335, -20.62655511095648109, -9.202611407326488191 ) ) ;
#1752=CARTESIAN_POINT ( 'NONE',  ( 4.243569643750003451, -23.80763393753414903, -13.99083499735581171 ) ) ;
#1754=LINE ( 'NONE', #357, #10644 ) ;
#1755=CARTESIAN_POINT ( 'NONE',  ( -4.000000000000000888, -25.01336322148850044, -11.44130475926444745 ) ) ;
#1756=CARTESIAN_POINT ( 'NONE',  ( -4.243569643749997233, -19.59184713035399383, -7.970067471831701056 ) ) ;
#1758=CARTESIAN_POINT ( 'NONE',  ( 4.000000000000003553, -19.09940784846689610, -7.021619088400267827 ) ) ;
#1759=CARTESIAN_POINT ( 'NONE',  ( 4.898587196589413815E-16, 2.700915433685006750, 35.11257424290206330 ) ) ;
#1772=CARTESIAN_POINT ( 'NONE',  ( -2.000000000000005773, -24.96876754848942070, -5.338138677143647648 ) ) ;
#1774=LINE ( 'NONE', #3156, #12675 ) ;
#1775=( BOUNDED_CURVE ( )  B_SPLINE_CURVE ( 3, ( #11679, #6405, #4737, #8900 ),
 .UNSPECIFIED., .F., .F. ) 
 B_SPLINE_CURVE_WITH_KNOTS ( ( 4, 4 ),
 ( 2.111895852752043279, 4.171289454427544285 ),
 .UNSPECIFIED. ) 
 CURVE ( )  GEOMETRIC_REPRESENTATION_ITEM ( )  RATIONAL_B_SPLINE_CURVE ( ( 1.000000000000000000, 0.6767191690918086255, 0.6767191690918086255, 1.000000000000000000 ) ) 
 REPRESENTATION_ITEM ( '' )  );
#1777=CARTESIAN_POINT ( 'NONE',  ( -9.350946484394057734, -10.00000000000000178, 13.61740000484205915 ) ) ;
#1778=VECTOR ( 'NONE', #10163, 1000.000000000000000 ) ;
#1779=CARTESIAN_POINT ( 'NONE',  ( 4.243569643749997233, -23.44441649529964877, -4.929126507931827383 ) ) ;
#1790=CARTESIAN_POINT ( 'NONE',  ( 2.121784821875004390, -18.62063887048139321, -8.718783387183849598 ) ) ;
#1793=CARTESIAN_POINT ( 'NONE',  ( -5.330712181944246111E-15, -30.68883019856478711, -11.00373138662392236 ) ) ;
#1794=FACE_OUTER_BOUND ( 'NONE', #15943, .T. ) ;
#1795=EDGE_CURVE ( 'NONE', #2086, #16968, #8361, .T. ) ;
#1796=CARTESIAN_POINT ( 'NONE',  ( -4.243569643750000786, -23.12593826097332794, -8.745782564029356720 ) ) ;
#1797=DIRECTION ( 'NONE',  ( -0.000000000000000000, 1.000000000000000000, -0.000000000000000000 ) ) ;
#1805=CARTESIAN_POINT ( 'NONE',  ( 4.000000000000000888, -25.65863671238343358, -12.36285080908956502 ) ) ;
#1806=VERTEX_POINT ( 'NONE', #4812 ) ;
#1808=CARTESIAN_POINT ( 'NONE',  ( -5.330712181944245322E-15, -29.88223833494613402, -9.851798824342527183 ) ) ;
#1811=ADVANCED_FACE ( 'NONE', ( #6100 ), #17256, .F. ) ;
#1812=CARTESIAN_POINT ( 'NONE',  ( 5.679766210340737587, -14.60833734475391665, -5.139172057956870709 ) ) ;
#1816=CARTESIAN_POINT ( 'NONE',  ( 4.243569643750000786, -26.35230571544794387, -13.35351281315494987 ) ) ;
#1817=CARTESIAN_POINT ( 'NONE',  ( -4.000000000000000888, -24.23903503241459845, -10.33544949947430425 ) ) ;
#1818=CARTESIAN_POINT ( 'NONE',  ( -4.243569643750004339, -28.17642209519573271, -11.68713087331604150 ) ) ;
#1821=CARTESIAN_POINT ( 'NONE',  ( 3.999999999999996447, -27.89453318800893555, -11.52972399695732442 ) ) ;
#1822=CARTESIAN_POINT ( 'NONE',  ( -4.243569643749997233, -22.91500560846283463, -12.71602962843106432 ) ) ;
#1823=LINE ( 'NONE', #15822, #7712 ) ;
#1824=CARTESIAN_POINT ( 'NONE',  ( 2.000000000000004441, -17.16411318991132617, -6.270890832864717268 ) ) ;
#1827=ORIENTED_EDGE ( 'NONE', *, *, #4057, .F. ) ;
#1829=LINE ( 'NONE', #11726, #3633 ) ;
#1831=CARTESIAN_POINT ( 'NONE',  ( 2.000000000000004441, -23.35873870250257767, -15.11773291118586293 ) ) ;
#1832=LINE ( 'NONE', #7558, #4246 ) ;
#1834=VERTEX_POINT ( 'NONE', #9162 ) ;
#1835=CARTESIAN_POINT ( 'NONE',  ( 4.243569643750000786, -23.77121175186825752, -9.667328613854474284 ) ) ;
#1837=ORIENTED_EDGE ( 'NONE', *, *, #4785, .T. ) ;
#1839=CARTESIAN_POINT ( 'NONE',  ( -3.706921591972381904E-14, -18.18775084441045209, -8.667107230630458403 ) ) ;
#1841=EDGE_CURVE ( 'NONE', #8838, #17169, #10437, .T. ) ;
#1842=CARTESIAN_POINT ( 'NONE',  ( -2.121784821874996396, -22.99774405038527547, -14.96993742516424497 ) ) ;
#1844=CARTESIAN_POINT ( 'NONE',  ( 5.040478647146456659, -10.97734431112249887, 19.36653379754666560 ) ) ;
#1847=CARTESIAN_POINT ( 'NONE',  ( -2.121784821875005722, -25.06089824606716476, -5.101956642404802622 ) ) ;
#1848=ORIENTED_EDGE ( 'NONE', *, *, #15782, .F. ) ;
#1849=CARTESIAN_POINT ( 'NONE',  ( -1.661723472263481630E-14, -20.31715336506863423, -11.70820919606011579 ) ) ;
#1850=FACE_OUTER_BOUND ( 'NONE', #1901, .T. ) ;
#1853=ORIENTED_EDGE ( 'NONE', *, *, #3887, .F. ) ;
#1855=( BOUNDED_CURVE ( )  B_SPLINE_CURVE ( 2, ( #3393, #9033, #1725, #7358, #9220 ),
 .UNSPECIFIED., .F., .T. ) 
 B_SPLINE_CURVE_WITH_KNOTS ( ( 3, 2, 3 ),
 ( 0.9913793103448276245, 0.9942528735632183423, 0.9961881965693012431 ),
 .UNSPECIFIED. ) 
 CURVE ( )  GEOMETRIC_REPRESENTATION_ITEM ( )  RATIONAL_B_SPLINE_CURVE ( ( 0.9330127018922194093, 0.9330127018922206306, 1.000000000000000000, 0.9548845634181245545, 0.9401540307727882517 ) ) 
 REPRESENTATION_ITEM ( '' )  );
#1856=CARTESIAN_POINT ( 'NONE',  ( 4.000000000000000888, -24.17450768403005767, -10.24329489549855410 ) ) ;
#1863=CONICAL_SURFACE ( 'NONE', #11899, 2.000000000000001776, 1.029744260000000189 ) ;
#1864=ORIENTED_EDGE ( 'NONE', *, *, #10960, .T. ) ;
#1866=CARTESIAN_POINT ( 'NONE',  ( -3.999999999999997335, -20.30391836480407619, -8.741838381407161407 ) ) ;
#1868=AXIS2_PLACEMENT_3D ( 'NONE', #10362, #2044, #8979 ) ;
#1872=CARTESIAN_POINT ( 'NONE',  ( -7.736359789466761505, -10.27164672540018309, 8.681487574489553438 ) ) ;
#1873=CARTESIAN_POINT ( 'NONE',  ( -4.243569643750004339, -23.27234356439432972, -4.683380894645134518 ) ) ;
#1879=CARTESIAN_POINT ( 'NONE',  ( -4.000000000000003553, -2.343145750507614533, 25.02027108472330141 ) ) ;
#1883=CARTESIAN_POINT ( 'NONE',  ( -1.661723472263481630E-14, -21.54317299706404754, -13.45914668972107897 ) ) ;
#1888=CARTESIAN_POINT ( 'NONE',  ( -4.243569643749997233, -19.81769285216720888, -8.292608589270493269 ) ) ;
#1891=CARTESIAN_POINT ( 'NONE',  ( 4.243569643750003451, -24.58196212660805458, -15.09669025714595314 ) ) ;
#1892=( BOUNDED_CURVE ( )  B_SPLINE_CURVE ( 2, ( #13286, #17587, #9206, #3560, #1995, #693, #16358, #9113, #598 ),
 .UNSPECIFIED., .F., .F. ) 
 B_SPLINE_CURVE_WITH_KNOTS ( ( 3, 2, 2, 2, 3 ),
 ( 0.8534482758620689502, 0.8563218390804597790, 0.8620689655172413257, 0.8678160919540229834, 0.8706896551724138122 ),
 .UNSPECIFIED. ) 
 CURVE ( )  GEOMETRIC_REPRESENTATION_ITEM ( )  RATIONAL_B_SPLINE_CURVE ( ( 0.9330127018922194093, 0.9330127018922194093, 1.000000000000000000, 0.8660254037844387076, 1.000000000000000000, 0.8660254037844387076, 1.000000000000000000, 0.9330127018922194093, 0.9330127018922194093 ) ) 
 REPRESENTATION_ITEM ( '' )  );
#1893=CARTESIAN_POINT ( 'NONE',  ( -5.279047395330986450E-15, -30.28099347676669240, -10.91162459443741817 ) ) ;
#1894=CARTESIAN_POINT ( 'NONE',  ( 4.243569643750003451, -19.93599299216462484, -8.461558698405095669 ) ) ;
#1899=CARTESIAN_POINT ( 'NONE',  ( 1.999999999999994449, -23.11898354125731458, -2.696373334311634284 ) ) ;
#1901=EDGE_LOOP ( 'NONE', ( #7877, #7597, #7826, #3052 ) ) ;
#1903=CARTESIAN_POINT ( 'NONE',  ( 4.243569643750000786, -19.86730713195397868, -4.091975012412500945 ) ) ;
#1905=CARTESIAN_POINT ( 'NONE',  ( -8.500000000000005329, 0.000000000000000000, 20.49999999999999645 ) ) ;
#1906=ORIENTED_EDGE ( 'NONE', *, *, #62, .F. ) ;
#1908=CARTESIAN_POINT ( 'NONE',  ( 4.730628863548789710E-15, -21.72540816142837983, -15.28859851726467589 ) ) ;
#1913=CARTESIAN_POINT ( 'NONE',  ( 4.242943609565477558, -15.02914320863476405, -7.979206348031381957 ) ) ;
#1916=CARTESIAN_POINT ( 'NONE',  ( -4.243569643749997233, -24.75403505751336297, -15.34243587043265755 ) ) ;
#1919=CARTESIAN_POINT ( 'NONE',  ( 4.730628863548789710E-15, -19.91864238692259903, -12.70826957775434174 ) ) ;
#1920=DIRECTION ( 'NONE',  ( -0.000000000000000000, 1.000000000000000000, -0.000000000000000000 ) ) ;
#1925=CARTESIAN_POINT ( 'NONE',  ( 2.121784821874994176, -26.27616332058593684, -6.837535036242106123 ) ) ;
#1927=CARTESIAN_POINT ( 'NONE',  ( 4.299564228933482956E-15, -17.21984060877302269, -7.284788156899542066 ) ) ;
#1928=ADVANCED_FACE ( 'NONE', ( #366 ), #649, .F. ) ;
#1930=CARTESIAN_POINT ( 'NONE',  ( 0.000000000000000000, 9.254131787996968228, 30.52396275209373044 ) ) ;
#1934=CARTESIAN_POINT ( 'NONE',  ( 4.713407268011036227E-15, -22.90757307230037654, -16.48656056924132329 ) ) ;
#1938=CARTESIAN_POINT ( 'NONE',  ( 4.243569643749997233, -25.28344594435018777, -7.555532749933419723 ) ) ;
#1940=EDGE_LOOP ( 'NONE', ( #7830, #2785, #12942 ) ) ;
#1943=CARTESIAN_POINT ( 'NONE',  ( -4.243569643749997233, -22.94726928300758217, -12.76210693092232162 ) ) ;
#1944=CARTESIAN_POINT ( 'NONE',  ( 4.000000000000000888, -26.69107429781530527, -13.83732448880975419 ) ) ;
#1946=CARTESIAN_POINT ( 'NONE',  ( -6.158835246850665095E-15, -22.12391913957442569, -14.28853813557044639 ) ) ;
#1947=CARTESIAN_POINT ( 'NONE',  ( -4.243569643749997233, -18.30130014856414533, -6.126975372181463264 ) ) ;
#1949=CARTESIAN_POINT ( 'NONE',  ( -4.000000000000007105, 6.938893903907228378E-15, 30.00000000000000000 ) ) ;
#1950=CARTESIAN_POINT ( 'NONE',  ( -3.999999999999997335, -21.14277390367241694, -9.939848247186581887 ) ) ;
#1951=CARTESIAN_POINT ( 'NONE',  ( -5.577813053751546416E-15, -28.54808079570739920, -9.515617434797091434 ) ) ;
#1952=ORIENTED_EDGE ( 'NONE', *, *, #1019, .F. ) ;
#1954=CARTESIAN_POINT ( 'NONE',  ( 0.000000000000000000, 5.977523610840987267, 32.81826849749789687 ) ) ;
#1955=DIRECTION ( 'NONE',  ( -0.000000000000000000, -0.5735764363510414965, -0.8191520442889950182 ) ) ;
#1961=CARTESIAN_POINT ( 'NONE',  ( 3.999999999999996447, -23.95836489284496906, -5.908293092017330217 ) ) ;
#1962=ORIENTED_EDGE ( 'NONE', *, *, #12426, .F. ) ;
#1963=ADVANCED_FACE ( 'NONE', ( #13238 ), #3428, .T. ) ;
#1966=FACE_OUTER_BOUND ( 'NONE', #11914, .T. ) ;
#1967=CARTESIAN_POINT ( 'NONE',  ( -4.243569643750004339, -23.01423416803636002, -4.314762474715088558 ) ) ;
#1968=( BOUNDED_CURVE ( )  B_SPLINE_CURVE ( 2, ( #638, #447, #17626, #6088, #14544, #11738, #10351, #11931, #3321 ),
 .UNSPECIFIED., .F., .T. ) 
 B_SPLINE_CURVE_WITH_KNOTS ( ( 3, 2, 2, 2, 3 ),
 ( 0.2155172413793103592, 0.2183908045977011603, 0.2241379310344827624, 0.2298850574712643646, 0.2327586206896551657 ),
 .UNSPECIFIED. ) 
 CURVE ( )  GEOMETRIC_REPRESENTATION_ITEM ( )  RATIONAL_B_SPLINE_CURVE ( ( 0.9330127018922192983, 0.9330127018922196314, 1.000000000000000000, 0.8660254037844387076, 1.000000000000000000, 0.8660254037844387076, 1.000000000000000000, 0.9330127018922194093, 0.9330127018922194093 ) ) 
 REPRESENTATION_ITEM ( '' )  );
#1979=CARTESIAN_POINT ( 'NONE',  ( 4.243569643749996345, -23.96063528801558462, -5.666363347791923744 ) ) ;
#1981=EDGE_CURVE ( 'NONE', #9801, #3352, #13338, .T. ) ;
#1983=CARTESIAN_POINT ( 'NONE',  ( -4.243569643750004339, -28.46679516609844995, -12.10182659573734476 ) ) ;
#1985=CARTESIAN_POINT ( 'NONE',  ( 4.713407268011036227E-15, -21.81060813707406609, -14.91993228353185508 ) ) ;
#1987=CARTESIAN_POINT ( 'NONE',  ( -4.243569643750005227, -23.30460723893907371, -4.729458197136391817 ) ) ;
#1989=FACE_OUTER_BOUND ( 'NONE', #3979, .T. ) ;
#1990=CARTESIAN_POINT ( 'NONE',  ( -4.000000000000004441, -27.39982351095120805, -10.82320535775130743 ) ) ;
#1992=DIRECTION ( 'NONE',  ( 0.000000000000000000, 0.8191520442889952403, -0.5735764363510413855 ) ) ;
#1994=EDGE_LOOP ( 'NONE', ( #11832, #10181, #7563, #17488 ) ) ;
#1995=CARTESIAN_POINT ( 'NONE',  ( 4.000000000000000888, -20.75455818158202703, -5.359100830418656258 ) ) ;
#1996=ORIENTED_EDGE ( 'NONE', *, *, #3630, .F. ) ;
#1999=VECTOR ( 'NONE', #2736, 1000.000000000000000 ) ;
#2000=CARTESIAN_POINT ( 'NONE',  ( 4.243569643749996345, -28.09038562974308562, -11.56425806667268752 ) ) ;
#2003=CARTESIAN_POINT ( 'NONE',  ( 1.848264997552677702, -9.999999999999433342, -4.668605916318575133 ) ) ;
#2005=CARTESIAN_POINT ( 'NONE',  ( 4.243569643750000786, -25.31986813001606862, -11.87903913343475892 ) ) ;
#2007=CARTESIAN_POINT ( 'NONE',  ( -1.071796769724481457, -21.85428304249762022, -13.90345788098448665 ) ) ;
#2009=CARTESIAN_POINT ( 'NONE',  ( -2.121784821875005722, -27.60972853510210001, -8.742063539214022683 ) ) ;
#2010=CARTESIAN_POINT ( 'NONE',  ( -6.938893903907228378E-15, 6.938893903907228378E-15, 30.00000000000000000 ) ) ;
#2011=CARTESIAN_POINT ( 'NONE',  ( 0.000000000000000000, 9.254131787996968228, 30.52396275209373044 ) ) ;
#2013=CARTESIAN_POINT ( 'NONE',  ( 2.121784821874994176, -27.05049150965984595, -7.943390296032248443 ) ) ;
#2015=CARTESIAN_POINT ( 'NONE',  ( -4.000000000000000888, -19.65759324776559680, -3.792472546722722715 ) ) ;
#2017=ORIENTED_EDGE ( 'NONE', *, *, #17101, .T. ) ;
#2019=CARTESIAN_POINT ( 'NONE',  ( 1.071796769724494780, -27.76222590591464723, -8.393300340351034450 ) ) ;
#2026=ORIENTED_EDGE ( 'NONE', *, *, #14309, .F. ) ;
#2027=CARTESIAN_POINT ( 'NONE',  ( -4.243569643750004339, -24.59515422072892221, -6.572550296786629609 ) ) ;
#2029=ORIENTED_EDGE ( 'NONE', *, *, #6657, .F. ) ;
#2033=CARTESIAN_POINT ( 'NONE',  ( 4.730628863548789710E-15, -20.98334364689921827, -14.22882055996578643 ) ) ;
#2037=CARTESIAN_POINT ( 'NONE',  ( 4.243569643750003451, -24.80780784842128028, -15.41923137458474535 ) ) ;
#2039=CARTESIAN_POINT ( 'NONE',  ( -4.000000000000000888, -19.91570264412356650, -4.161090966652770895 ) ) ;
#2040=CARTESIAN_POINT ( 'NONE',  ( 4.000000000000003553, -20.97070097276710854, -9.694102633899879251 ) ) ;
#2042=ORIENTED_EDGE ( 'NONE', *, *, #609, .T. ) ;
#2044=DIRECTION ( 'NONE',  ( -0.000000000000000000, -0.5735764363510414965, -0.8191520442889950182 ) ) ;
#2047=CARTESIAN_POINT ( 'NONE',  ( 3.579096709490575479E-14, -23.83758431146952361, -2.788331270066955359 ) ) ;
#2049=ORIENTED_EDGE ( 'NONE', *, *, #11410, .F. ) ;
#2054=CARTESIAN_POINT ( 'NONE',  ( -4.000000000000004441, -23.52818256558167320, -5.293929058800590504 ) ) ;
#2059=CARTESIAN_POINT ( 'NONE',  ( 2.121784821875004390, -19.13685766319732906, -9.456020227043945070 ) ) ;
#2060=CARTESIAN_POINT ( 'NONE',  ( -5.330712181944245322E-15, -27.59151744226915781, -6.580310347463352194 ) ) ;
#2065=CARTESIAN_POINT ( 'NONE',  ( 7.971931588564637572, -10.00000000000000178, 17.73270869615947021 ) ) ;
#2067=CARTESIAN_POINT ( 'NONE',  ( 4.000000000000003553, -20.19637278369320299, -8.588247374109734267 ) ) ;
#2068=CARTESIAN_POINT ( 'NONE',  ( -1.071796769724505882, -19.53129847527590712, -10.58589210161404814 ) ) ;
#2069=VERTEX_POINT ( 'NONE', #18301 ) ;
#2072=CARTESIAN_POINT ( 'NONE',  ( -4.243569643749997233, -19.04336466309330689, -7.186753329480350061 ) ) ;
#2075=CARTESIAN_POINT ( 'NONE',  ( 4.243569643750003451, -24.84007152296602428, -15.46530867707600088 ) ) ;
#2076=CARTESIAN_POINT ( 'NONE',  ( -4.000000000000000888, -26.56201959963631509, -13.65301527884473387 ) ) ;
#2077=VECTOR ( 'NONE', #8869, 1000.000000000000000 ) ;
#2078=CARTESIAN_POINT ( 'NONE',  ( -2.121784821875005722, -24.80278884970919506, -4.733338222474753998 ) ) ;
#2081=EDGE_CURVE ( 'NONE', #5846, #12141, #3843, .T. ) ;
#2083=EDGE_CURVE ( 'NONE', #3510, #1667, #1151, .T. ) ;
#2086=VERTEX_POINT ( 'NONE', #17251 ) ;
#2088=CARTESIAN_POINT ( 'NONE',  ( -5.577813053751546416E-15, -28.99977223862889275, -10.16069966866791141 ) ) ;
#2090=EDGE_CURVE ( 'NONE', #2141, #13230, #16907, .T. ) ;
#2091=ORIENTED_EDGE ( 'NONE', *, *, #7137, .F. ) ;
#2093=CARTESIAN_POINT ( 'NONE',  ( 2.121784821874994176, -28.85725728416562674, -10.52371923554258260 ) ) ;
#2095=ADVANCED_FACE ( 'NONE', ( #1850 ), #2804, .F. ) ;
#2097=CARTESIAN_POINT ( 'NONE',  ( 0.6850780354679415485, -10.00000000000053113, -5.037014450714041303 ) ) ;
#2098=CARTESIAN_POINT ( 'NONE',  ( 2.121784821875004390, -22.78265288675364175, -14.66275540855586890 ) ) ;
#2102=CARTESIAN_POINT ( 'NONE',  ( 4.730628863548789710E-15, -20.17675178328056873, -13.07688799768438948 ) ) ;
#2105=DIRECTION ( 'NONE',  ( -0.000000000000000000, -0.5735764363510414965, -0.8191520442889950182 ) ) ;
#2107=CARTESIAN_POINT ( 'NONE',  ( -5.330712181944245322E-15, -27.55925376772441382, -6.534233044972094895 ) ) ;
#2110=DIRECTION ( 'NONE',  ( -0.000000000000000000, -0.5735764363510414965, -0.8191520442889950182 ) ) ;
#2114=CARTESIAN_POINT ( 'NONE',  ( -1.999999999999996225, -23.83193926249218109, -15.79353334772428497 ) ) ;
#2120=CARTESIAN_POINT ( 'NONE',  ( -2.121784821874996396, -19.38421250137371388, -9.809279546143578443 ) ) ;
#2125=CARTESIAN_POINT ( 'NONE',  ( -3.924030842084162085, -26.26574055918599626, -14.95313944102314707 ) ) ;
#2126=DIRECTION ( 'NONE',  ( 0.000000000000000000, 0.000000000000000000, 1.000000000000000000 ) ) ;
#2128=CARTESIAN_POINT ( 'NONE',  ( 7.338942192890510086, -12.39130301598704520, 9.345622607077766375 ) ) ;
#2130=CARTESIAN_POINT ( 'NONE',  ( -4.243569643750005227, -22.01406025714923231, -2.886366097486154469 ) ) ;
#2133=CARTESIAN_POINT ( 'NONE',  ( 1.999999999999994449, -25.50649545827347353, -6.106093719671341624 ) ) ;
#2136=CARTESIAN_POINT ( 'NONE',  ( -2.000000000000005773, -24.19443935941551160, -4.232283417353504440 ) ) ;
#2141=VERTEX_POINT ( 'NONE', #11744 ) ;
#2144=CARTESIAN_POINT ( 'NONE',  ( 4.713407268011036227E-15, -17.93896719170453835, -9.390655984581140814 ) ) ;
#2151=CARTESIAN_POINT ( 'NONE',  ( 4.730628863548789710E-15, -15.78889204519509981, -6.810374858873577075 ) ) ;
#2152=CARTESIAN_POINT ( 'NONE',  ( -4.243569643750005227, -26.66002939159267271, -9.521497656227012385 ) ) ;
#2154=CARTESIAN_POINT ( 'NONE',  ( 1.071796769724495224, -23.16788342572513315, -15.77947364994655288 ) ) ;
#2156=ORIENTED_EDGE ( 'NONE', *, *, #10788, .F. ) ;
#2157=CARTESIAN_POINT ( 'NONE',  ( 0.000000000000000000, -10.00000000000000178, -12.59063537424807677 ) ) ;
#2160=CARTESIAN_POINT ( 'NONE',  ( 4.243569643750003451, -24.58196212660805458, -15.09669025714595314 ) ) ;
#2161=ORIENTED_EDGE ( 'NONE', *, *, #3935, .T. ) ;
#2164=CARTESIAN_POINT ( 'NONE',  ( -2.121784821875005722, -24.51241577880647782, -4.318642500053448963 ) ) ;
#2169=CARTESIAN_POINT ( 'NONE',  ( 2.121784821875004390, -23.04076228311161145, -15.03137382848591663 ) ) ;
#2170=CARTESIAN_POINT ( 'NONE',  ( -1.999999999999996225, -23.50930251633977264, -15.33276032180496173 ) ) ;
#2171=CARTESIAN_POINT ( 'NONE',  ( 2.121784821875004390, -18.91101194138411046, -9.133479109605152857 ) ) ;
#2175=VECTOR ( 'NONE', #4556, 999.9999999999998863 ) ;
#2176=CARTESIAN_POINT ( 'NONE',  ( -5.040478647146447777, -15.02265568887750646, -7.935421837999481198 ) ) ;
#2179=ORIENTED_EDGE ( 'NONE', *, *, #3658, .T. ) ;
#2183=CARTESIAN_POINT ( 'NONE',  ( 3.999999999999996447, -27.83000583821450036, -11.43756939096804714 ) ) ;
#2186=( NAMED_UNIT ( * ) PLANE_ANGLE_UNIT ( ) SI_UNIT ( $, .RADIAN. ) );
#2187=CARTESIAN_POINT ( 'NONE',  ( 2.121784821874994176, -28.34103849144968379, -9.786482395682487123 ) ) ;
#2191=EDGE_CURVE ( 'NONE', #5572, #4695, #3256, .T. ) ;
#2193=CIRCLE ( 'NONE', #1298, 6.000000000000000000 ) ;
#2194=CARTESIAN_POINT ( 'NONE',  ( -4.243569643750000786, -25.44892282819504459, -12.06334834339978634 ) ) ;
#2197=LINE ( 'NONE', #13662, #11458 ) ;
#2198=CARTESIAN_POINT ( 'NONE',  ( 4.243569643750000786, -22.70651049189163828, -8.146777631643026041 ) ) ;
#2200=DIRECTION ( 'NONE',  ( -0.000000000000000000, -0.5735764363510414965, -0.8191520442889950182 ) ) ;
#2211=ORIENTED_EDGE ( 'NONE', *, *, #8240, .F. ) ;
#2212=CARTESIAN_POINT ( 'NONE',  ( 2.121784821875004390, -19.16912133774208016, -9.502097529535200593 ) ) ;
#2220=CARTESIAN_POINT ( 'NONE',  ( 6.931282879835348076, -10.37761417744432002, 2.815650091973651126 ) ) ;
#2221=CARTESIAN_POINT ( 'NONE',  ( 4.299564228933482956E-15, -18.51038759056286054, -9.127880256549779858 ) ) ;
#2223=CARTESIAN_POINT ( 'NONE',  ( -2.121784821875005722, -23.51224186791935011, -2.890246122824515318 ) ) ;
#2224=ORIENTED_EDGE ( 'NONE', *, *, #2965, .T. ) ;
#2225=CARTESIAN_POINT ( 'NONE',  ( -4.000000000000004441, -25.39947568988189985, -7.966412604300202815 ) ) ;
#2226=ORIENTED_EDGE ( 'NONE', *, *, #10859, .F. ) ;
#2228=DIRECTION ( 'NONE',  ( -0.000000000000000000, 1.000000000000000000, -0.000000000000000000 ) ) ;
#2235=VECTOR ( 'NONE', #10376, 1000.000000000000000 ) ;
#2236=CARTESIAN_POINT ( 'NONE',  ( 3.999999999999996447, -22.92592730741309737, -4.433819412297139273 ) ) ;
#2240=( BOUNDED_CURVE ( )  B_SPLINE_CURVE ( 3, ( #14878, #2176, #16351, #6510 ),
 .UNSPECIFIED., .F., .F. ) 
 B_SPLINE_CURVE_WITH_KNOTS ( ( 4, 4 ),
 ( 5.253488506341836839, 6.283185307179586232 ),
 .UNSPECIFIED. ) 
 CURVE ( )  GEOMETRIC_REPRESENTATION_ITEM ( )  RATIONAL_B_SPLINE_CURVE ( ( 1.000000000000000000, 0.9135782535825738293, 0.9135782535825738293, 1.000000000000000000 ) ) 
 REPRESENTATION_ITEM ( '' )  );
#2241=CARTESIAN_POINT ( 'NONE',  ( -8.500000000000005329, 10.00000000000000000, 20.49999999999999645 ) ) ;
#2244=CARTESIAN_POINT ( 'NONE',  ( 2.121784821875004390, -21.49210590496380036, -12.81966330890563022 ) ) ;
#2245=CARTESIAN_POINT ( 'NONE',  ( 2.884887816493423518, -29.26500710983614084, -12.65241590468473909 ) ) ;
#2248=CARTESIAN_POINT ( 'NONE',  ( 6.503403972914452602, -9.999999999998879119, 16.98026834952917952 ) ) ;
#2249=CARTESIAN_POINT ( 'NONE',  ( 4.299564228933482956E-15, -17.15531325897858039, -7.192633550910265683 ) ) ;
#2251=CARTESIAN_POINT ( 'NONE',  ( -1.999999999999996225, -19.96029831712264979, -10.26425704877356715 ) ) ;
#2255=CARTESIAN_POINT ( 'NONE',  ( -4.243569643750000786, -20.77069001920686375, -5.382139482167671574 ) ) ;
#2258=CARTESIAN_POINT ( 'NONE',  ( 4.000000000000000888, -26.17485550509936942, -13.10008764894965871 ) ) ;
#2260=ADVANCED_FACE ( 'NONE', ( #6121 ), #2893, .F. ) ;
#2261=CARTESIAN_POINT ( 'NONE',  ( 4.243569643749996345, -22.70235198077049787, -3.869348550632942363 ) ) ;
#2270=DIRECTION ( 'NONE',  ( 0.000000000000000000, 0.8191520442889952403, -0.5735764363510413855 ) ) ;
#2271=CARTESIAN_POINT ( 'NONE',  ( 6.774437128121542528, -14.04910375689483537, -1.424172483101618036 ) ) ;
#2274=CARTESIAN_POINT ( 'NONE',  ( 4.730628863548789710E-15, -20.43486117963853843, -13.44550641761443366 ) ) ;
#2277=LINE ( 'NONE', #12077, #418 ) ;
#2279=CARTESIAN_POINT ( 'NONE',  ( 4.243569643750003451, -23.29141514481821318, -13.25359815749571268 ) ) ;
#2281=CYLINDRICAL_SURFACE ( 'NONE', #8778, 4.000000000000000000 ) ;
#2283=CARTESIAN_POINT ( 'NONE',  ( 8.500000000000019540, 10.00000000000000000, -18.49999999999998934 ) ) ;
#2284=DIRECTION ( 'NONE',  ( -0.000000000000000000, -0.5735764363510414965, -0.8191520442889950182 ) ) ;
#2285=VECTOR ( 'NONE', #1273, 1000.000000000000000 ) ;
#2286=CARTESIAN_POINT ( 'NONE',  ( 4.730628863548789710E-15, -18.88620480149072378, -11.23379589803414902 ) ) ;
#2287=ORIENTED_EDGE ( 'NONE', *, *, #3935, .F. ) ;
#2289=CYLINDRICAL_SURFACE ( 'NONE', #8855, 4.000000000000000000 ) ;
#2291=ORIENTED_EDGE ( 'NONE', *, *, #16828, .T. ) ;
#2293=CARTESIAN_POINT ( 'NONE',  ( -4.000000000000004441, -28.49678844617752205, -12.38983364346077565 ) ) ;
#2296=CARTESIAN_POINT ( 'NONE',  ( 4.243569643750003451, -20.96843057759648943, -9.936032378125284836 ) ) ;
#2299=EDGE_LOOP ( 'NONE', ( #9471, #2364, #2750, #3687 ) ) ;
#2300=CARTESIAN_POINT ( 'NONE',  ( -5.577813053751546416E-15, -29.51599103134483570, -10.89793650852800511 ) ) ;
#2301=CARTESIAN_POINT ( 'NONE',  ( 1.533898589781675205E-14, -27.51564321027552040, -8.041143755076902266 ) ) ;
#2302=CARTESIAN_POINT ( 'NONE',  ( -3.658469487637143303, -25.65435779525035898, -15.39514208652095029 ) ) ;
#2303=CARTESIAN_POINT ( 'NONE',  ( 7.076300148717182381, -12.11289111431826448, 11.47713140425214284 ) ) ;
#2305=CARTESIAN_POINT ( 'NONE',  ( 4.243569643750003451, -25.06591724477924288, -15.78784979451479309 ) ) ;
#2307=VERTEX_POINT ( 'NONE', #4736 ) ;
#2309=CARTESIAN_POINT ( 'NONE',  ( 4.000000000000003553, -20.71259157640914239, -9.325484213969829739 ) ) ;
#2315=VERTEX_POINT ( 'NONE', #15970 ) ;
#2321=ORIENTED_EDGE ( 'NONE', *, *, #5925, .T. ) ;
#2324=CARTESIAN_POINT ( 'NONE',  ( -1.999999999999996225, -18.08900519282243025, -7.591773503273958390 ) ) ;
#2327=CARTESIAN_POINT ( 'NONE',  ( -1.071796769724505882, -18.43433354004959668, -9.019263815904585257 ) ) ;
#2328=CIRCLE ( 'NONE', #7927, 2.000000000000001776 ) ;
#2332=CARTESIAN_POINT ( 'NONE',  ( 2.121784821875004390, -17.33009188869154826, -6.875691287533610918 ) ) ;
#2333=CARTESIAN_POINT ( 'NONE',  ( 4.730628863548789710E-15, -20.72523425054125212, -13.86020214003574047 ) ) ;
#2335=DIRECTION ( 'NONE',  ( -0.000000000000000000, -0.5735764363510414965, -0.8191520442889950182 ) ) ;
#2337=CARTESIAN_POINT ( 'NONE',  ( 0.9009846993710122209, -10.00000000000000178, 24.02174733379527538 ) ) ;
#2341=CARTESIAN_POINT ( 'NONE',  ( 4.243569643750003451, -24.32385273025008843, -14.72807183721590718 ) ) ;
#2343=AXIS2_PLACEMENT_3D ( 'NONE', #16824, #4098, #9748 ) ;
#2346=CIRCLE ( 'NONE', #8821, 7.500000000000000888 ) ;
#2347=CARTESIAN_POINT ( 'NONE',  ( 4.243569643749996345, -22.41197890986777352, -3.454652828211636884 ) ) ;
#2350=CARTESIAN_POINT ( 'NONE',  ( 1.999999999999994449, -27.50684327934278528, -8.962886473122447129 ) ) ;
#2351=( BOUNDED_CURVE ( )  B_SPLINE_CURVE ( 2, ( #10903, #1000, #4036, #1357, #18341, #15460, #1272, #12381, #16946, #18250, #5614, #15093, #12289, #6819, #8026, #6641, #16581, #5521, #9506, #15184, #13777, #11079, #10993, #1089, #18071, #5341, #16765, #9685, #15368, #3950, #15275, #2576, #8208, #2668, #13872, #8302, #15909, #11432, #1628, #5706, #49, #8469, #3019, #1818, #12748, #14139, #17220, #3205, #7455, #17318, #14420, #1539, #11714, #1724, #4582, #6062, #7083, #14329, #5970, #15542, #9867, #13113, #10228, #15628, #17410, #7262, #5789, #425, #2839, #8842, #12921, #233, #5880, #11623, #1451, #7357, #9954, #11529, #11346, #17036, #14520, #4306, #8745, #17123, #8652, #2927, #4493, #8563, #12835, #138, #4401, #10135, #3113, #14236, #7175, #10042, #15719, #15815, #13019, #332, #17508, #6684, #15239, #10422, #13828, #7730, #7546, #12432, #10951, #13390, #4769, #10514, #3813, #16183, #10324, #5300, #2009, #16635, #2534, #17601, #16102, #11904, #3479, #16536, #9125, #3392, #18025, #7636, #8164, #1045, #703, #2445, #14803, #13301, #517, #2102, #5207, #14617, #6599, #8938, #12246, #13201, #613, #1137, #11810, #17934, #10858, #1919, #12337, #9467, #3908, #4675, #9560, #6161, #6774, #15139, #8076, #9032, #13735, #14710, #6253, #4864, #16005, #3297, #2886, #8431, #14008, #12701, #4353, #5567, #16996, #11216, #5392, #98, #15420, #5753, #15681, #12610, #5482, #7038, #18299, #11303, #16905, #16814, #12793, #2715, #10003, #14192, #2802, #15584, #4180, #8350, #13923, #9826, #8, #9644, #15506, #4000, #14098, #9738, #1410, #8606, #6866, #5659, #4270, #15323, #1495, #9913, #7130, #7222, #11390, #8264, #2976, #8518, #17081, #18214, #14285, #12522, #2623, #1588, #18123, #11042, #1232, #11128, #16725, #4084, #1320, #6954, #11577, #14477, #2059, #4728, #3159, #10377, #8995, #10088, #4630, #15862, #14670, #12878, #10279, #185, #5835, #3349, #17556, #17178, #17271, #383, #14571, #17365, #8894, #13160, #4826, #11482, #4451, #6021, #15768, #571, #11672, #14761, #16056, #3067, #6213, #1779, #15961, #8700, #14374, #7409, #5930, #3255, #470, #1873, #3441, #4543, #1676, #11765, #13067, #7504, #10185, #6114, #8796, #17459, #7311, #1967, #12971, #7593, #13252, #287, #11861, #10473, #16150, #9081, #6484, #17738, #5089, #6665, #15118, #13713, #12043, #8051, #932, #843, #9444, #15214, #2422, #16238, #18005, #12133, #17826, #7783, #6574, #14856, #10562, #12315, #2332, #1025, #10930, #11958, #13440, #17913, #661, #3530, #17651, #15028, #5276, #16613, #3886, #12226, #5001, #9535, #5182, #7690, #13351, #4910, #10749, #3791, #6308, #9177, #16512, #2151, #753, #6398, #16422, #3616, #10658, #16329, #9266, #3704, #9352 ),
 .UNSPECIFIED., .F., .F. ) 
 B_SPLINE_CURVE_WITH_KNOTS ( ( 3, 2, 2, 2, 2, 2, 2, 2, 2, 2, 2, 2, 2, 2, 2, 2, 2, 2, 2, 2, 2, 2, 2, 2, 2, 2, 2, 2, 2, 2, 2, 2, 2, 2, 2, 2, 2, 2, 2, 2, 2, 2, 2, 2, 2, 2, 2, 2, 2, 2, 2, 2, 2, 2, 2, 2, 2, 2, 2, 2, 2, 2, 2, 2, 2, 2, 2, 2, 2, 2, 2, 2, 2, 2, 2, 2, 2, 2, 2, 2, 2, 2, 2, 2, 2, 2, 2, 2, 2, 2, 2, 2, 2, 2, 2, 2, 2, 2, 2, 2, 2, 2, 2, 2, 2, 2, 2, 2, 2, 2, 2, 2, 2, 2, 2, 2, 2, 2, 2, 2, 2, 2, 2, 2, 2, 2, 2, 2, 2, 2, 2, 2, 2, 2, 2, 2, 2, 2, 2, 2, 2, 2, 2, 2, 2, 2, 2, 2, 2, 2, 2, 2, 2, 2, 2, 2, 2, 2, 2, 2, 2, 2, 2, 2, 2, 2, 2, 2, 2, 2, 2, 2, 2, 2, 3 ),
 ( 0.000000000000000000, 0.005769117253040331565, 0.01153823450608066313, 0.01730735175912099383, 0.02307646901216132626, 0.02884558626520165869, 0.03461470351824198766, 0.04038382077128232356, 0.04615293802432265252, 0.05192205527736298148, 0.05769117253040331739, 0.06346028978344366023, 0.06922940703648397531, 0.07499852428952431815, 0.08076764154256464712, 0.08653675879560497608, 0.09230587604864530504, 0.09807499330168564788, 0.1038441105547259630, 0.1096132278077663058, 0.1153823450608066348, 0.1211514623138469637, 0.1269205795668873205, 0.1326896968199276217, 0.1384588140729679506, 0.1442279313260082796, 0.1499970485790486363, 0.1557661658320889653, 0.1615352830851292942, 0.1673044003381695954, 0.1730735175912099522, 0.1788426348442502811, 0.1846117520972906101, 0.1903808693503309390, 0.1961499866033712958, 0.2019191038564116247, 0.2076882211094519259, 0.2134573383624922549, 0.2192264556155326116, 0.2249955728685729406, 0.2307646901216132695, 0.2365338073746535985, 0.2423029246276939275, 0.2480720418807342564, 0.2538411591337746409, 0.2596102763868149421, 0.2653793936398552433, 0.2711485108928956000, 0.2769176281459359013, 0.2826867453989762580, 0.2884558626520165592, 0.2942249799050568604, 0.2999940971580972726, 0.3057632144111375738, 0.3115323316641779305, 0.3173014489172182317, 0.3230705661702585885, 0.3288396834232988897, 0.3346088006763391909, 0.3403779179293795476, 0.3461470351824199043, 0.3519161524354602610, 0.3576852696885005622, 0.3634543869415409190, 0.3692235041945812202, 0.3749926214476215214, 0.3807617387006618781, 0.3865308559537021793, 0.3922999732067425915, 0.3980690904597828927, 0.4038382077128232495, 0.4096073249658635507, 0.4153764422189038519, 0.4211455594719442086, 0.4269146767249845098, 0.4326837939780248665, 0.4384529112310652232, 0.4442220284841055244, 0.4499911457371458812, 0.4557602629901861824, 0.4615293802432265391, 0.4672984974962668403, 0.4730676147493071970, 0.4788367320023474982, 0.4846058492553878549, 0.4903749665084282117, 0.4961440837614685129, 0.5019132010145088696, 0.5076823182675492818, 0.5134514355205894720, 0.5192205527736298842, 0.5249896700266701854, 0.5307587872797104867, 0.5365279045327507879, 0.5422970217857912001, 0.5480661390388316123, 0.5538352562918718025, 0.5596043735449122147, 0.5653734907979525159, 0.5711426080509928171, 0.5769117253040331184, 0.5826808425570735306, 0.5884499598101137208, 0.5942190770631541330, 0.5999881943161945452, 0.6057573115692348464, 0.6115264288222751476, 0.6172955460753154489, 0.6230646633283558611, 0.6288337805813960513, 0.6346028978344364635, 0.6403720150874768757, 0.6461411323405171769, 0.6519102495935574781, 0.6576793668465977794, 0.6634484840996381916, 0.6692176013526783818, 0.6749867186057187940, 0.6807558358587590952, 0.6865249531117995074, 0.6922940703648398086, 0.6980631876178801098, 0.7038323048709205221, 0.7096014221239607123, 0.7153705393770011245, 0.7211396566300414257, 0.7269087738830818379, 0.7326778911361221391, 0.7384470083891624403, 0.7442161256422028526, 0.7499852428952430428, 0.7557543601482834550, 0.7615234774013237562, 0.7672925946543641684, 0.7730617119074043586, 0.7788308291604447708, 0.7845999464134851831, 0.7903690636665253733, 0.7961381809195657855, 0.8019072981726060867, 0.8076764154256464989, 0.8134455326786866891, 0.8192146499317271013, 0.8249837671847675136, 0.8307528844378077038, 0.8365220016908481160, 0.8422911189438884172, 0.8480602361969287184, 0.8538293534499690196, 0.8595984707030094318, 0.8653675879560497330, 0.8711367052090900343, 0.8769058224621304465, 0.8826749397151707477, 0.8884440569682110489, 0.8942131742212513501, 0.8999822914742917623, 0.9057514087273320635, 0.9115205259803723647, 0.9172896432334127770, 0.9230587604864530782, 0.9288278777394933794, 0.9345969949925336806, 0.9403661122455740928, 0.9461352294986143940, 0.9519043467516546952, 0.9576734640046949965, 0.9634425812577354087, 0.9692116985107757099, 0.9749808157638160111, 0.9807499330168564233, 0.9865190502698967245, 0.9922881675229370257, 0.9980572847759773270, 1.000000000000000000 ),
 .UNSPECIFIED. ) 
 CURVE ( )  GEOMETRIC_REPRESENTATION_ITEM ( )  RATIONAL_B_SPLINE_CURVE ( ( 1.000000000000000000, 0.8660254037844387076, 1.000000000000000000, 0.8660254037844387076, 1.000000000000000000, 0.8660254037844387076, 1.000000000000000000, 0.8660254037844387076, 1.000000000000000000, 0.8660254037844387076, 1.000000000000000000, 0.8660254037844387076, 1.000000000000000000, 0.8660254037844387076, 1.000000000000000000, 0.8660254037844387076, 1.000000000000000000, 0.8660254037844387076, 1.000000000000000000, 0.8660254037844387076, 1.000000000000000000, 0.8660254037844387076, 1.000000000000000000, 0.8660254037844387076, 1.000000000000000000, 0.8660254037844387076, 1.000000000000000000, 0.8660254037844387076, 1.000000000000000000, 0.8660254037844387076, 1.000000000000000000, 0.8660254037844387076, 1.000000000000000000, 0.8660254037844387076, 1.000000000000000000, 0.8660254037844387076, 1.000000000000000000, 0.8660254037844387076, 1.000000000000000000, 0.8660254037844387076, 1.000000000000000000, 0.8660254037844387076, 1.000000000000000000, 0.8660254037844387076, 1.000000000000000000, 0.8660254037844387076, 1.000000000000000000, 0.8660254037844387076, 1.000000000000000000, 0.8660254037844387076, 1.000000000000000000, 0.8660254037844387076, 1.000000000000000000, 0.8660254037844387076, 1.000000000000000000, 0.8660254037844387076, 1.000000000000000000, 0.8660254037844387076, 1.000000000000000000, 0.8660254037844387076, 1.000000000000000000, 0.8660254037844387076, 1.000000000000000000, 0.8660254037844387076, 1.000000000000000000, 0.8660254037844387076, 1.000000000000000000, 0.8660254037844387076, 1.000000000000000000, 0.8660254037844387076, 1.000000000000000000, 0.8660254037844387076, 1.000000000000000000, 0.8660254037844387076, 1.000000000000000000, 0.8660254037844387076, 1.000000000000000000, 0.8660254037844387076, 1.000000000000000000, 0.8660254037844387076, 1.000000000000000000, 0.8660254037844387076, 1.000000000000000000, 0.8660254037844387076, 1.000000000000000000, 0.8660254037844387076, 1.000000000000000000, 0.8660254037844387076, 1.000000000000000000, 0.8660254037844387076, 1.000000000000000000, 0.8660254037844387076, 1.000000000000000000, 0.8660254037844387076, 1.000000000000000000, 0.8660254037844387076, 1.000000000000000000, 0.8660254037844387076, 1.000000000000000000, 0.8660254037844387076, 1.000000000000000000, 0.8660254037844387076, 1.000000000000000000, 0.8660254037844387076, 1.000000000000000000, 0.8660254037844387076, 1.000000000000000000, 0.8660254037844387076, 1.000000000000000000, 0.8660254037844387076, 1.000000000000000000, 0.8660254037844387076, 1.000000000000000000, 0.8660254037844387076, 1.000000000000000000, 0.8660254037844387076, 1.000000000000000000, 0.8660254037844387076, 1.000000000000000000, 0.8660254037844387076, 1.000000000000000000, 0.8660254037844387076, 1.000000000000000000, 0.8660254037844387076, 1.000000000000000000, 0.8660254037844387076, 1.000000000000000000, 0.8660254037844387076, 1.000000000000000000, 0.8660254037844387076, 1.000000000000000000, 0.8660254037844387076, 1.000000000000000000, 0.8660254037844387076, 1.000000000000000000, 0.8660254037844387076, 1.000000000000000000, 0.8660254037844387076, 1.000000000000000000, 0.8660254037844387076, 1.000000000000000000, 0.8660254037844387076, 1.000000000000000000, 0.8660254037844387076, 1.000000000000000000, 0.8660254037844387076, 1.000000000000000000, 0.8660254037844387076, 1.000000000000000000, 0.8660254037844387076, 1.000000000000000000, 0.8660254037844387076, 1.000000000000000000, 0.8660254037844387076, 1.000000000000000000, 0.8660254037844387076, 1.000000000000000000, 0.8660254037844387076, 1.000000000000000000, 0.8660254037844387076, 1.000000000000000000, 0.8660254037844387076, 1.000000000000000000, 0.8660254037844387076, 1.000000000000000000, 0.8660254037844387076, 1.000000000000000000, 0.8660254037844387076, 1.000000000000000000, 0.8660254037844387076, 1.000000000000000000, 0.8660254037844387076, 1.000000000000000000, 0.8660254037844387076, 1.000000000000000000, 0.8660254037844387076, 1.000000000000000000, 0.8660254037844387076, 1.000000000000000000, 0.8660254037844387076, 1.000000000000000000, 0.8660254037844387076, 1.000000000000000000, 0.8660254037844387076, 1.000000000000000000, 0.8660254037844387076, 1.000000000000000000, 0.8660254037844387076, 1.000000000000000000, 0.8660254037844387076, 1.000000000000000000, 0.8660254037844387076, 1.000000000000000000, 0.8660254037844387076, 1.000000000000000000, 0.8660254037844387076, 1.000000000000000000, 0.8660254037844387076, 1.000000000000000000, 0.8660254037844387076, 1.000000000000000000, 0.8660254037844387076, 1.000000000000000000, 0.8660254037844387076, 1.000000000000000000, 0.8660254037844387076, 1.000000000000000000, 0.8660254037844387076, 1.000000000000000000, 0.8660254037844387076, 1.000000000000000000, 0.8660254037844387076, 1.000000000000000000, 0.8660254037844387076, 1.000000000000000000, 0.8660254037844387076, 1.000000000000000000, 0.8660254037844387076, 1.000000000000000000, 0.8660254037844387076, 1.000000000000000000, 0.8660254037844387076, 1.000000000000000000, 0.8660254037844387076, 1.000000000000000000, 0.8660254037844387076, 1.000000000000000000, 0.8660254037844387076, 1.000000000000000000, 0.8660254037844387076, 1.000000000000000000, 0.8660254037844387076, 1.000000000000000000, 0.8660254037844387076, 1.000000000000000000, 0.8660254037844387076, 1.000000000000000000, 0.8660254037844387076, 1.000000000000000000, 0.8660254037844387076, 1.000000000000000000, 0.8660254037844387076, 1.000000000000000000, 0.8660254037844387076, 1.000000000000000000, 0.8660254037844387076, 1.000000000000000000, 0.8660254037844387076, 1.000000000000000000, 0.8660254037844387076, 1.000000000000000000, 0.8660254037844387076, 1.000000000000000000, 0.8660254037844387076, 1.000000000000000000, 0.8660254037844387076, 1.000000000000000000, 0.8660254037844387076, 1.000000000000000000, 0.8660254037844387076, 1.000000000000000000, 0.8660254037844387076, 1.000000000000000000, 0.8660254037844387076, 1.000000000000000000, 0.8660254037844387076, 1.000000000000000000, 0.8660254037844387076, 1.000000000000000000, 0.8660254037844387076, 1.000000000000000000, 0.8660254037844387076, 1.000000000000000000, 0.8660254037844387076, 1.000000000000000000, 0.8660254037844387076, 1.000000000000000000, 0.8660254037844387076, 1.000000000000000000, 0.8660254037844387076, 1.000000000000000000, 0.8660254037844387076, 1.000000000000000000, 0.8660254037844387076, 1.000000000000000000, 0.8660254037844387076, 1.000000000000000000, 0.8660254037844387076, 1.000000000000000000, 0.8660254037844387076, 1.000000000000000000, 0.8660254037844387076, 1.000000000000000000, 0.8660254037844387076, 1.000000000000000000, 0.8660254037844387076, 1.000000000000000000, 0.8660254037844387076, 1.000000000000000000, 0.8660254037844387076, 1.000000000000000000, 0.8660254037844387076, 1.000000000000000000, 0.8660254037844387076, 1.000000000000000000, 0.8660254037844387076, 1.000000000000000000, 0.8660254037844387076, 1.000000000000000000, 0.8660254037844387076, 1.000000000000000000, 0.8660254037844387076, 1.000000000000000000, 0.8660254037844387076, 1.000000000000000000, 0.8660254037844387076, 1.000000000000000000, 0.8660254037844387076, 1.000000000000000000, 0.8660254037844387076, 1.000000000000000000, 0.8660254037844387076, 1.000000000000000000, 0.8660254037844387076, 1.000000000000000000, 0.8660254037844387076, 1.000000000000000000, 0.8660254037844387076, 1.000000000000000000, 0.8660254037844387076, 1.000000000000000000, 0.8660254037844387076, 1.000000000000000000, 0.8660254037844387076, 1.000000000000000000, 0.8660254037844387076, 1.000000000000000000, 0.8660254037844387076, 1.000000000000000000, 0.8660254037844387076, 1.000000000000000000, 0.8660254037844387076, 1.000000000000000000, 0.8660254037844387076, 1.000000000000000000, 0.8660254037844387076, 1.000000000000000000, 0.9548848677736452295, 0.9401542295229485813 ) ) 
 REPRESENTATION_ITEM ( '' )  );
#2353=CARTESIAN_POINT ( 'NONE',  ( -2.121784821874996396, -16.80311853779403108, -6.123095346843099307 ) ) ;
#2364=ORIENTED_EDGE ( 'NONE', *, *, #5369, .F. ) ;
#2367=CARTESIAN_POINT ( 'NONE',  ( -2.121784821875005722, -27.86783793146007326, -9.110681959144070419 ) ) ;
#2374=CARTESIAN_POINT ( 'NONE',  ( 4.243569643750003451, -23.54952454117618288, -13.62221657742576397 ) ) ;
#2379=CARTESIAN_POINT ( 'NONE',  ( 4.243569643749996345, -23.44441649529964877, -4.929126507931827383 ) ) ;
#2380=CARTESIAN_POINT ( 'NONE',  ( -1.071796769724505882, -18.75697028620200868, -9.480036841823904936 ) ) ;
#2381=FACE_OUTER_BOUND ( 'NONE', #14338, .T. ) ;
#2384=CARTESIAN_POINT ( 'NONE',  ( 1.071796769724494780, -26.72978832048277553, -6.918826660630844394 ) ) ;
#2388=CARTESIAN_POINT ( 'NONE',  ( -2.465190328815646976E-33, -26.97786251599082519, -14.24690051095425858 ) ) ;
#2389=ORIENTED_EDGE ( 'NONE', *, *, #4375, .F. ) ;
#2390=CARTESIAN_POINT ( 'NONE',  ( -4.243569643750000786, -21.31917248646755070, -6.165453624519022569 ) ) ;
#2393=ORIENTED_EDGE ( 'NONE', *, *, #15984, .F. ) ;
#2394=CARTESIAN_POINT ( 'NONE',  ( 1.999999999999994449, -24.66763991940512568, -4.908083853891920256 ) ) ;
#2396=CARTESIAN_POINT ( 'NONE',  ( 2.446180570232387108, -24.42336006072196142, -16.36676630457531445 ) ) ;
#2397=CARTESIAN_POINT ( 'NONE',  ( 7.315923705238545516, -13.46616490046861792, 2.115434428656500998 ) ) ;
#2399=CARTESIAN_POINT ( 'NONE',  ( -4.243569643750000786, -25.93287794636623644, -12.75450788076862452 ) ) ;
#2401=CARTESIAN_POINT ( 'NONE',  ( 2.000000000000004441, -20.26142594620695192, -10.69431187202529010 ) ) ;
#2402=CARTESIAN_POINT ( 'NONE',  ( 1.999999999999994449, -24.73216726919956443, -5.000238459881198416 ) ) ;
#2405=ORIENTED_EDGE ( 'NONE', *, *, #16786, .T. ) ;
#2407=CARTESIAN_POINT ( 'NONE',  ( 1.071796769724504328, -25.69735073505090384, -5.444352980910657003 ) ) ;
#2414=CARTESIAN_POINT ( 'NONE',  ( 4.713407268011036227E-15, -17.42274839898859895, -8.653419144721045342 ) ) ;
#2422=CARTESIAN_POINT ( 'NONE',  ( -2.121784821874996396, -17.54518305232318554, -7.182873304141986992 ) ) ;
#2423=CARTESIAN_POINT ( 'NONE',  ( -4.243569643750000786, -23.90026645004723704, -9.851637823819498152 ) ) ;
#2424=EDGE_CURVE ( 'NONE', #18219, #6378, #14862, .T. ) ;
#2426=EDGE_LOOP ( 'NONE', ( #5914, #12294, #16787, #1295 ) ) ;
#2428=CARTESIAN_POINT ( 'NONE',  ( -8.999999999999996447, -10.00000000000000000, -3.713574246709372417 ) ) ;
#2430=CARTESIAN_POINT ( 'NONE',  ( 9.184850993605147944E-16, -33.35093342269870931, -10.27273805603704737 ) ) ;
#2435=CARTESIAN_POINT ( 'NONE',  ( -2.121784821875005722, -22.96375940065866672, -2.106931980473163879 ) ) ;
#2438=CARTESIAN_POINT ( 'NONE',  ( 4.000000000000003553, -22.45483000112048799, -11.81365854749089017 ) ) ;
#2440=CARTESIAN_POINT ( 'NONE',  ( 4.243569643750003451, -17.87111782130087434, -5.512611338964712893 ) ) ;
#2441=EDGE_CURVE ( 'NONE', #15144, #8682, #6404, .T. ) ;
#2445=CARTESIAN_POINT ( 'NONE',  ( 4.243569643749997233, -26.28361985523730837, -8.983929127162353367 ) ) ;
#2446=CARTESIAN_POINT ( 'NONE',  ( -4.000000000000000888, -20.62550348340303685, -5.174791620453635943 ) ) ;
#2448=CARTESIAN_POINT ( 'NONE',  ( 0.000000000000000000, 5.977523610840987267, 32.81826849749789687 ) ) ;
#2455=CARTESIAN_POINT ( 'NONE',  ( 1.999999999999994449, -26.99062448662684943, -8.225649633262349880 ) ) ;
#2458=CARTESIAN_POINT ( 'NONE',  ( 2.121784821874994176, -27.30860090601781209, -8.312008715962296179 ) ) ;
#2460=( BOUNDED_CURVE ( )  B_SPLINE_CURVE ( 2, ( #7648, #530, #6266, #11919, #17616, #16295, #11728, #16200, #6177 ),
 .UNSPECIFIED., .F., .F. ) 
 B_SPLINE_CURVE_WITH_KNOTS ( ( 3, 2, 2, 2, 3 ),
 ( 0.8879310344827586743, 0.8908045977011493921, 0.8965517241379310498, 0.9022988505747125965, 0.9051724137931034253 ),
 .UNSPECIFIED. ) 
 CURVE ( )  GEOMETRIC_REPRESENTATION_ITEM ( )  RATIONAL_B_SPLINE_CURVE ( ( 0.9330127018922194093, 0.9330127018922206306, 1.000000000000000000, 0.8660254037844387076, 1.000000000000000000, 0.8660254037844387076, 1.000000000000000000, 0.9330127018922194093, 0.9330127018922194093 ) ) 
 REPRESENTATION_ITEM ( '' )  );
#2464=CYLINDRICAL_SURFACE ( 'NONE', #16413, 4.000000000000000000 ) ;
#2466=CARTESIAN_POINT ( 'NONE',  ( 4.243569643749996345, -26.05777413342408622, -8.661388009723561154 ) ) ;
#2471=CARTESIAN_POINT ( 'NONE',  ( 4.243569643750000786, -22.44840109553366858, -7.778159211712977417 ) ) ;
#2473=CARTESIAN_POINT ( 'NONE',  ( -4.648177544792955347E-16, -30.03220982406077155, -11.63517334838810058 ) ) ;
#2476=CARTESIAN_POINT ( 'NONE',  ( 4.299564228933482956E-15, -16.63909446626264454, -6.455396711050170211 ) ) ;
#2482=CARTESIAN_POINT ( 'NONE',  ( -4.243569643750004339, -22.78838844622314497, -3.992221357276295901 ) ) ;
#2486=ADVANCED_FACE ( 'NONE', ( #18108 ), #12506, .F. ) ;
#2493=CARTESIAN_POINT ( 'NONE',  ( -5.330712181944245322E-15, -29.62412893858816076, -9.483180404412477671 ) ) ;
#2496=CARTESIAN_POINT ( 'NONE',  ( 4.713407268011036227E-15, -18.26160393785694325, -9.851429010500462269 ) ) ;
#2499=ORIENTED_EDGE ( 'NONE', *, *, #9322, .F. ) ;
#2507=CARTESIAN_POINT ( 'NONE',  ( -4.243569643750000786, -25.44892282819504459, -12.06334834339978634 ) ) ;
#2510=CARTESIAN_POINT ( 'NONE',  ( -4.000000000000004441, -21.97952618743386566, -3.082218539220304976 ) ) ;
#2512=LINE ( 'NONE', #8140, #4717 ) ;
#2514=DIRECTION ( 'NONE',  ( -0.000000000000000000, -0.000000000000000000, 1.000000000000000000 ) ) ;
#2516=CARTESIAN_POINT ( 'NONE',  ( 4.243569643750003451, -20.45221178488055713, -9.198795538265191141 ) ) ;
#2517=CARTESIAN_POINT ( 'NONE',  ( -3.291771655530798757, -28.93493258167780269, -13.02337503524261386 ) ) ;
#2518=VERTEX_POINT ( 'NONE', #2249 ) ;
#2519=CARTESIAN_POINT ( 'NONE',  ( -4.000000000000000888, -25.07789057128293919, -11.53345936525372650 ) ) ;
#2521=DIRECTION ( 'NONE',  ( 0.000000000000000000, 1.000000000000000000, 0.000000000000000000 ) ) ;
#2525=CARTESIAN_POINT ( 'NONE',  ( 4.243569643749996345, -22.67008830622574322, -3.823271248141685508 ) ) ;
#2527=EDGE_CURVE ( 'NONE', #17673, #13336, #2193, .T. ) ;
#2529=CARTESIAN_POINT ( 'NONE',  ( -2.000000000000005773, -27.29175211571113735, -8.655704456514076384 ) ) ;
#2531=CARTESIAN_POINT ( 'NONE',  ( -4.243569643750005227, -21.75595086079126261, -2.517747677556105845 ) ) ;
#2534=CARTESIAN_POINT ( 'NONE',  ( 2.121784821874994176, -27.56671030237578179, -8.680627135892345692 ) ) ;
#2542=EDGE_CURVE ( 'NONE', #9873, #8670, #16620, .T. ) ;
#2543=CARTESIAN_POINT ( 'NONE',  ( -1.661723472263481630E-14, -21.28506360070608139, -13.09052826979102946 ) ) ;
#2544=DIRECTION ( 'NONE',  ( -0.000000000000000000, -0.5735764363510414965, -0.8191520442889950182 ) ) ;
#2548=CARTESIAN_POINT ( 'NONE',  ( -2.121784821874996396, -21.41682399769271328, -12.71214960309270303 ) ) ;
#2554=CARTESIAN_POINT ( 'NONE',  ( -4.243569643749997233, -22.68915988664961247, -12.39348851099227389 ) ) ;
#2555=CARTESIAN_POINT ( 'NONE',  ( 0.000000000000000000, -15.45745613286698550, -10.86990606519495195 ) ) ;
#2557=CARTESIAN_POINT ( 'NONE',  ( -3.999999999999997335, -18.81978933645070029, -6.622282467816152263 ) ) ;
#2558=DIRECTION ( 'NONE',  ( 0.000000000000000000, 0.000000000000000000, 1.000000000000000000 ) ) ;
#2559=( BOUNDED_CURVE ( )  B_SPLINE_CURVE ( 2, ( #5335, #1170, #5146, #2658, #3851, #7923, #803, #12279, #10804 ),
 .UNSPECIFIED., .F., .F. ) 
 B_SPLINE_CURVE_WITH_KNOTS ( ( 3, 2, 2, 2, 3 ),
 ( 0.9396551724137931494, 0.9425287356321838672, 0.9482758620689655249, 0.9540229885057470716, 0.9568965517241379004 ),
 .UNSPECIFIED. ) 
 CURVE ( )  GEOMETRIC_REPRESENTATION_ITEM ( )  RATIONAL_B_SPLINE_CURVE ( ( 0.9330127018922194093, 0.9330127018922206306, 1.000000000000000000, 0.8660254037844387076, 1.000000000000000000, 0.8660254037844387076, 1.000000000000000000, 0.9330127018922194093, 0.9330127018922194093 ) ) 
 REPRESENTATION_ITEM ( '' )  );
#2560=CARTESIAN_POINT ( 'NONE',  ( -2.121784821874996396, -18.83573003411303048, -9.025965403792225672 ) ) ;
#2562=CARTESIAN_POINT ( 'NONE',  ( 0.000000000000000000, 9.254131787996968228, 30.52396275209373044 ) ) ;
#2568=CARTESIAN_POINT ( 'NONE',  ( 0.000000000000000000, -3.999999999999991562, 11.59510085796834566 ) ) ;
#2572=CARTESIAN_POINT ( 'NONE',  ( -4.243569643749998122, -19.33373773399602058, -7.601449051901652432 ) ) ;
#2574=CYLINDRICAL_SURFACE ( 'NONE', #6163, 4.000000000000000000 ) ;
#2576=CARTESIAN_POINT ( 'NONE',  ( -4.243569643750004339, -28.43453149155370241, -12.05574929324608924 ) ) ;
#2578=DIRECTION ( 'NONE',  ( -0.000000000000000000, -0.000000000000000000, 1.000000000000000000 ) ) ;
#2580=CARTESIAN_POINT ( 'NONE',  ( -4.243569643750005227, -28.17642209519573271, -11.68713087331604150 ) ) ;
#2581=EDGE_LOOP ( 'NONE', ( #12518, #916, #2405, #9613 ) ) ;
#2583=CARTESIAN_POINT ( 'NONE',  ( 2.000000000000004441, -19.48709775713304637, -9.588456612235146892 ) ) ;
#2586=CARTESIAN_POINT ( 'NONE',  ( -4.000000000000007105, 6.938893903907228378E-15, 30.00000000000000000 ) ) ;
#2587=EDGE_CURVE ( 'NONE', #15966, #16586, #14040, .T. ) ;
#2592=EDGE_CURVE ( 'NONE', #2690, #12581, #2831, .T. ) ;
#2593=ORIENTED_EDGE ( 'NONE', *, *, #17161, .T. ) ;
#2594=CARTESIAN_POINT ( 'NONE',  ( -4.243569643750004339, -28.20868576974048025, -11.73320817580729525 ) ) ;
#2596=CARTESIAN_POINT ( 'NONE',  ( 2.000000000000004441, -18.39013282190673237, -8.021828326525680453 ) ) ;
#2599=CARTESIAN_POINT ( 'NONE',  ( -4.000000000000004441, -25.91569448259783215, -8.703649444160298287 ) ) ;
#2600=CYLINDRICAL_SURFACE ( 'NONE', #15004, 4.000000000000000000 ) ;
#2601=DIRECTION ( 'NONE',  ( 1.000000000000000000, 0.000000000000000000, 0.000000000000000000 ) ) ;
#2602=CARTESIAN_POINT ( 'NONE',  ( 2.121784821875004390, -19.42723073410004986, -9.870715949465248329 ) ) ;
#2604=CARTESIAN_POINT ( 'NONE',  ( -1.661723472263481630E-14, -20.05904396871067874, -11.33959077613006450 ) ) ;
#2605=ORIENTED_EDGE ( 'NONE', *, *, #17223, .T. ) ;
#2606=CARTESIAN_POINT ( 'NONE',  ( 3.999999999999996447, -26.34587680986112090, -9.318013477377038001 ) ) ;
#2607=DIRECTION ( 'NONE',  ( -0.000000000000000000, -0.5735764363510414965, -0.8191520442889950182 ) ) ;
#2608=DIRECTION ( 'NONE',  ( -1.000000000000000000, 8.673617379884035472E-16, 0.000000000000000000 ) ) ;
#2614=CARTESIAN_POINT ( 'NONE',  ( 4.730628863548789710E-15, -16.30511083791103744, -7.547611698733671659 ) ) ;
#2618=CARTESIAN_POINT ( 'NONE',  ( -5.279047395330986450E-15, -28.99044649497685455, -9.068532494787179488 ) ) ;
#2620=CARTESIAN_POINT ( 'NONE',  ( -2.000000000000005773, -28.38871705093744779, -10.22233274222354460 ) ) ;
#2622=FACE_OUTER_BOUND ( 'NONE', #8437, .T. ) ;
#2623=CARTESIAN_POINT ( 'NONE',  ( 2.121784821875004390, -19.39496705955529876, -9.824638646973991030 ) ) ;
#2626=CARTESIAN_POINT ( 'NONE',  ( 8.500000000000019540, 10.00000000000000000, 18.49999999999998934 ) ) ;
#2634=ORIENTED_EDGE ( 'NONE', *, *, #5808, .F. ) ;
#2636=CARTESIAN_POINT ( 'NONE',  ( -2.121784821875005722, -27.09350974238616416, -8.004826699353927211 ) ) ;
#2639=CARTESIAN_POINT ( 'NONE',  ( -5.577813053751546416E-15, -25.64435008597530796, -5.368660209577289955 ) ) ;
#2642=CARTESIAN_POINT ( 'NONE',  ( -5.330712181944245322E-15, -27.59151744226915781, -6.580310347463352194 ) ) ;
#2644=EDGE_CURVE ( 'NONE', #10757, #6383, #10125, .T. ) ;
#2646=CARTESIAN_POINT ( 'NONE',  ( 0.000000000000000000, 9.254131787996968228, 30.52396275209373044 ) ) ;
#2647=EDGE_CURVE ( 'NONE', #11633, #14859, #17210, .T. ) ;
#2648=CARTESIAN_POINT ( 'NONE',  ( 9.000000000000003553, -4.000000000000000000, 30.00000000000000000 ) ) ;
#2649=VECTOR ( 'NONE', #13207, 999.9999999999998863 ) ;
#2650=CARTESIAN_POINT ( 'NONE',  ( -4.243569643750000786, -22.06123700099670870, -7.225231581817909365 ) ) ;
#2656=CARTESIAN_POINT ( 'NONE',  ( 1.999999999999994449, -26.28082364734737908, -7.211948979461484832 ) ) ;
#2658=CARTESIAN_POINT ( 'NONE',  ( -3.999999999999997335, -18.23904319394032569, -5.792891021966779519 ) ) ;
#2663=CARTESIAN_POINT ( 'NONE',  ( 4.243569643750003451, -19.67788359580665869, -8.092940278475046156 ) ) ;
#2666=DIRECTION ( 'NONE',  ( -0.000000000000000000, 1.000000000000000000, -0.000000000000000000 ) ) ;
#2668=CARTESIAN_POINT ( 'NONE',  ( -5.330712181944246111E-15, -30.39845712766207697, -10.58903566420262088 ) ) ;
#2672=CARTESIAN_POINT ( 'NONE',  ( 4.730628863548789710E-15, -22.49973635050228538, -16.39445377705482088 ) ) ;
#2673=EDGE_LOOP ( 'NONE', ( #3283, #7736, #15748, #15408, #4894, #14015, #8873, #17450, #432, #16336, #463, #11979, #6964, #11277, #4568, #2179, #2848, #5279, #12708, #1226, #2593, #9073, #15890, #4055, #12737, #421, #6870, #8259, #3891, #1864, #2605, #9159, #18245, #5070, #8599, #15145, #15010, #17984, #6949, #12616, #15685, #7296, #18358, #10543, #12560, #3536, #15425, #2017, #12591, #536, #18329, #15390, #5361, #4209, #17207, #5938, #2813, #15488, #8213, #312, #15772, #5990, #11315, #6824 ) ) ;
#2675=CARTESIAN_POINT ( 'NONE',  ( 4.713407268011036227E-15, -17.74538514514100740, -9.114192170640368573 ) ) ;
#2678=CARTESIAN_POINT ( 'NONE',  ( 1.071796769724495224, -19.03813308399763571, -9.881578931065789106 ) ) ;
#2683=CARTESIAN_POINT ( 'NONE',  ( -8.500000000000005329, 10.00000000000000000, -20.49999999999999645 ) ) ;
#2686=CARTESIAN_POINT ( 'NONE',  ( 2.121784821875004390, -22.78265288675364175, -14.66275540855586890 ) ) ;
#2689=CARTESIAN_POINT ( 'NONE',  ( 4.730628863548789710E-15, -23.04821881776296877, -17.17776791940616832 ) ) ;
#2690=VERTEX_POINT ( 'NONE', #8733 ) ;
#2692=CARTESIAN_POINT ( 'NONE',  ( 4.898587196589413815E-16, 2.700915433685006750, 35.11257424290206330 ) ) ;
#2695=DIRECTION ( 'NONE',  ( 0.000000000000000000, 0.000000000000000000, 1.000000000000000000 ) ) ;
#2696=CARTESIAN_POINT ( 'NONE',  ( 2.121784821874994176, -25.79220820241474854, -6.146375498873266174 ) ) ;
#2697=ORIENTED_EDGE ( 'NONE', *, *, #11288, .T. ) ;
#2700=CARTESIAN_POINT ( 'NONE',  ( -3.999999999999997335, -22.94953967817820129, -12.52017718669691604 ) ) ;
#2701=CARTESIAN_POINT ( 'NONE',  ( -5.000000000000001776, 0.000000000000000000, 5.000000000000000888 ) ) ;
#2702=DIRECTION ( 'NONE',  ( 0.000000000000000000, 0.000000000000000000, 1.000000000000000000 ) ) ;
#2703=ORIENTED_EDGE ( 'NONE', *, *, #3889, .F. ) ;
#2706=CARTESIAN_POINT ( 'NONE',  ( 4.713407268011036227E-15, -22.13324488322647454, -15.38070530945117831 ) ) ;
#2710=CARTESIAN_POINT ( 'NONE',  ( 3.999999999999996447, -26.79756825278262511, -9.963095711247856201 ) ) ;
#2713=CARTESIAN_POINT ( 'NONE',  ( 4.299564228933482956E-15, -22.38202853593239183, -14.65715655550049590 ) ) ;
#2715=CARTESIAN_POINT ( 'NONE',  ( -4.243569643749998122, -21.10823983395705383, -10.13570068892073195 ) ) ;
#2722=ORIENTED_EDGE ( 'NONE', *, *, #14043, .T. ) ;
#2725=CARTESIAN_POINT ( 'NONE',  ( 4.299564228933482956E-15, -18.70396963712639504, -9.404344070490550322 ) ) ;
#2728=EDGE_LOOP ( 'NONE', ( #10209, #9209, #13408, #619 ) ) ;
#2730=CARTESIAN_POINT ( 'NONE',  ( -4.243569643750005227, -24.56289054618417111, -6.526472994295373198 ) ) ;
#2733=CARTESIAN_POINT ( 'NONE',  ( -5.577813053751546416E-15, -25.45076803941176991, -5.092196395636519490 ) ) ;
#2734=CARTESIAN_POINT ( 'NONE',  ( -4.000000000000003553, 6.938893903907228378E-15, 0.000000000000000000 ) ) ;
#2735=CARTESIAN_POINT ( 'NONE',  ( -4.243569643750005227, -25.36948240980282421, -7.678405556576772817 ) ) ;
#2736=DIRECTION ( 'NONE',  ( -0.000000000000000000, -0.5735764363510414965, -0.8191520442889950182 ) ) ;
#2739=CARTESIAN_POINT ( 'NONE',  ( -8.500000000000005329, 0.000000000000000000, -20.49999999999999645 ) ) ;
#2740=CARTESIAN_POINT ( 'NONE',  ( 4.730628863548789710E-15, -18.11187661241681823, -10.12794063824400581 ) ) ;
#2741=DIRECTION ( 'NONE',  ( -0.000000000000000000, -0.5735764363510414965, -0.8191520442889950182 ) ) ;
#2744=CARTESIAN_POINT ( 'NONE',  ( 1.071796769724495224, -17.16683995969741616, -7.209095385566181236 ) ) ;
#2746=CARTESIAN_POINT ( 'NONE',  ( 1.999999999999994449, -28.60380821456909572, -10.52951475883191357 ) ) ;
#2748=CARTESIAN_POINT ( 'NONE',  ( -8.999999999999996447, -10.00000000000000000, -3.713574246709372417 ) ) ;
#2750=ORIENTED_EDGE ( 'NONE', *, *, #1841, .F. ) ;
#2752=CARTESIAN_POINT ( 'NONE',  ( -4.243569643749998122, -19.59184713035399383, -7.970067471831701056 ) ) ;
#2759=CARTESIAN_POINT ( 'NONE',  ( 1.071796769724485232, -29.31088228406247609, -10.60501085993131909 ) ) ;
#2760=CARTESIAN_POINT ( 'NONE',  ( -2.121784821875005722, -29.41649430960788081, -11.32239247872435506 ) ) ;
#2761=ORIENTED_EDGE ( 'NONE', *, *, #5135, .T. ) ;
#2762=CARTESIAN_POINT ( 'NONE',  ( 4.299564228933482956E-15, -17.73605940148895854, -8.022024996759636650 ) ) ;
#2764=CARTESIAN_POINT ( 'NONE',  ( 3.999999999999996447, -23.24856405356549871, -4.894592438216464281 ) ) ;
#2767=ORIENTED_EDGE ( 'NONE', *, *, #14672, .F. ) ;
#2768=CARTESIAN_POINT ( 'NONE',  ( -1.071796769724496334, -25.46229474013060567, -5.108658230292436819 ) ) ;
#2769=EDGE_CURVE ( 'NONE', #2986, #5758, #16423, .T. ) ;
#2776=CARTESIAN_POINT ( 'NONE',  ( -5.330712181944246111E-15, -28.88206442405900987, -8.423402447113589986 ) ) ;
#2784=CARTESIAN_POINT ( 'NONE',  ( -4.243569643749997233, -20.10806592306992613, -8.707304311691796528 ) ) ;
#2785=ORIENTED_EDGE ( 'NONE', *, *, #342, .T. ) ;
#2788=CARTESIAN_POINT ( 'NONE',  ( -4.000000000000000888, -24.30356238220903364, -10.42760410546358152 ) ) ;
#2793=CARTESIAN_POINT ( 'NONE',  ( -4.000000000000000888, -26.62654694943075029, -13.74516988483401114 ) ) ;
#2796=CARTESIAN_POINT ( 'NONE',  ( -5.279047395330986450E-15, -27.69989951318700250, -7.225440395136942584 ) ) ;
#2797=ORIENTED_EDGE ( 'NONE', *, *, #16786, .F. ) ;
#2799=CARTESIAN_POINT ( 'NONE',  ( 1.999999999999994449, -23.69972968376769273, -3.525764780161007472 ) ) ;
#2802=CARTESIAN_POINT ( 'NONE',  ( -2.121784821875005722, -26.06107215695429247, -6.530353019633736267 ) ) ;
#2804=CYLINDRICAL_SURFACE ( 'NONE', #6304, 4.000000000000000000 ) ;
#2813=ORIENTED_EDGE ( 'NONE', *, *, #16182, .T. ) ;
#2815=CARTESIAN_POINT ( 'NONE',  ( -5.330712181944245322E-15, -27.30114437136644767, -6.165614625042047159 ) ) ;
#2817=EDGE_CURVE ( 'NONE', #2141, #14057, #5137, .T. ) ;
#2821=CARTESIAN_POINT ( 'NONE',  ( 4.243569643750000786, -24.54553994094216307, -10.77318387364461572 ) ) ;
#2822=( BOUNDED_CURVE ( )  B_SPLINE_CURVE ( 2, ( #18126, #7986, #1139, #1049, #12434, #5302, #6602, #12339, #10953 ),
 .UNSPECIFIED., .F., .F. ) 
 B_SPLINE_CURVE_WITH_KNOTS ( ( 3, 2, 2, 2, 3 ),
 ( 0.7500000000000000000, 0.7528735632183908288, 0.7586206896551723755, 0.7643678160919540332, 0.7672413793103448620 ),
 .UNSPECIFIED. ) 
 CURVE ( )  GEOMETRIC_REPRESENTATION_ITEM ( )  RATIONAL_B_SPLINE_CURVE ( ( 0.9330127018922194093, 0.9330127018922194093, 1.000000000000000000, 0.8660254037844387076, 1.000000000000000000, 0.8660254037844387076, 1.000000000000000000, 0.9330127018922180770, 0.9330127018922194093 ) ) 
 REPRESENTATION_ITEM ( '' )  );
#2823=CARTESIAN_POINT ( 'NONE',  ( -14.99999999999999645, -4.000000000000000000, 30.00000000000000000 ) ) ;
#2824=CARTESIAN_POINT ( 'NONE',  ( 4.299564228933482956E-15, -22.38202853593239183, -14.65715655550049590 ) ) ;
#2826=CARTESIAN_POINT ( 'NONE',  ( -2.121784821875005722, -22.96375940065866672, -2.106931980473163879 ) ) ;
#2827=CARTESIAN_POINT ( 'NONE',  ( 4.000000000000003553, -22.77746674727289289, -12.27443157341021163 ) ) ;
#2830=CARTESIAN_POINT ( 'NONE',  ( 4.243569643750000786, -26.32004204090319632, -13.30743551066369257 ) ) ;
#2831=LINE ( 'NONE', #4482, #15473 ) ;
#2833=CARTESIAN_POINT ( 'NONE',  ( -9.178305741915819382, -9.999999999999996447, -2.937604372561400279 ) ) ;
#2835=VERTEX_POINT ( 'NONE', #4360 ) ;
#2836=CARTESIAN_POINT ( 'NONE',  ( -4.243569643750000786, -19.77051610831973605, -3.953743104938735708 ) ) ;
#2839=CARTESIAN_POINT ( 'NONE',  ( -2.121784821875005722, -28.64216612053397526, -10.21653721893421363 ) ) ;
#2840=LINE ( 'NONE', #13873, #2285 ) ;
#2841=DIRECTION ( 'NONE',  ( -0.000000000000000000, 1.000000000000000000, -0.000000000000000000 ) ) ;
#2843=CARTESIAN_POINT ( 'NONE',  ( 4.243569643750003451, -22.22671388484159039, -11.73304717528426977 ) ) ;
#2846=CARTESIAN_POINT ( 'NONE',  ( 4.000000000000003553, -17.87338821647148990, -5.270681594739305531 ) ) ;
#2848=ORIENTED_EDGE ( 'NONE', *, *, #9219, .T. ) ;
#2850=CARTESIAN_POINT ( 'NONE',  ( 3.579096709490575479E-14, -26.67678767140717966, -6.843133889297480899 ) ) ;
#2853=CARTESIAN_POINT ( 'NONE',  ( -4.243569643749998122, -22.17294109393367663, -11.65625167113217664 ) ) ;
#2856=ORIENTED_EDGE ( 'NONE', *, *, #3659, .T. ) ;
#2858=EDGE_CURVE ( 'NONE', #4607, #5051, #12979, .T. ) ;
#2859=CARTESIAN_POINT ( 'NONE',  ( -3.291771655530798757, -28.93493258167780269, -13.02337503524261386 ) ) ;
#2862=CARTESIAN_POINT ( 'NONE',  ( 4.243569643749996345, -24.50911775527627157, -6.449677490143276515 ) ) ;
#2863=ORIENTED_EDGE ( 'NONE', *, *, #1700, .T. ) ;
#2866=DIRECTION ( 'NONE',  ( -0.000000000000000000, -0.5735764363510414965, -0.8191520442889950182 ) ) ;
#2869=CARTESIAN_POINT ( 'NONE',  ( -4.000000000000000888, -24.04545298585106394, -10.05898568553353378 ) ) ;
#2876=CARTESIAN_POINT ( 'NONE',  ( 3.999999999999996447, -27.89453318800893555, -11.52972399695732264 ) ) ;
#2879=CARTESIAN_POINT ( 'NONE',  ( 2.000000000000004441, -20.97122678548641872, -11.70801252582615604 ) ) ;
#2881=ADVANCED_FACE ( 'NONE', ( #14485 ), #5631, .F. ) ;
#2882=DIRECTION ( 'NONE',  ( -0.000000000000000000, -0.5735764363510414965, -0.8191520442889950182 ) ) ;
#2883=VECTOR ( 'NONE', #8870, 1000.000000000000000 ) ;
#2885=CARTESIAN_POINT ( 'NONE',  ( -7.467367394352450560, -10.10642962993511951, 13.07819922209348107 ) ) ;
#2886=CARTESIAN_POINT ( 'NONE',  ( -2.121784821875005722, -26.57729094967022831, -7.267589859493831739 ) ) ;
#2888=CYLINDRICAL_SURFACE ( 'NONE', #15699, 2.000000000000001776 ) ;
#2893=CYLINDRICAL_SURFACE ( 'NONE', #12525, 4.000000000000000000 ) ;
#2894=CARTESIAN_POINT ( 'NONE',  ( -2.000000000000005773, -27.29175211571113735, -8.655704456514076384 ) ) ;
#2895=CARTESIAN_POINT ( 'NONE',  ( -1.071796769724488341, -23.66104881700340457, -16.48378682049481725 ) ) ;
#2897=AXIS2_PLACEMENT_3D ( 'NONE', #7667, #6806, #18151 ) ;
#2900=CARTESIAN_POINT ( 'NONE',  ( 4.730628863548789710E-15, -18.88620480149072378, -11.23379589803414902 ) ) ;
#2904=DIRECTION ( 'NONE',  ( -0.000000000000000000, -0.5735764363510414965, -0.8191520442889950182 ) ) ;
#2905=CARTESIAN_POINT ( 'NONE',  ( -5.330712181944245322E-15, -26.04286106412135027, -4.368599827883064890 ) ) ;
#2911=CARTESIAN_POINT ( 'NONE',  ( -3.999999999999997335, -19.07789873280866999, -6.990900887746200887 ) ) ;
#2912=CARTESIAN_POINT ( 'NONE',  ( 4.243569643750000786, -21.15785411374382363, -5.935067112062737849 ) ) ;
#2915=VERTEX_POINT ( 'NONE', #2157 ) ;
#2917=CARTESIAN_POINT ( 'NONE',  ( -5.330712181944245322E-15, -30.65656652402004312, -10.95765408413266861 ) ) ;
#2919=CARTESIAN_POINT ( 'NONE',  ( -9.609630862508756977, -9.971178627260298910, 12.03209595322010905 ) ) ;
#2921=DIRECTION ( 'NONE',  ( -0.000000000000000000, -0.5735764363510414965, -0.8191520442889950182 ) ) ;
#2925=( BOUNDED_CURVE ( )  B_SPLINE_CURVE ( 2, ( #11167, #6991, #6729, #14050, #12654, #1185, #12385, #18073, #16674 ),
 .UNSPECIFIED., .F., .F. ) 
 B_SPLINE_CURVE_WITH_KNOTS ( ( 3, 2, 2, 2, 3 ),
 ( 0.09482758620689656082, 0.09770114942528736190, 0.1034482758620689641, 0.1091954022988505801, 0.1120689655172413812 ),
 .UNSPECIFIED. ) 
 CURVE ( )  GEOMETRIC_REPRESENTATION_ITEM ( )  RATIONAL_B_SPLINE_CURVE ( ( 0.9330127018922194093, 0.9330127018922195203, 1.000000000000000000, 0.8660254037844387076, 1.000000000000000000, 0.8660254037844387076, 1.000000000000000000, 0.9330127018922194093, 0.9330127018922194093 ) ) 
 REPRESENTATION_ITEM ( '' )  );
#2927=CARTESIAN_POINT ( 'NONE',  ( 4.243569643750003451, -23.25915147027346563, -13.20752085500445894 ) ) ;
#2931=EDGE_CURVE ( 'NONE', #159, #6301, #8225, .T. ) ;
#2932=DIRECTION ( 'NONE',  ( 0.000000000000000000, 0.000000000000000000, 1.000000000000000000 ) ) ;
#2933=CARTESIAN_POINT ( 'NONE',  ( -2.121784821874996396, -21.15871460133474713, -12.34353118316265707 ) ) ;
#2935=CARTESIAN_POINT ( 'NONE',  ( 4.000000000000003553, -18.90582580190336515, -6.745155274459496475 ) ) ;
#2940=AXIS2_PLACEMENT_3D ( 'NONE', #13871, #6818, #12919 ) ;
#2942=CARTESIAN_POINT ( 'NONE',  ( -1.071796769724486786, -19.78940787163386972, -10.95451052154410299 ) ) ;
#2945=CARTESIAN_POINT ( 'NONE',  ( -2.121784821875005722, -27.12577341693091171, -8.050904001845182734 ) ) ;
#2951=CARTESIAN_POINT ( 'NONE',  ( -1.071796769724486786, -19.27318907891793032, -10.21727368168400751 ) ) ;
#2952=CARTESIAN_POINT ( 'NONE',  ( 4.000000000000003553, -19.35751724482486225, -7.390237508330316452 ) ) ;
#2953=DIRECTION ( 'NONE',  ( -1.000000000000000000, -0.000000000000000000, -0.000000000000000000 ) ) ;
#2955=CARTESIAN_POINT ( 'NONE',  ( 4.730628863548789710E-15, -16.85359330517172083, -8.330925841085024430 ) ) ;
#2965=EDGE_CURVE ( 'NONE', #6584, #9470, #7628, .T. ) ;
#2969=CARTESIAN_POINT ( 'NONE',  ( 4.000000000000003553, -22.19672060476252540, -11.44504012756084066 ) ) ;
#2970=VERTEX_POINT ( 'NONE', #9452 ) ;
#2972=DIRECTION ( 'NONE',  ( -0.000000000000000000, 1.000000000000000000, -0.000000000000000000 ) ) ;
#2976=CARTESIAN_POINT ( 'NONE',  ( -2.121784821875005722, -25.54485336423835307, -5.793116179773641683 ) ) ;
#2978=CARTESIAN_POINT ( 'NONE',  ( 1.999999999999994449, -22.86087414489934488, -2.327754914381585660 ) ) ;
#2982=CARTESIAN_POINT ( 'NONE',  ( -8.535862155143941976, -10.00000000000000178, 16.49127580077173150 ) ) ;
#2984=DIRECTION ( 'NONE',  ( 0.000000000000000000, 0.000000000000000000, 1.000000000000000000 ) ) ;
#2986=VERTEX_POINT ( 'NONE', #17918 ) ;
#2989=CARTESIAN_POINT ( 'NONE',  ( -5.330712181944245322E-15, -27.04303497500847797, -5.796996205112000311 ) ) ;
#2995=CARTESIAN_POINT ( 'NONE',  ( -1.661723472263481630E-14, -21.60770034685848984, -13.55130129571035447 ) ) ;
#2996=CARTESIAN_POINT ( 'NONE',  ( -2.121784821875005722, -26.09333583149904001, -6.576430322124992678 ) ) ;
#2997=AXIS2_PLACEMENT_3D ( 'NONE', #3088, #1797, #13190 ) ;
#3001=CARTESIAN_POINT ( 'NONE',  ( -4.243569643750000786, -20.25447122649092790, -4.644902642307576102 ) ) ;
#3002=LINE ( 'NONE', #7159, #17485 ) ;
#3006=CARTESIAN_POINT ( 'NONE',  ( -2.121784821874996396, -23.99791796127240318, -16.39833380239318217 ) ) ;
#3009=PRODUCT_DEFINITION ( 'UNKNOWN', '', #13086, #5188 ) ;
#3011=FACE_OUTER_BOUND ( 'NONE', #7766, .T. ) ;
#3014=CARTESIAN_POINT ( 'NONE',  ( 4.243569643750003451, -17.87111782130087434, -5.512611338964712893 ) ) ;
#3016=CARTESIAN_POINT ( 'NONE',  ( 2.121784821875004390, -24.07319986854348670, -16.50584750820610580 ) ) ;
#3017=AXIS2_PLACEMENT_3D ( 'NONE', #11025, #2607, #10937 ) ;
#3019=CARTESIAN_POINT ( 'NONE',  ( -4.243569643750000786, -26.19098734272420614, -13.12312630069867225 ) ) ;
#3023=CARTESIAN_POINT ( 'NONE',  ( -2.121784821874996396, -21.93304279040865623, -13.44938644295279850 ) ) ;
#3025=CARTESIAN_POINT ( 'NONE',  ( 1.999999999999994449, -22.92540149469378363, -2.419909520370864264 ) ) ;
#3027=VERTEX_POINT ( 'NONE', #8057 ) ;
#3029=CARTESIAN_POINT ( 'NONE',  ( -3.999999999999997335, -21.91710209274632604, -11.04570350697672509 ) ) ;
#3031=EDGE_CURVE ( 'NONE', #8354, #6383, #8246, .T. ) ;
#3036=( BOUNDED_CURVE ( )  B_SPLINE_CURVE ( 3, ( #18271, #18365, #161, #12767 ),
 .UNSPECIFIED., .F., .F. ) 
 B_SPLINE_CURVE_WITH_KNOTS ( ( 4, 4 ),
 ( 8.673617379884033500E-16, 1.570796326794896558 ),
 .UNSPECIFIED. ) 
 CURVE ( )  GEOMETRIC_REPRESENTATION_ITEM ( )  RATIONAL_B_SPLINE_CURVE ( ( 1.000000000000000000, 0.8047378541243652705, 0.8047378541243652705, 1.000000000000000000 ) ) 
 REPRESENTATION_ITEM ( '' )  );
#3039=CARTESIAN_POINT ( 'NONE',  ( 4.243569643749997233, -26.31588352978205592, -9.030006429653608890 ) ) ;
#3043=ADVANCED_FACE ( 'NONE', ( #5281 ), #5464, .F. ) ;
#3047=CARTESIAN_POINT ( 'NONE',  ( 6.428571428571431490, -11.73421655796352425, 14.25837509840157935 ) ) ;
#3049=CARTESIAN_POINT ( 'NONE',  ( 4.243569643750000786, -20.93200839193060148, -5.612525994623947412 ) ) ;
#3052=ORIENTED_EDGE ( 'NONE', *, *, #3999, .F. ) ;
#3053=VERTEX_POINT ( 'NONE', #15125 ) ;
#3061=EDGE_CURVE ( 'NONE', #2915, #17169, #5038, .T. ) ;
#3062=CARTESIAN_POINT ( 'NONE',  ( -4.000000000000004441, -25.59305773644543081, -8.242876418240973280 ) ) ;
#3066=CARTESIAN_POINT ( 'NONE',  ( -7.425558702535789202, -12.48286535448649914, 8.644520698117755586 ) ) ;
#3067=CARTESIAN_POINT ( 'NONE',  ( -5.330712181944246111E-15, -25.49437859686066687, -3.585285685531713451 ) ) ;
#3070=ORIENTED_EDGE ( 'NONE', *, *, #10734, .F. ) ;
#3074=CARTESIAN_POINT ( 'NONE',  ( -5.577813053751546416E-15, -26.41867827504920996, -6.474515469367432274 ) ) ;
#3076=CYLINDRICAL_SURFACE ( 'NONE', #63, 4.000000000000000000 ) ;
#3077=CARTESIAN_POINT ( 'NONE',  ( 1.071796769724485454, -21.55469969778287975, -13.47560852437699452 ) ) ;
#3080=CARTESIAN_POINT ( 'NONE',  ( 4.299564228933482956E-15, -22.38202853593239183, -14.65715655550049590 ) ) ;
#3081=CARTESIAN_POINT ( 'NONE',  ( 4.243569643750003451, -20.16183871397784344, -8.784099815843886105 ) ) ;
#3085=CARTESIAN_POINT ( 'NONE',  ( 4.713407268011036227E-15, -23.35926451522188430, -17.13164280311214327 ) ) ;
#3086=CARTESIAN_POINT ( 'NONE',  ( -2.121784821875005722, -25.31900764242513091, -5.470575062334849470 ) ) ;
#3088=CARTESIAN_POINT ( 'NONE',  ( 8.500000000000019540, 10.00000000000000000, 20.49999999999998934 ) ) ;
#3089=CARTESIAN_POINT ( 'NONE',  ( -8.767957691171661239, -10.00000000000000178, -4.386791830708038908 ) ) ;
#3093=CARTESIAN_POINT ( 'NONE',  ( -1.661723472263481630E-14, -21.54317299706404754, -13.45914668972107897 ) ) ;
#3094=CARTESIAN_POINT ( 'NONE',  ( -4.243569643750005227, -22.75612477167838676, -3.946144054785039490 ) ) ;
#3095=LINE ( 'NONE', #15704, #7079 ) ;
#3096=DIRECTION ( 'NONE',  ( 0.000000000000000000, 0.000000000000000000, 1.000000000000000000 ) ) ;
#3100=CARTESIAN_POINT ( 'NONE',  ( -4.243569643750000786, -26.96531553179811169, -14.22898156048881724 ) ) ;
#3101=CARTESIAN_POINT ( 'NONE',  ( -8.500000000000005329, 0.000000000000000000, -22.50000000000000000 ) ) ;
#3104=ADVANCED_FACE ( 'NONE', ( #16890 ), #13624, .F. ) ;
#3106=CARTESIAN_POINT ( 'NONE',  ( 9.000000000000007105, -10.00000000000000178, -3.713574246709336002 ) ) ;
#3108=CARTESIAN_POINT ( 'NONE',  ( 4.243569643749997233, -22.70235198077049432, -3.869348550632942363 ) ) ;
#3110=CARTESIAN_POINT ( 'NONE',  ( -4.243569643750000786, -26.99757920634285924, -14.27505886298007276 ) ) ;
#3112=CARTESIAN_POINT ( 'NONE',  ( -4.000000000000004441, -26.10927652916136310, -8.980113258101068752 ) ) ;
#3113=CARTESIAN_POINT ( 'NONE',  ( -2.121784821875005722, -28.12594732781803941, -9.479300379074118155 ) ) ;
#3116=CARTESIAN_POINT ( 'NONE',  ( 1.999999999999994449, -28.86191761092706187, -10.89813317876196308 ) ) ;
#3117=CARTESIAN_POINT ( 'NONE',  ( 2.121784821874994176, -27.30860090601781209, -8.312008715962296179 ) ) ;
#3119=CARTESIAN_POINT ( 'NONE',  ( -4.000000000000000888, -20.43192143683950590, -4.898327806512866367 ) ) ;
#3125=CARTESIAN_POINT ( 'NONE',  ( -5.577813053751546416E-15, -26.22509622848567545, -6.198051655426662698 ) ) ;
#3128=CARTESIAN_POINT ( 'NONE',  ( -4.243569643750000786, -24.41648524276317289, -10.58887466367959540 ) ) ;
#3131=CARTESIAN_POINT ( 'NONE',  ( 4.730628863548789710E-15, -21.75767183597312737, -15.33467581975593141 ) ) ;
#3132=CARTESIAN_POINT ( 'NONE',  ( 1.071796769724495224, -18.71549633784523081, -9.420805905146465875 ) ) ;
#3133=CARTESIAN_POINT ( 'NONE',  ( 2.694913683823408235, -10.54254386713301805, 22.30101802474215233 ) ) ;
#3135=CARTESIAN_POINT ( 'NONE',  ( 2.121784821875004390, -18.65290254502614431, -8.764860689675106897 ) ) ;
#3137=CARTESIAN_POINT ( 'NONE',  ( 4.000000000000003553, -20.38995483025674105, -8.864711188050506507 ) ) ;
#3141=( BOUNDED_CURVE ( )  B_SPLINE_CURVE ( 2, ( #7426, #3456, #400, #7609, #7330, #9097, #6325, #5946, #6038 ),
 .UNSPECIFIED., .F., .T. ) 
 B_SPLINE_CURVE_WITH_KNOTS ( ( 3, 2, 2, 2, 3 ),
 ( 0.9568965517241379004, 0.9597701149425287293, 0.9655172413793103869, 0.9712643678160919336, 0.9741379310344827624 ),
 .UNSPECIFIED. ) 
 CURVE ( )  GEOMETRIC_REPRESENTATION_ITEM ( )  RATIONAL_B_SPLINE_CURVE ( ( 0.9330127018922194093, 0.9330127018922194093, 1.000000000000000000, 0.8660254037844387076, 1.000000000000000000, 0.8660254037844387076, 1.000000000000000000, 0.9330127018922194093, 0.9330127018922194093 ) ) 
 REPRESENTATION_ITEM ( '' )  );
#3142=AXIS2_PLACEMENT_3D ( 'NONE', #1145, #9835, #5590 ) ;
#3143=CARTESIAN_POINT ( 'NONE',  ( -4.000000000000000888, -20.43192143683950590, -4.898327806512866367 ) ) ;
#3145=DIRECTION ( 'NONE',  ( -0.000000000000000000, -1.000000000000000000, -0.000000000000000000 ) ) ;
#3148=B_SPLINE_CURVE_WITH_KNOTS ( 'NONE', 3,
 ( #10112, #7335, #11880, #3370, #15983, #15883, #9103, #3279, #6233, #5858, #8914, #13274, #17578, #9014 ),
 .UNSPECIFIED., .F., .F.,
 ( 4, 2, 2, 2, 2, 2, 4 ),
 ( 0.000000000000000000, 0.004344441487376424042, 0.008688882974752848085, 0.01086110371844106227, 0.01303332446212927473, 0.01520554520581748718, 0.01737776594950569964 ),
 .UNSPECIFIED. ) ;
#3154=CARTESIAN_POINT ( 'NONE',  ( -5.279047395330986450E-15, -26.66746192775513080, -5.750966715416751640 ) ) ;
#3156=CARTESIAN_POINT ( 'NONE',  ( 4.898587196589413815E-16, 2.700915433685006750, 35.11257424290206330 ) ) ;
#3158=CARTESIAN_POINT ( 'NONE',  ( -7.666554591372073624, -10.31261801969990444, 7.182588619990075252 ) ) ;
#3159=CARTESIAN_POINT ( 'NONE',  ( -2.121784821874996396, -19.09383943047100018, -9.394583823722271632 ) ) ;
#3165=EDGE_LOOP ( 'NONE', ( #15403, #364, #9885, #13609, #4187 ) ) ;
#3168=CARTESIAN_POINT ( 'NONE',  ( 4.299564228933482956E-15, -22.89824732864832768, -15.39439339536058959 ) ) ;
#3173=CARTESIAN_POINT ( 'NONE',  ( -4.243569643749997233, -19.30147405945127304, -7.555371749410396021 ) ) ;
#3176=CARTESIAN_POINT ( 'NONE',  ( 2.121784821874994176, -29.92195854414224598, -12.04427021775403084 ) ) ;
#3178=CARTESIAN_POINT ( 'NONE',  ( 3.999999999999996447, -28.86244342364637205, -12.91204307068823987 ) ) ;
#3179=CARTESIAN_POINT ( 'NONE',  ( -4.243569643749997233, -20.36617531942789228, -9.075922731621842487 ) ) ;
#3180=CARTESIAN_POINT ( 'NONE',  ( 3.579096709490575479E-14, -25.12813129325936501, -4.631423369717193594 ) ) ;
#3181=CARTESIAN_POINT ( 'NONE',  ( -3.820650143297558365, -10.00000000000057199, -3.109998371641696124 ) ) ;
#3182=CARTESIAN_POINT ( 'NONE',  ( 0.000000000000000000, 9.254131787996968228, 30.52396275209373044 ) ) ;
#3186=AXIS2_PLACEMENT_3D ( 'NONE', #4405, #2841, #1543 ) ;
#3188=CARTESIAN_POINT ( 'NONE',  ( 2.121784821874994176, -23.69506935700625050, -3.151350836941627875 ) ) ;
#3196=CYLINDRICAL_SURFACE ( 'NONE', #12014, 4.000000000000000000 ) ;
#3197=EDGE_CURVE ( 'NONE', #269, #11442, #11301, .T. ) ;
#3200=CARTESIAN_POINT ( 'NONE',  ( 4.243569643750000786, -27.12663390452184942, -14.45936807294509308 ) ) ;
#3201=EDGE_CURVE ( 'NONE', #6301, #8381, #15753, .T. ) ;
#3204=CYLINDRICAL_SURFACE ( 'NONE', #3981, 4.000000000000000000 ) ;
#3205=CARTESIAN_POINT ( 'NONE',  ( 4.243569643749997233, -28.09038562974308562, -11.56425806667268752 ) ) ;
#3208=CARTESIAN_POINT ( 'NONE',  ( -4.000000000000000888, -24.56167177856700334, -10.79622252539362925 ) ) ;
#3210=CARTESIAN_POINT ( 'NONE',  ( 4.243569643749996345, -26.28361985523730837, -8.983929127162353367 ) ) ;
#3212=CARTESIAN_POINT ( 'NONE',  ( -4.000000000000000888, -19.91570264412356650, -4.161090966652770895 ) ) ;
#3219=CARTESIAN_POINT ( 'NONE',  ( 2.000000000000004441, -21.03575413528086102, -11.80016713181543331 ) ) ;
#3220=CARTESIAN_POINT ( 'NONE',  ( 4.000000000000003553, -24.84234191813664339, -15.22337893285059529 ) ) ;
#3224=CARTESIAN_POINT ( 'NONE',  ( 2.121784821875004390, -20.45966831953192511, -11.34518962918543927 ) ) ;
#3229=CARTESIAN_POINT ( 'NONE',  ( -5.577813053751546416E-15, -23.38589286854802296, -2.143249036196138047 ) ) ;
#3230=CARTESIAN_POINT ( 'NONE',  ( 4.730628863548789710E-15, -22.01578123233109707, -15.70329423968597915 ) ) ;
#3232=CARTESIAN_POINT ( 'NONE',  ( 0.000000000000000000, 9.254131787996968228, 30.52396275209373044 ) ) ;
#3234=CARTESIAN_POINT ( 'NONE',  ( -4.243569643750000786, -21.31917248646755070, -6.165453624519022569 ) ) ;
#3236=CARTESIAN_POINT ( 'NONE',  ( -1.999999999999996225, -20.73462650619655534, -11.37011230856371036 ) ) ;
#3237=CARTESIAN_POINT ( 'NONE',  ( -5.577813053751546416E-15, -25.64435008597530796, -5.368660209577289955 ) ) ;
#3240=ORIENTED_EDGE ( 'NONE', *, *, #9829, .T. ) ;
#3247=ORIENTED_EDGE ( 'NONE', *, *, #10691, .F. ) ;
#3249=CARTESIAN_POINT ( 'NONE',  ( -1.999999999999996225, -18.60522398553836965, -8.329010343134054750 ) ) ;
#3253=CARTESIAN_POINT ( 'NONE',  ( -9.320967924960621431, -9.992678415326631480, -2.177024574453123140 ) ) ;
#3255=CARTESIAN_POINT ( 'NONE',  ( -4.243569643749998122, -19.30147405945127304, -7.555371749410397797 ) ) ;
#3256=( BOUNDED_CURVE ( )  B_SPLINE_CURVE ( 2, ( #3168, #4190, #11398, #12619, #5843, #18307, #1685, #11585, #16913 ),
 .UNSPECIFIED., .F., .F. ) 
 B_SPLINE_CURVE_WITH_KNOTS ( ( 3, 2, 2, 2, 3 ),
 ( 0.1120689655172413812, 0.1149425287356321823, 0.1206896551724137984, 0.1264367816091954144, 0.1293103448275862155 ),
 .UNSPECIFIED. ) 
 CURVE ( )  GEOMETRIC_REPRESENTATION_ITEM ( )  RATIONAL_B_SPLINE_CURVE ( ( 0.9330127018922194093, 0.9330127018922194093, 1.000000000000000000, 0.8660254037844387076, 1.000000000000000000, 0.8660254037844387076, 1.000000000000000000, 0.9330127018922194093, 0.9330127018922194093 ) ) 
 REPRESENTATION_ITEM ( '' )  );
#3259=ORIENTED_EDGE ( 'NONE', *, *, #9603, .T. ) ;
#3265=ORIENTED_EDGE ( 'NONE', *, *, #11841, .F. ) ;
#3268=CARTESIAN_POINT ( 'NONE',  ( 2.000000000000004441, -22.84251990978664182, -14.38049607132576746 ) ) ;
#3269=CARTESIAN_POINT ( 'NONE',  ( -4.243569643749997233, -20.07580224852517858, -8.661227009200541005 ) ) ;
#3274=CARTESIAN_POINT ( 'NONE',  ( 4.243569643749997233, -28.63886809700377611, -12.34757220902403851 ) ) ;
#3275=CARTESIAN_POINT ( 'NONE',  ( -4.000000000000000888, -26.82012899599428124, -14.02163369877478161 ) ) ;
#3277=CARTESIAN_POINT ( 'NONE',  ( -5.330712181944245322E-15, -27.07529864955322552, -5.843073507603255834 ) ) ;
#3278=ADVANCED_FACE ( 'NONE', ( #7117 ), #7208, .F. ) ;
#3279=CARTESIAN_POINT ( 'NONE',  ( -7.381432656702920703, -13.34861180364788247, 2.835002125509740623 ) ) ;
#3280=CARTESIAN_POINT ( 'NONE',  ( -7.649231854195242875, -10.00000000000000178, -6.849627928939406196 ) ) ;
#3281=CARTESIAN_POINT ( 'NONE',  ( 1.071796769724485232, -23.56794821439272880, -2.403251015480991626 ) ) ;
#3282=CARTESIAN_POINT ( 'NONE',  ( 0.000000000000000000, 5.977523610840987267, 32.81826849749789687 ) ) ;
#3283=ORIENTED_EDGE ( 'NONE', *, *, #11462, .T. ) ;
#3284=EDGE_LOOP ( 'NONE', ( #9897, #4410, #14663, #13878 ) ) ;
#3285=CARTESIAN_POINT ( 'NONE',  ( 4.898587196589413815E-16, 2.700915433685006750, 35.11257424290206330 ) ) ;
#3288=FILL_AREA_STYLE_COLOUR ( '', #4181 ) ;
#3289=CARTESIAN_POINT ( 'NONE',  ( 4.730628863548789710E-15, -21.20918936871244043, -14.55136167740457864 ) ) ;
#3292=CARTESIAN_POINT ( 'NONE',  ( 1.448116719718851364, -9.999999999999500844, -4.839896329769187489 ) ) ;
#3293=ORIENTED_EDGE ( 'NONE', *, *, #13111, .T. ) ;
#3295=CARTESIAN_POINT ( 'NONE',  ( 4.000000000000000888, -19.98022999250811793, -4.253245570628513939 ) ) ;
#3297=CARTESIAN_POINT ( 'NONE',  ( -4.243569643750004339, -25.59532813161605347, -8.000946674015564142 ) ) ;
#3298=CARTESIAN_POINT ( 'NONE',  ( 0.000000000000000000, -10.00099999999999767, 0.000000000000000000 ) ) ;
#3301=CARTESIAN_POINT ( 'NONE',  ( -4.243569643750005227, -24.82099994254214437, -6.895091414225420934 ) ) ;
#3305=LINE ( 'NONE', #1930, #8519 ) ;
#3307=ADVANCED_FACE ( 'NONE', ( #12777 ), #171, .F. ) ;
#3308=CARTESIAN_POINT ( 'NONE',  ( 1.999999999999994449, -27.31326123277925433, -8.686422659181676664 ) ) ;
#3310=CARTESIAN_POINT ( 'NONE',  ( -3.999999999999997335, -24.24008665996804268, -14.36326928634715472 ) ) ;
#3314=CARTESIAN_POINT ( 'NONE',  ( -2.121784821874996396, -20.41665008680558913, -11.28375322586376939 ) ) ;
#3316=AXIS2_PLACEMENT_3D ( 'NONE', #14974, #15248, #2270 ) ;
#3318=CARTESIAN_POINT ( 'NONE',  ( 1.999999999999994449, -24.40953052304715953, -4.539465433961872520 ) ) ;
#3320=CARTESIAN_POINT ( 'NONE',  ( -2.121784821874996396, -21.96530646495340378, -13.49546374544405403 ) ) ;
#3321=CARTESIAN_POINT ( 'NONE',  ( -5.577813053751546416E-15, -28.54808079570739920, -9.515617434797091434 ) ) ;
#3322=LINE ( 'NONE', #17435, #1778 ) ;
#3323=CARTESIAN_POINT ( 'NONE',  ( 3.579096709490575479E-14, -25.90245948233327056, -5.737278629507336802 ) ) ;
#3324=CARTESIAN_POINT ( 'NONE',  ( -4.243569643750000786, -21.06106309010958100, -5.796835204588974833 ) ) ;
#3326=ORIENTED_EDGE ( 'NONE', *, *, #14028, .T. ) ;
#3327=LINE ( 'NONE', #1949, #9788 ) ;
#3333=VERTEX_POINT ( 'NONE', #5915 ) ;
#3342=CARTESIAN_POINT ( 'NONE',  ( -3.999999999999997335, -19.78769957208813679, -8.004601541547065935 ) ) ;
#3344=AXIS2_PLACEMENT_3D ( 'NONE', #14936, #2228, #7855 ) ;
#3349=CARTESIAN_POINT ( 'NONE',  ( 4.730628863548789710E-15, -17.85376721605885209, -9.759322218313958075 ) ) ;
#3352=VERTEX_POINT ( 'NONE', #11561 ) ;
#3354=CARTESIAN_POINT ( 'NONE',  ( 3.579096709490575479E-14, -23.06325612239561451, -1.682476010276811040 ) ) ;
#3357=CARTESIAN_POINT ( 'NONE',  ( 3.999999999999996447, 6.938893903907228378E-15, 24.28148006742132026 ) ) ;
#3362=CARTESIAN_POINT ( 'NONE',  ( 4.898587196589413815E-16, 2.700915433685006750, 35.11257424290206330 ) ) ;
#3363=CARTESIAN_POINT ( 'NONE',  ( -5.330712181944245322E-15, -25.75248799321863657, -3.953904105461760743 ) ) ;
#3365=EDGE_CURVE ( 'NONE', #14905, #4281, #13321, .T. ) ;
#3367=CARTESIAN_POINT ( 'NONE',  ( -4.243569643749998122, -24.49592566115538972, -14.97381745050260804 ) ) ;
#3368=CARTESIAN_POINT ( 'NONE',  ( -1.999999999999996225, -22.99308372362383679, -14.59552348194486626 ) ) ;
#3369=CARTESIAN_POINT ( 'NONE',  ( -4.243569643749997233, -19.33373773399602058, -7.601449051901653320 ) ) ;
#3370=CARTESIAN_POINT ( 'NONE',  ( -7.429936681370006291, -12.48975054434458620, 8.592747494639136008 ) ) ;
#3375=ORIENTED_EDGE ( 'NONE', *, *, #17613, .T. ) ;
#3376=ORIENTED_EDGE ( 'NONE', *, *, #1981, .F. ) ;
#3379=CARTESIAN_POINT ( 'NONE',  ( 4.000000000000003553, -23.74537698291033294, -13.65675064714112708 ) ) ;
#3380=LINE ( 'NONE', #9021, #12370 ) ;
#3383=CARTESIAN_POINT ( 'NONE',  ( -4.648177544792955347E-16, -29.77410042770280185, -11.26655492845805107 ) ) ;
#3384=CARTESIAN_POINT ( 'NONE',  ( -5.330712181944245322E-15, -29.10791014587222847, -8.745943564552380423 ) ) ;
#3386=ADVANCED_FACE ( 'NONE', ( #17815 ), #14558, .F. ) ;
#3390=CARTESIAN_POINT ( 'NONE',  ( 4.730628863548789710E-15, -21.49956243961515767, -14.96605739982588368 ) ) ;
#3391=CARTESIAN_POINT ( 'NONE',  ( -1.999999999999996225, -21.44442734547602569, -12.38381296236458162 ) ) ;
#3392=CARTESIAN_POINT ( 'NONE',  ( -4.243569643749998122, -22.39878681574689878, -11.97879278857096885 ) ) ;
#3393=CARTESIAN_POINT ( 'NONE',  ( 3.579096709490575479E-14, -23.06325612239561451, -1.682476010276811040 ) ) ;
#3396=CARTESIAN_POINT ( 'NONE',  ( -4.243569643750000786, -23.09367458642858040, -8.699705261538101198 ) ) ;
#3398=CARTESIAN_POINT ( 'NONE',  ( 0.000000000000000000, 5.977523610840987267, 32.81826849749789687 ) ) ;
#3401=ORIENTED_EDGE ( 'NONE', *, *, #2931, .F. ) ;
#3405=CARTESIAN_POINT ( 'NONE',  ( 3.999999999999996447, -27.12020499893502645, -10.42386873716718121 ) ) ;
#3409=CARTESIAN_POINT ( 'NONE',  ( -4.243569643750000786, -23.38404765733129764, -9.114400983959404456 ) ) ;
#3411=ORIENTED_EDGE ( 'NONE', *, *, #12016, .T. ) ;
#3412=CYLINDRICAL_SURFACE ( 'NONE', #16128, 2.000000000000001776 ) ;
#3414=CARTESIAN_POINT ( 'NONE',  ( 4.243569643750003451, -23.29141514481821318, -13.25359815749571268 ) ) ;
#3415=DIRECTION ( 'NONE',  ( -1.000000000000000000, 0.000000000000000000, 0.000000000000000000 ) ) ;
#3416=CARTESIAN_POINT ( 'NONE',  ( 7.706178721746812954, -10.26817993880334257, 8.683600939131450147 ) ) ;
#3419=( BOUNDED_CURVE ( )  B_SPLINE_CURVE ( 2, ( #7711, #13640, #9104, #4846, #7614, #1990, #13462, #10860, #15050 ),
 .UNSPECIFIED., .F., .T. ) 
 B_SPLINE_CURVE_WITH_KNOTS ( ( 3, 2, 2, 2, 3 ),
 ( 0.2155172413793103592, 0.2183908045977011603, 0.2241379310344827624, 0.2298850574712643646, 0.2327586206896551657 ),
 .UNSPECIFIED. ) 
 CURVE ( )  GEOMETRIC_REPRESENTATION_ITEM ( )  RATIONAL_B_SPLINE_CURVE ( ( 0.9330127018922192983, 0.9330127018922196314, 1.000000000000000000, 0.8660254037844387076, 1.000000000000000000, 0.8660254037844387076, 1.000000000000000000, 0.9330127018922194093, 0.9330127018922194093 ) ) 
 REPRESENTATION_ITEM ( '' )  );
#3420=CARTESIAN_POINT ( 'NONE',  ( 4.243569643749996345, -28.86471381881699116, -12.67011332646282895 ) ) ;
#3423=CARTESIAN_POINT ( 'NONE',  ( 4.713407268011036227E-15, -19.03593212693084524, -10.95728427029060725 ) ) ;
#3428=PLANE ( 'NONE',  #14596 ) ;
#3434=CARTESIAN_POINT ( 'NONE',  ( 1.999999999999994449, -24.92574931576309538, -5.276702273821968880 ) ) ;
#3435=ORIENTED_EDGE ( 'NONE', *, *, #15188, .T. ) ;
#3436=ADVANCED_FACE ( 'NONE', ( #9068 ), #17445, .F. ) ;
#3437=DIRECTION ( 'NONE',  ( 0.000000000000000000, 0.8191520442889952403, -0.5735764363510413855 ) ) ;
#3439=CARTESIAN_POINT ( 'NONE',  ( 2.000000000000004441, -22.51988316363423337, -13.91972304540644245 ) ) ;
#3441=CARTESIAN_POINT ( 'NONE',  ( -2.121784821875005722, -24.25430638244851167, -3.950024080123402559 ) ) ;
#3442=CARTESIAN_POINT ( 'NONE',  ( -4.243569643750000786, -23.64215705368926379, -9.483019403889452192 ) ) ;
#3445=ORIENTED_EDGE ( 'NONE', *, *, #1176, .F. ) ;
#3446=CIRCLE ( 'NONE', #1379, 2.000000000000001776 ) ;
#3447=CARTESIAN_POINT ( 'NONE',  ( 4.772237607920560620, -11.09252097142802640, 18.58920227068357178 ) ) ;
#3452=CARTESIAN_POINT ( 'NONE',  ( -2.121784821874996396, -18.06140184503912494, -7.920110144002082464 ) ) ;
#3456=CARTESIAN_POINT ( 'NONE',  ( 1.071796769724485232, -23.11625677147122104, -1.758168781610173204 ) ) ;
#3457=CARTESIAN_POINT ( 'NONE',  ( 2.000000000000004441, -23.55232074906610507, -15.39419672512663340 ) ) ;
#3458=CARTESIAN_POINT ( 'NONE',  ( 4.243569643749996345, -23.21857077348643017, -4.606585390493037835 ) ) ;
#3459=VECTOR ( 'NONE', #8843, 1000.000000000000000 ) ;
#3461=CARTESIAN_POINT ( 'NONE',  ( -14.99999999999999645, 10.00000000000000000, 30.00000000000000000 ) ) ;
#3467=VECTOR ( 'NONE', #5457, 1000.000000000000000 ) ;
#3473=CARTESIAN_POINT ( 'NONE',  ( 4.243569643750000786, -25.28760445547132107, -11.83296183094350340 ) ) ;
#3476=CARTESIAN_POINT ( 'NONE',  ( 2.220605816132281252, -15.34963770581821763, -10.14223552587152888 ) ) ;
#3477=CARTESIAN_POINT ( 'NONE',  ( -5.330712181944245322E-15, -29.91450200949088156, -9.897876126833780930 ) ) ;
#3479=CARTESIAN_POINT ( 'NONE',  ( 2.121784821875004390, -21.45984223041904926, -12.77358600641437469 ) ) ;
#3480=CARTESIAN_POINT ( 'NONE',  ( 3.608366422512736094, -25.49736372916365212, -15.63892331459559593 ) ) ;
#3482=CARTESIAN_POINT ( 'NONE',  ( -2.121784821875005722, -26.57729094967022831, -7.267589859493831739 ) ) ;
#3483=ORIENTED_EDGE ( 'NONE', *, *, #3497, .T. ) ;
#3484=CARTESIAN_POINT ( 'NONE',  ( 1.533898589781675205E-14, -27.45111586048108521, -7.948989149087622330 ) ) ;
#3487=ORIENTED_EDGE ( 'NONE', *, *, #10565, .F. ) ;
#3489=CARTESIAN_POINT ( 'NONE',  ( -1.071796769724486564, -27.01095111827842388, -7.320368749872718794 ) ) ;
#3496=CARTESIAN_POINT ( 'NONE',  ( -2.121784821874996396, -19.90043129408965328, -10.54651638600367214 ) ) ;
#3497=EDGE_CURVE ( 'NONE', #5271, #11449, #9412, .T. ) ;
#3502=CARTESIAN_POINT ( 'NONE',  ( -5.330712181944245322E-15, -29.65639261313291541, -9.529257706903733194 ) ) ;
#3504=( GEOMETRIC_REPRESENTATION_CONTEXT ( 3 ) GLOBAL_UNCERTAINTY_ASSIGNED_CONTEXT ( ( #13791 ) ) GLOBAL_UNIT_ASSIGNED_CONTEXT ( ( #15992, #17206, #413 ) ) REPRESENTATION_CONTEXT ( 'NONE', 'WORKASPACE' ) );
#3509=CARTESIAN_POINT ( 'NONE',  ( 2.121784821875004390, -17.36235556323629936, -6.921768590024867329 ) ) ;
#3510=VERTEX_POINT ( 'NONE', #9252 ) ;
#3511=CARTESIAN_POINT ( 'NONE',  ( 4.000000000000000888, -23.14207009859818243, -8.768821215778363154 ) ) ;
#3512=CARTESIAN_POINT ( 'NONE',  ( 1.999999999999994449, -26.28082364734737908, -7.211948979461484832 ) ) ;
#3515=CARTESIAN_POINT ( 'NONE',  ( -1.999999999999996225, -18.60522398553836965, -8.329010343134054750 ) ) ;
#3521=VECTOR ( 'NONE', #12068, 1000.000000000000000 ) ;
#3524=CARTESIAN_POINT ( 'NONE',  ( -5.279047395330986450E-15, -26.15124313503919495, -5.013729875556656168 ) ) ;
#3525=ORIENTED_EDGE ( 'NONE', *, *, #14847, .T. ) ;
#3528=( BOUNDED_CURVE ( )  B_SPLINE_CURVE ( 2, ( #16539, #3815, #12772, #16726, #5301, #4001, #10952, #15140, #12951 ),
 .UNSPECIFIED., .F., .T. ) 
 B_SPLINE_CURVE_WITH_KNOTS ( ( 3, 2, 2, 2, 3 ),
 ( 0.1465517241379310498, 0.1494252873563218509, 0.1551724137931034531, 0.1609195402298850552, 0.1637931034482758563 ),
 .UNSPECIFIED. ) 
 CURVE ( )  GEOMETRIC_REPRESENTATION_ITEM ( )  RATIONAL_B_SPLINE_CURVE ( ( 0.9330127018922192983, 0.9330127018922196314, 1.000000000000000000, 0.8660254037844387076, 1.000000000000000000, 0.8660254037844387076, 1.000000000000000000, 0.9330127018922194093, 0.9330127018922194093 ) ) 
 REPRESENTATION_ITEM ( '' )  );
#3529=CARTESIAN_POINT ( 'NONE',  ( -5.577813053751546416E-15, -28.74166284227092305, -9.792081248737861898 ) ) ;
#3530=CARTESIAN_POINT ( 'NONE',  ( -5.330712181944246111E-15, -24.20383161507082193, -1.742193585881474771 ) ) ;
#3531=CARTESIAN_POINT ( 'NONE',  ( 2.121784821875004390, -20.97588711224786095, -12.08242646904553474 ) ) ;
#3536=ORIENTED_EDGE ( 'NONE', *, *, #1110, .T. ) ;
#3537=CARTESIAN_POINT ( 'NONE',  ( -0.6435604995507047121, -10.54254386713301628, 22.30101802474215233 ) ) ;
#3538=EDGE_CURVE ( 'NONE', #12774, #8670, #11313, .T. ) ;
#3540=CARTESIAN_POINT ( 'NONE',  ( -5.577813053751546416E-15, -25.96698683212770931, -5.829433235496615850 ) ) ;
#3541=ORIENTED_EDGE ( 'NONE', *, *, #6831, .T. ) ;
#3544=CARTESIAN_POINT ( 'NONE',  ( 4.243569643750000786, -21.93218230281772918, -7.040922371852881945 ) ) ;
#3547=CARTESIAN_POINT ( 'NONE',  ( -4.243569643749998122, -24.23781626479742712, -14.60519903057256208 ) ) ;
#3548=CARTESIAN_POINT ( 'NONE',  ( -2.000000000000005773, -28.84040849385894845, -10.86741497609436280 ) ) ;
#3550=CARTESIAN_POINT ( 'NONE',  ( -5.330712181944245322E-15, -25.26853287504744472, -3.262744568092923014 ) ) ;
#3556=VERTEX_POINT ( 'NONE', #13511 ) ;
#3559=EDGE_CURVE ( 'NONE', #16544, #5572, #10717, .T. ) ;
#3560=CARTESIAN_POINT ( 'NONE',  ( 3.999999999999996447, -22.66781791105512767, -4.065200992367092425 ) ) ;
#3561=CARTESIAN_POINT ( 'NONE',  ( 4.299564228933482956E-15, -22.57561058249592278, -14.93362036944126814 ) ) ;
#3565=EDGE_CURVE ( 'NONE', #10757, #18352, #7019, .T. ) ;
#3566=CARTESIAN_POINT ( 'NONE',  ( -4.243569643749997233, -24.20555259025267603, -14.55912172808130656 ) ) ;
#3569=CARTESIAN_POINT ( 'NONE',  ( 4.730628863548789710E-15, -22.01578123233109707, -15.70329423968597915 ) ) ;
#3571=AXIS2_PLACEMENT_3D ( 'NONE', #7197, #16302, #4600 ) ;
#3574=CARTESIAN_POINT ( 'NONE',  ( 4.243569643750003451, -20.93616690305174544, -9.889955075634029313 ) ) ;
#3575=CARTESIAN_POINT ( 'NONE',  ( 1.533898589781675205E-14, -27.19300646412311551, -7.580370729157575482 ) ) ;
#3576=CARTESIAN_POINT ( 'NONE',  ( -8.500000000000005329, 10.00000000000000000, 20.49999999999999645 ) ) ;
#3584=VERTEX_POINT ( 'NONE', #5443 ) ;
#3585=CARTESIAN_POINT ( 'NONE',  ( -2.121784821875005722, -25.57711703878310061, -5.839193482264897206 ) ) ;
#3590=CARTESIAN_POINT ( 'NONE',  ( -3.250871920745033616, -25.09854970161199716, -15.79815562995958977 ) ) ;
#3591=( GEOMETRIC_REPRESENTATION_CONTEXT ( 3 ) GLOBAL_UNCERTAINTY_ASSIGNED_CONTEXT ( ( #8257 ) ) GLOBAL_UNIT_ASSIGNED_CONTEXT ( ( #8924, #6342, #16364 ) ) REPRESENTATION_CONTEXT ( 'NONE', 'WORKASPACE' ) );
#3592=CARTESIAN_POINT ( 'NONE',  ( 9.000000000000005329, -10.00000000000000178, 15.14468620625654616 ) ) ;
#3593=CARTESIAN_POINT ( 'NONE',  ( 1.533898589781675205E-14, -27.96733465319702105, -8.686225988947720467 ) ) ;
#3594=CARTESIAN_POINT ( 'NONE',  ( 4.243569643750000786, -27.09437022997710187, -14.41329077045383578 ) ) ;
#3596=CARTESIAN_POINT ( 'NONE',  ( 4.000000000000003553, -21.22881036912508179, -10.06272105382992521 ) ) ;
#3597=CARTESIAN_POINT ( 'NONE',  ( 4.713407268011036227E-15, -18.77782273057287910, -10.58866585036055596 ) ) ;
#3610=CARTESIAN_POINT ( 'NONE',  ( -4.000000000000004441, -23.27007316922370350, -4.925310638870541879 ) ) ;
#3612=CARTESIAN_POINT ( 'NONE',  ( -8.999999999999996447, -10.00000000000000000, 15.14468620625656925 ) ) ;
#3614=CARTESIAN_POINT ( 'NONE',  ( 2.000000000000004441, -20.97122678548641872, -11.70801252582615604 ) ) ;
#3616=CARTESIAN_POINT ( 'NONE',  ( -4.243569643750004339, -21.72368718624651507, -2.471670375064849434 ) ) ;
#3618=CARTESIAN_POINT ( 'NONE',  ( 4.243569643750003451, -22.00086816302836823, -11.41050605784547578 ) ) ;
#3623=CARTESIAN_POINT ( 'NONE',  ( 1.287074048710447283, -10.56983422227372671, 22.11683441173062192 ) ) ;
#3626=CARTESIAN_POINT ( 'NONE',  ( -4.000000000000000888, -22.75490600406122255, -8.215893585883295103 ) ) ;
#3629=CARTESIAN_POINT ( 'NONE',  ( -8.500000000000005329, 10.00000000000000000, -22.50000000000000000 ) ) ;
#3630=EDGE_CURVE ( 'NONE', #2315, #15771, #6817, .T. ) ;
#3631=CARTESIAN_POINT ( 'NONE',  ( 2.121784821875004390, -17.58820128504952152, -7.244309707463659542 ) ) ;
#3633=VECTOR ( 'NONE', #7832, 999.9999999999998863 ) ;
#3636=CARTESIAN_POINT ( 'NONE',  ( 1.999999999999994449, -28.79739026113263023, -10.80597857277268403 ) ) ;
#3637=( BOUNDED_CURVE ( )  B_SPLINE_CURVE ( 2, ( #1951, #5233, #16566, #6534, #12364, #16038, #3847, #13763, #17539 ),
 .UNSPECIFIED., .F., .T. ) 
 B_SPLINE_CURVE_WITH_KNOTS ( ( 3, 2, 2, 2, 3 ),
 ( 0.2327586206896551657, 0.2356321839080459668, 0.2413793103448275967, 0.2471264367816091989, 0.2500000000000000000 ),
 .UNSPECIFIED. ) 
 CURVE ( )  GEOMETRIC_REPRESENTATION_ITEM ( )  RATIONAL_B_SPLINE_CURVE ( ( 0.9330127018922194093, 0.9330127018922194093, 1.000000000000000000, 0.8660254037844387076, 1.000000000000000000, 0.8660254037844387076, 1.000000000000000000, 0.9330127018922197424, 0.9330127018922194093 ) ) 
 REPRESENTATION_ITEM ( '' )  );
#3639=CARTESIAN_POINT ( 'NONE',  ( -2.121784821874996396, -18.86799370865777803, -9.072042706283481195 ) ) ;
#3645=EDGE_LOOP ( 'NONE', ( #6369, #5806 ) ) ;
#3648=CARTESIAN_POINT ( 'NONE',  ( 7.503318896749359368, -12.79558280299057316, 6.421203217138808483 ) ) ;
#3651=CARTESIAN_POINT ( 'NONE',  ( -2.121784821874996396, -23.22358977219849407, -15.29247854260303718 ) ) ;
#3653=DIRECTION ( 'NONE',  ( -0.000000000000000000, -0.5735764363510414965, -0.8191520442889950182 ) ) ;
#3654=CARTESIAN_POINT ( 'NONE',  ( 2.526502195916454863, -15.31622431267016360, -9.916727303591175158 ) ) ;
#3657=CARTESIAN_POINT ( 'NONE',  ( -2.121784821875005722, -27.90010160600482081, -9.156759261635325942 ) ) ;
#3658=EDGE_CURVE ( 'NONE', #8888, #10898, #12607, .T. ) ;
#3659=EDGE_CURVE ( 'NONE', #5080, #3510, #3737, .T. ) ;
#3660=( BOUNDED_CURVE ( )  B_SPLINE_CURVE ( 3, ( #3357, #14486, #9088, #479 ),
 .UNSPECIFIED., .F., .F. ) 
 B_SPLINE_CURVE_WITH_KNOTS ( ( 4, 4 ),
 ( 4.712388980384689674, 6.283185307179585344 ),
 .UNSPECIFIED. ) 
 CURVE ( )  GEOMETRIC_REPRESENTATION_ITEM ( )  RATIONAL_B_SPLINE_CURVE ( ( 1.000000000000000000, 0.8047378541243649375, 0.8047378541243649375, 1.000000000000000000 ) ) 
 REPRESENTATION_ITEM ( '' )  );
#3661=CARTESIAN_POINT ( 'NONE',  ( 3.798794474141382604, -25.80746198062961838, -15.42752687081247132 ) ) ;
#3663=EDGE_CURVE ( 'NONE', #1446, #5758, #15286, .T. ) ;
#3664=CARTESIAN_POINT ( 'NONE',  ( -1.999999999999996225, -23.50930251633977264, -15.33276032180496173 ) ) ;
#3666=CARTESIAN_POINT ( 'NONE',  ( 4.730628863548789710E-15, -19.14431419784869348, -11.60241431796419853 ) ) ;
#3678=CARTESIAN_POINT ( 'NONE',  ( 4.730628863548789710E-15, -18.91846847603547133, -11.27987320052540809 ) ) ;
#3680=ORIENTED_EDGE ( 'NONE', *, *, #7961, .F. ) ;
#3683=CARTESIAN_POINT ( 'NONE',  ( -2.714947574412843956, -24.61702768235999272, -16.14861449798980075 ) ) ;
#3685=CARTESIAN_POINT ( 'NONE',  ( 1.071796769724485454, -21.29659030142491005, -13.10699010444694679 ) ) ;
#3686=CARTESIAN_POINT ( 'NONE',  ( 4.243569643749996345, -21.92802379169658877, -2.763493290842798267 ) ) ;
#3687=ORIENTED_EDGE ( 'NONE', *, *, #18287, .F. ) ;
#3688=CARTESIAN_POINT ( 'NONE',  ( 3.999999999999993339, 7.428752623566170548E-15, 30.00000000000000000 ) ) ;
#3689=CARTESIAN_POINT ( 'NONE',  ( 4.713407268011036227E-15, -19.55215091964678820, -11.69452111015069917 ) ) ;
#3693=CARTESIAN_POINT ( 'NONE',  ( 4.000000000000000888, -26.23938285489380462, -13.19224225493893599 ) ) ;
#3699=CARTESIAN_POINT ( 'NONE',  ( -4.000000000000004441, -22.23763558379183181, -3.450836959150351380 ) ) ;
#3704=CARTESIAN_POINT ( 'NONE',  ( 2.769793372871041548, -22.34959508723814992, -1.882086548653339797 ) ) ;
#3705=CARTESIAN_POINT ( 'NONE',  ( 4.243569643749996345, -26.31588352978205592, -9.030006429653610667 ) ) ;
#3708=CARTESIAN_POINT ( 'NONE',  ( -4.000000000000004441, -21.72141679107589596, -2.713600119290256352 ) ) ;
#3709=DIRECTION ( 'NONE',  ( 0.000000000000000000, -0.000000000000000000, 1.000000000000000000 ) ) ;
#3710=CARTESIAN_POINT ( 'NONE',  ( -1.999999999999996225, -19.89577096732821104, -10.17210244278429343 ) ) ;
#3711=CARTESIAN_POINT ( 'NONE',  ( 4.243569643749996345, -28.89697749336173871, -12.71619062895408803 ) ) ;
#3715=CARTESIAN_POINT ( 'NONE',  ( 4.243569643749996345, -21.89576011715183768, -2.717415988351541856 ) ) ;
#3718=CARTESIAN_POINT ( 'NONE',  ( -4.000000000000004441, -26.62549532187730250, -9.717350097961160671 ) ) ;
#3721=CARTESIAN_POINT ( 'NONE',  ( 2.121784821875004390, -17.62046495959427261, -7.290387009954915953 ) ) ;
#3729=ORIENTED_EDGE ( 'NONE', *, *, #18287, .T. ) ;
#3731=FACE_OUTER_BOUND ( 'NONE', #66, .T. ) ;
#3732=CARTESIAN_POINT ( 'NONE',  ( 4.299564228933482956E-15, -19.80093457235270549, -10.97097235620001854 ) ) ;
#3735=CARTESIAN_POINT ( 'NONE',  ( 4.243569643750000786, -23.73894807732350998, -9.621251311363216985 ) ) ;
#3737=( BOUNDED_CURVE ( )  B_SPLINE_CURVE ( 2, ( #11091, #1012, #6561, #16684, #6651, #17990, #3961, #5262, #9614 ),
 .UNSPECIFIED., .F., .T. ) 
 B_SPLINE_CURVE_WITH_KNOTS ( ( 3, 2, 2, 2, 3 ),
 ( 0.8017241379310344751, 0.8045977011494253039, 0.8103448275862068506, 0.8160919540229885083, 0.8189655172413793371 ),
 .UNSPECIFIED. ) 
 CURVE ( )  GEOMETRIC_REPRESENTATION_ITEM ( )  RATIONAL_B_SPLINE_CURVE ( ( 0.9330127018922194093, 0.9330127018922194093, 1.000000000000000000, 0.8660254037844387076, 1.000000000000000000, 0.8660254037844387076, 1.000000000000000000, 0.9330127018922194093, 0.9330127018922194093 ) ) 
 REPRESENTATION_ITEM ( '' )  );
#3741=CARTESIAN_POINT ( 'NONE',  ( -5.330712181944245322E-15, -29.39828321677494216, -9.160639286973687234 ) ) ;
#3744=CARTESIAN_POINT ( 'NONE',  ( -1.071796769724486786, -23.08030267449302286, -15.65439537464544806 ) ) ;
#3747=CARTESIAN_POINT ( 'NONE',  ( -2.121784821874996396, -19.09383943047100018, -9.394583823722271632 ) ) ;
#3748=VERTEX_POINT ( 'NONE', #5718 ) ;
#3749=DIRECTION ( 'NONE',  ( -0.000000000000000000, -0.5735764363510414965, -0.8191520442889950182 ) ) ;
#3756=ADVANCED_FACE ( 'NONE', ( #7000 ), #9964, .F. ) ;
#3760=ORIENTED_EDGE ( 'NONE', *, *, #6381, .T. ) ;
#3761=CARTESIAN_POINT ( 'NONE',  ( -5.330712181944246111E-15, -25.01042347868948212, -2.894126148162874834 ) ) ;
#3763=ORIENTED_EDGE ( 'NONE', *, *, #4008, .F. ) ;
#3764=ADVANCED_FACE ( 'NONE', ( #10148 ), #11358, .F. ) ;
#3766=CARTESIAN_POINT ( 'NONE',  ( 1.998572135942813466, -24.18888450820426783, -16.52405203462232564 ) ) ;
#3767=CARTESIAN_POINT ( 'NONE',  ( 7.573138360694985138, -10.32747394560775511, 6.453217690228979286 ) ) ;
#3769=CARTESIAN_POINT ( 'NONE',  ( -4.243569643749997233, -23.94744319389470633, -14.19050330815125704 ) ) ;
#3771=DIRECTION ( 'NONE',  ( 0.000000000000000000, 0.8191520442889952403, -0.5735764363510413855 ) ) ;
#3772=CARTESIAN_POINT ( 'NONE',  ( 4.000000000000003553, -19.68015399097727069, -7.851010534249639683 ) ) ;
#3777=CARTESIAN_POINT ( 'NONE',  ( 3.579096709490575479E-14, -25.70887743576973605, -5.460814815566567226 ) ) ;
#3780=CARTESIAN_POINT ( 'NONE',  ( 4.000000000000000888, -23.59376154151967953, -9.413903449649181354 ) ) ;
#3781=EDGE_CURVE ( 'NONE', #15771, #6047, #15121, .T. ) ;
#3785=CARTESIAN_POINT ( 'NONE',  ( -2.000000000000005773, -23.42011117034160605, -3.126428157563360344 ) ) ;
#3786=ORIENTED_EDGE ( 'NONE', *, *, #15552, .T. ) ;
#3791=CARTESIAN_POINT ( 'NONE',  ( 4.243569643749997233, -21.89576011715183057, -2.717415988351541412 ) ) ;
#3792=CARTESIAN_POINT ( 'NONE',  ( -2.121784821874996396, -20.67475948316355883, -11.65237164579381535 ) ) ;
#3793=LINE ( 'NONE', #9355, #17145 ) ;
#3798=CARTESIAN_POINT ( 'NONE',  ( -4.243569643749997233, -24.23781626479742712, -14.60519903057256208 ) ) ;
#3803=CARTESIAN_POINT ( 'NONE',  ( -4.243569643749997233, -17.75281768130346194, -5.343661229830111381 ) ) ;
#3807=CARTESIAN_POINT ( 'NONE',  ( -5.279047395330986450E-15, -28.21611830590294190, -7.962677234997037168 ) ) ;
#3813=CARTESIAN_POINT ( 'NONE',  ( -2.121784821874996396, -21.67493339405068653, -13.08076802302275077 ) ) ;
#3814=AXIS2_PLACEMENT_3D ( 'NONE', #95, #10085, #3437 ) ;
#3815=CARTESIAN_POINT ( 'NONE',  ( -1.071796769724491671, -22.82219327813506737, -15.28577695471540210 ) ) ;
#3819=ORIENTED_EDGE ( 'NONE', *, *, #14291, .F. ) ;
#3823=DIRECTION ( 'NONE',  ( -6.162975822039154730E-33, 0.5735764363510414965, 0.8191520442889950182 ) ) ;
#3824=DIRECTION ( 'NONE',  ( -0.7601375407242620952, -0.6497622020259954390, 0.000000000000000000 ) ) ;
#3827=CARTESIAN_POINT ( 'NONE',  ( 4.730628863548789710E-15, -19.66053299056463288, -12.33965115782429400 ) ) ;
#3832=LINE ( 'NONE', #13561, #117 ) ;
#3836=CARTESIAN_POINT ( 'NONE',  ( 2.121784821874994176, -27.08275518420459349, -7.989467598523504854 ) ) ;
#3841=FACE_OUTER_BOUND ( 'NONE', #13740, .T. ) ;
#3843=( BOUNDED_CURVE ( )  B_SPLINE_CURVE ( 2, ( #3237, #453, #18216, #11220, #1412, #3137, #7042, #6001, #4708 ),
 .UNSPECIFIED., .F., .F. ) 
 B_SPLINE_CURVE_WITH_KNOTS ( ( 3, 2, 2, 2, 3 ),
 ( 0.6465517241379310498, 0.6494252873563218786, 0.6551724137931034253, 0.6609195402298850830, 0.6637931034482759118 ),
 .UNSPECIFIED. ) 
 CURVE ( )  GEOMETRIC_REPRESENTATION_ITEM ( )  RATIONAL_B_SPLINE_CURVE ( ( 0.9330127018922194093, 0.9330127018922194093, 1.000000000000000000, 0.8660254037844387076, 1.000000000000000000, 0.8660254037844387076, 1.000000000000000000, 0.9330127018922180770, 0.9330127018922194093 ) ) 
 REPRESENTATION_ITEM ( '' )  );
#3844=CARTESIAN_POINT ( 'NONE',  ( -4.243569643750005227, -24.56289054618417111, -6.526472994295373198 ) ) ;
#3845=ORIENTED_EDGE ( 'NONE', *, *, #4725, .T. ) ;
#3846=CARTESIAN_POINT ( 'NONE',  ( 1.533898589781675205E-14, -28.03186200299146336, -8.778380594936995962 ) ) ;
#3847=CARTESIAN_POINT ( 'NONE',  ( 2.000000000000004441, -22.32630111707070242, -13.64325923146567199 ) ) ;
#3851=CARTESIAN_POINT ( 'NONE',  ( -4.000000000000000888, -20.10928469068709745, -4.437554780593541359 ) ) ;
#3854=CARTESIAN_POINT ( 'NONE',  ( -4.243569643749998122, -18.81751894128008473, -6.864212212041559624 ) ) ;
#3858=CARTESIAN_POINT ( 'NONE',  ( 0.000000000000000000, 5.977523610840987267, 32.81826849749789687 ) ) ;
#3860=CARTESIAN_POINT ( 'NONE',  ( 0.2152313249818218199, -23.77077346268850988, -16.79000057782539201 ) ) ;
#3863=CARTESIAN_POINT ( 'NONE',  ( 4.243569643750003451, -24.54969845206331058, -15.05061295465469762 ) ) ;
#3864=EDGE_CURVE ( 'NONE', #16968, #12341, #15668, .T. ) ;
#3865=EDGE_LOOP ( 'NONE', ( #10369, #5746, #8317, #17045 ) ) ;
#3867=CARTESIAN_POINT ( 'NONE',  ( -4.000000000000004441, -23.33460051901814225, -5.017465244859820039 ) ) ;
#3868=AXIS2_PLACEMENT_3D ( 'NONE', #8631, #4473, #7243 ) ;
#3877=ORIENTED_EDGE ( 'NONE', *, *, #15787, .F. ) ;
#3878=CARTESIAN_POINT ( 'NONE',  ( 4.730628863548789710E-15, -21.49956243961516122, -14.96605739982588368 ) ) ;
#3880=CARTESIAN_POINT ( 'NONE',  ( -4.000000000000000888, -21.14172227611897270, -5.912028460313731415 ) ) ;
#3881=ORIENTED_EDGE ( 'NONE', *, *, #6478, .F. ) ;
#3882=CARTESIAN_POINT ( 'NONE',  ( -1.071796769724486786, -20.82184545706574852, -12.42898420126429748 ) ) ;
#3884=ADVANCED_FACE ( 'NONE', ( #246 ), #17266, .F. ) ;
#3886=CARTESIAN_POINT ( 'NONE',  ( 2.121784821875004390, -17.07198249233357856, -6.507072867603563182 ) ) ;
#3887=EDGE_CURVE ( 'NONE', #6155, #12907, #639, .T. ) ;
#3888=CARTESIAN_POINT ( 'NONE',  ( -4.243569643750000786, -22.09350067554145625, -7.271308884309165776 ) ) ;
#3889=EDGE_CURVE ( 'NONE', #8328, #2307, #17637, .T. ) ;
#3891=ORIENTED_EDGE ( 'NONE', *, *, #3889, .T. ) ;
#3892=CARTESIAN_POINT ( 'NONE',  ( -2.000000000000005773, -27.35627946550557255, -8.747859062503353655 ) ) ;
#3896=ORIENTED_EDGE ( 'NONE', *, *, #12152, .T. ) ;
#3900=CARTESIAN_POINT ( 'NONE',  ( -2.000000000000005773, -29.67926403272728919, -12.06542484187378506 ) ) ;
#3903=CARTESIAN_POINT ( 'NONE',  ( -1.999999999999996225, -21.96064613819196154, -13.12104980222467532 ) ) ;
#3905=CARTESIAN_POINT ( 'NONE',  ( 0.000000000000000000, -3.999999999999991562, 11.59510085796834566 ) ) ;
#3907=DIRECTION ( 'NONE',  ( 0.000000000000000000, 0.000000000000000000, 1.000000000000000000 ) ) ;
#3908=CARTESIAN_POINT ( 'NONE',  ( -4.243569643750000786, -23.86800277550248950, -9.805560521328242629 ) ) ;
#3909=CARTESIAN_POINT ( 'NONE',  ( -1.999999999999996225, -17.83089579646446410, -7.223155083343911542 ) ) ;
#3917=CARTESIAN_POINT ( 'NONE',  ( 1.071796769724476128, -18.26380489492371595, -8.775723671275654780 ) ) ;
#3918=DIRECTION ( 'NONE',  ( -0.5735764363510413855, 0.6710100716628397688, -0.4698463103929523266 ) ) ;
#3921=CARTESIAN_POINT ( 'NONE',  ( 4.730628863548789710E-15, -20.69297057599650813, -13.81412483754448495 ) ) ;
#3925=CARTESIAN_POINT ( 'NONE',  ( 8.500000000000019540, -1.201721234452885367, 20.49999999999998934 ) ) ;
#3927=CARTESIAN_POINT ( 'NONE',  ( 4.243569643750003451, -21.74275876667039853, -11.04188763791542804 ) ) ;
#3932=CYLINDRICAL_SURFACE ( 'NONE', #17506, 6.000000000000000000 ) ;
#3934=CARTESIAN_POINT ( 'NONE',  ( 4.730628863548789710E-15, -17.85376721605885209, -9.759322218313958075 ) ) ;
#3935=EDGE_CURVE ( 'NONE', #5777, #8773, #1829, .T. ) ;
#3941=CARTESIAN_POINT ( 'NONE',  ( -1.071796769724481457, -22.04786508906114761, -14.17992169492525889 ) ) ;
#3942=VECTOR ( 'NONE', #13951, 1000.000000000000000 ) ;
#3946=ORIENTED_EDGE ( 'NONE', *, *, #9880, .T. ) ;
#3947=CARTESIAN_POINT ( 'NONE',  ( 4.243569643749997233, -23.73478956620236957, -5.343822230353133307 ) ) ;
#3950=CARTESIAN_POINT ( 'NONE',  ( -4.243569643749998122, -24.46366198661065283, -14.92774014801135074 ) ) ;
#3952=CARTESIAN_POINT ( 'NONE',  ( 3.064183985264992582, -21.85725672082847382, -2.451266466499125052 ) ) ;
#3954=CARTESIAN_POINT ( 'NONE',  ( -2.000000000000005773, -23.67822056669957576, -3.495046577493408968 ) ) ;
#3955=CARTESIAN_POINT ( 'NONE',  ( 4.243569643750003451, -24.29158905570534088, -14.68199453472465166 ) ) ;
#3958=CARTESIAN_POINT ( 'NONE',  ( 4.000000000000000888, -21.07719492773443193, -5.819873856337981266 ) ) ;
#3961=CARTESIAN_POINT ( 'NONE',  ( -2.000000000000005773, -23.93632996305754190, -3.863664997423455816 ) ) ;
#3967=ORIENTED_EDGE ( 'NONE', *, *, #4289, .F. ) ;
#3968=CARTESIAN_POINT ( 'NONE',  ( -4.243569643750000786, -24.93270403547910874, -11.32611150353969087 ) ) ;
#3970=CARTESIAN_POINT ( 'NONE',  ( 4.000000000000000888, -20.75455818158202703, -5.359100830418656258 ) ) ;
#3971=EDGE_LOOP ( 'NONE', ( #17487, #15706, #12869, #4193 ) ) ;
#3973=DIRECTION ( 'NONE',  ( 1.000000000000000000, 0.000000000000000000, 0.000000000000000000 ) ) ;
#3975=CARTESIAN_POINT ( 'NONE',  ( 4.243569643749996345, -24.76722715163424127, -6.818295910073324251 ) ) ;
#3979=EDGE_LOOP ( 'NONE', ( #12829, #8789, #9971, #13310, #18277, #15752, #7206, #3877, #1962 ) ) ;
#3980=CARTESIAN_POINT ( 'NONE',  ( -1.999999999999996225, -20.99273590255452149, -11.73873072849375987 ) ) ;
#3981=AXIS2_PLACEMENT_3D ( 'NONE', #8262, #18122, #18297 ) ;
#3982=CARTESIAN_POINT ( 'NONE',  ( 4.000000000000000888, -25.14241791966749417, -11.62561396922946777 ) ) ;
#3983=DIRECTION ( 'NONE',  ( 0.000000000000000000, 0.000000000000000000, -1.000000000000000000 ) ) ;
#3987=CARTESIAN_POINT ( 'NONE',  ( 2.121784821875004390, -17.33009188869154826, -6.875691287533610918 ) ) ;
#3993=CARTESIAN_POINT ( 'NONE',  ( -2.000000000000005773, -27.80797090842707320, -9.392941296374171856 ) ) ;
#3996=CARTESIAN_POINT ( 'NONE',  ( 2.121784821875004390, -16.84613677052036351, -6.184531750164772745 ) ) ;
#3999=EDGE_CURVE ( 'NONE', #16392, #8328, #17022, .T. ) ;
#4000=CARTESIAN_POINT ( 'NONE',  ( -4.243569643749998122, -20.85013043759908413, -9.767082268990684213 ) ) ;
#4001=CARTESIAN_POINT ( 'NONE',  ( -4.000000000000004441, -27.91604230366714390, -11.56044219761139935 ) ) ;
#4008=EDGE_CURVE ( 'NONE', #16065, #5051, #8115, .T. ) ;
#4009=CARTESIAN_POINT ( 'NONE',  ( -4.000000000000004441, -23.78629196193964646, -5.662547478730638240 ) ) ;
#4011=FACE_OUTER_BOUND ( 'NONE', #1462, .T. ) ;
#4014=CARTESIAN_POINT ( 'NONE',  ( -4.243569643750000786, -24.38422156821842535, -10.54279736118833988 ) ) ;
#4017=FACE_OUTER_BOUND ( 'NONE', #7449, .T. ) ;
#4018=VECTOR ( 'NONE', #5589, 1000.000000000000000 ) ;
#4019=CARTESIAN_POINT ( 'NONE',  ( -4.243569643750000786, -24.15837584640520674, -10.22025624374954766 ) ) ;
#4023=CARTESIAN_POINT ( 'NONE',  ( 2.121784821875004390, -18.62063887048139321, -8.718783387183849598 ) ) ;
#4025=CARTESIAN_POINT ( 'NONE',  ( -4.000000000000000888, -21.98057781498731345, -7.110038326093152783 ) ) ;
#4030=CARTESIAN_POINT ( 'NONE',  ( -4.000000000000004441, -27.14171411459323835, -10.45458693782125792 ) ) ;
#4033=CARTESIAN_POINT ( 'NONE',  ( 4.243569643750000786, -21.70633658100450702, -6.718381254414091508 ) ) ;
#4036=CARTESIAN_POINT ( 'NONE',  ( 2.121784821875004390, -24.04093619399873560, -16.45977020571485028 ) ) ;
#4039=CARTESIAN_POINT ( 'NONE',  ( 2.121784821875004390, -22.75038921220889065, -14.61667810606461337 ) ) ;
#4041=CARTESIAN_POINT ( 'NONE',  ( 1.999999999999994449, -24.47405787284159828, -4.631620039951150680 ) ) ;
#4045=ADVANCED_FACE ( 'NONE', ( #6174 ), #13312, .F. ) ;
#4051=CARTESIAN_POINT ( 'NONE',  ( 2.121784821875004390, -22.26643409403770590, -13.92551856869577342 ) ) ;
#4053=EDGE_CURVE ( 'NONE', #10497, #7716, #9524, .T. ) ;
#4054=CARTESIAN_POINT ( 'NONE',  ( 2.000000000000004441, -17.09958584011689098, -6.178736226875440884 ) ) ;
#4055=ORIENTED_EDGE ( 'NONE', *, *, #4008, .T. ) ;
#4056=CARTESIAN_POINT ( 'NONE',  ( -2.000000000000005773, -24.45254875577348130, -4.600901837283550400 ) ) ;
#4057=EDGE_CURVE ( 'NONE', #5987, #6584, #6922, .T. ) ;
#4060=AXIS2_PLACEMENT_3D ( 'NONE', #17916, #2335, #5185 ) ;
#4063=CARTESIAN_POINT ( 'NONE',  ( 4.243569643750000786, -22.73877416643638227, -8.192854934134281564 ) ) ;
#4066=VERTEX_POINT ( 'NONE', #2568 ) ;
#4067=CARTESIAN_POINT ( 'NONE',  ( -3.999999999999997335, -23.20764907453616743, -12.88879560662696200 ) ) ;
#4068=DIRECTION ( 'NONE',  ( -0.000000000000000000, -0.5735764363510414965, -0.8191520442889950182 ) ) ;
#4070=CARTESIAN_POINT ( 'NONE',  ( 4.299564228933482956E-15, -22.57561058249592278, -14.93362036944126814 ) ) ;
#4074=CARTESIAN_POINT ( 'NONE',  ( -4.000000000000000888, -25.59410936399887504, -12.27069620511382197 ) ) ;
#4079=CARTESIAN_POINT ( 'NONE',  ( -4.000000000000000888, -25.27147261784647014, -11.80992317919449519 ) ) ;
#4081=CARTESIAN_POINT ( 'NONE',  ( -4.243569643749997233, -18.04319075220617563, -5.758356952251413752 ) ) ;
#4084=CARTESIAN_POINT ( 'NONE',  ( -5.330712181944246111E-15, -26.26870678593456887, -4.691140945321855327 ) ) ;
#4088=CARTESIAN_POINT ( 'NONE',  ( -3.706921591972381904E-14, -17.67153205169451624, -7.929870390770359379 ) ) ;
#4096=CARTESIAN_POINT ( 'NONE',  ( -5.577813053751546416E-15, -25.19265864305380376, -4.723577975706471754 ) ) ;
#4098=DIRECTION ( 'NONE',  ( -0.000000000000000000, -0.5735764363510414965, -0.8191520442889950182 ) ) ;
#4101=CARTESIAN_POINT ( 'NONE',  ( 4.730628863548789710E-15, -20.17675178328056873, -13.07688799768438948 ) ) ;
#4105=DIRECTION ( 'NONE',  ( 0.000000000000000000, 0.8191520442889952403, -0.5735764363510413855 ) ) ;
#4107=CARTESIAN_POINT ( 'NONE',  ( 4.730628863548789710E-15, -19.95090606146734658, -12.75434688024559726 ) ) ;
#4110=( BOUNDED_CURVE ( )  B_SPLINE_CURVE ( 2, ( #14202, #18309, #5581, #16915, #9923, #6786, #12713, #8273, #4192 ),
 .UNSPECIFIED., .F., .T. ) 
 B_SPLINE_CURVE_WITH_KNOTS ( ( 3, 2, 2, 2, 3 ),
 ( 0.5431034482758620996, 0.5459770114942529284, 0.5517241379310344751, 0.5574712643678161328, 0.5603448275862069616 ),
 .UNSPECIFIED. ) 
 CURVE ( )  GEOMETRIC_REPRESENTATION_ITEM ( )  RATIONAL_B_SPLINE_CURVE ( ( 0.9330127018922194093, 0.9330127018922194093, 1.000000000000000000, 0.8660254037844387076, 1.000000000000000000, 0.8660254037844387076, 1.000000000000000000, 0.9330127018922180770, 0.9330127018922194093 ) ) 
 REPRESENTATION_ITEM ( '' )  );
#4113=EDGE_CURVE ( 'NONE', #9296, #12103, #2559, .T. ) ;
#4114=DIRECTION ( 'NONE',  ( -0.000000000000000000, -0.5735764363510414965, -0.8191520442889950182 ) ) ;
#4116=DIRECTION ( 'NONE',  ( 0.000000000000000000, 0.000000000000000000, 1.000000000000000000 ) ) ;
#4117=CARTESIAN_POINT ( 'NONE',  ( -4.243569643750000786, -21.80312760463873900, -6.856613161887861629 ) ) ;
#4118=CYLINDRICAL_SURFACE ( 'NONE', #11509, 4.000000000000000000 ) ;
#4119=FACE_BOUND ( 'NONE', #9018, .T. ) ;
#4120=VECTOR ( 'NONE', #8235, 1000.000000000000000 ) ;
#4122=VECTOR ( 'NONE', #16053, 1000.000000000000000 ) ;
#4123=CARTESIAN_POINT ( 'NONE',  ( 4.299564228933482956E-15, -19.22018842984233089, -10.14158091035064579 ) ) ;
#4125=CARTESIAN_POINT ( 'NONE',  ( -5.577813053751546416E-15, -29.06429958842333505, -10.25285427465718868 ) ) ;
#4127=ORIENTED_EDGE ( 'NONE', *, *, #2592, .T. ) ;
#4129=CARTESIAN_POINT ( 'NONE',  ( 4.730628863548789710E-15, -17.88603089060359963, -9.805399520805213598 ) ) ;
#4136=DIRECTION ( 'NONE',  ( 0.7601375407242620952, 0.6497622020259954390, 0.000000000000000000 ) ) ;
#4137=CARTESIAN_POINT ( 'NONE',  ( -4.243569643750000786, -26.44909673908217584, -13.49174472062871999 ) ) ;
#4138=ORIENTED_EDGE ( 'NONE', *, *, #15552, .F. ) ;
#4139=CARTESIAN_POINT ( 'NONE',  ( -1.661723472263481630E-14, -20.25262601527420969, -11.61605459007084029 ) ) ;
#4140=CARTESIAN_POINT ( 'NONE',  ( 2.000000000000004441, -18.97087896441710697, -8.851219772375051420 ) ) ;
#4146=AXIS2_PLACEMENT_3D ( 'NONE', #4677, #2105, #7733 ) ;
#4151=CARTESIAN_POINT ( 'NONE',  ( -2.121784821874996396, -22.73963465402730577, -14.60131900523419901 ) ) ;
#4154=CYLINDRICAL_SURFACE ( 'NONE', #288, 4.000000000000000000 ) ;
#4159=CARTESIAN_POINT ( 'NONE',  ( -4.243569643750005227, -24.59515422072892221, -6.572550296786629609 ) ) ;
#4166=CARTESIAN_POINT ( 'NONE',  ( -4.000000000000004441, -26.43191327531376800, -9.440886284020393759 ) ) ;
#4172=CARTESIAN_POINT ( 'NONE',  ( 4.713407268011036227E-15, -21.87513548686850129, -15.01208688952113057 ) ) ;
#4176=CARTESIAN_POINT ( 'NONE',  ( -2.000000000000005773, -26.51742392663723180, -7.549849196723933176 ) ) ;
#4178=LINE ( 'NONE', #17267, #15953 ) ;
#4180=CARTESIAN_POINT ( 'NONE',  ( 2.121784821874994176, -26.01805392422797070, -6.468916616312057499 ) ) ;
#4181=COLOUR_RGB ( '',0.8941176470588234615, 0.8941176470588234615, 0.8941176470588234615 ) ;
#4183=CARTESIAN_POINT ( 'NONE',  ( 0.000000000000000000, 9.254131787996968228, 30.52396275209373044 ) ) ;
#4184=DIRECTION ( 'NONE',  ( -0.000000000000000000, -0.000000000000000000, 1.000000000000000000 ) ) ;
#4187=ORIENTED_EDGE ( 'NONE', *, *, #3565, .F. ) ;
#4189=FACE_OUTER_BOUND ( 'NONE', #11845, .T. ) ;
#4190=CARTESIAN_POINT ( 'NONE',  ( -1.071796769724486786, -22.88672062792949546, -15.37793156070467582 ) ) ;
#4191=CARTESIAN_POINT ( 'NONE',  ( 4.000000000000003553, -19.16393519826133485, -7.113773694389544211 ) ) ;
#4192=CARTESIAN_POINT ( 'NONE',  ( -3.706921591972381904E-14, -19.54282517599473579, -10.60235393626997080 ) ) ;
#4193=ORIENTED_EDGE ( 'NONE', *, *, #17852, .F. ) ;
#4195=CARTESIAN_POINT ( 'NONE',  ( 4.243569643750003451, -20.93616690305174544, -9.889955075634029313 ) ) ;
#4201=CARTESIAN_POINT ( 'NONE',  ( 4.243569643750003451, -22.25897755938633793, -11.77912447777552352 ) ) ;
#4202=CARTESIAN_POINT ( 'NONE',  ( -0.3217809247881409651, -15.45745613286858422, -10.86990606519723279 ) ) ;
#4203=VECTOR ( 'NONE', #11705, 999.9999999999998863 ) ;
#4207=CARTESIAN_POINT ( 'NONE',  ( -4.243569643749997233, -18.01092707766142809, -5.712279649760157341 ) ) ;
#4208=DIRECTION ( 'NONE',  ( 0.000000000000000000, 0.8191520442889952403, -0.5735764363510413855 ) ) ;
#4209=ORIENTED_EDGE ( 'NONE', *, *, #13852, .T. ) ;
#4211=CARTESIAN_POINT ( 'NONE',  ( 2.121784821874994176, -29.37347607688156259, -11.26095607540267807 ) ) ;
#4216=ORIENTED_EDGE ( 'NONE', *, *, #17333, .F. ) ;
#4218=CARTESIAN_POINT ( 'NONE',  ( -5.330712181944246111E-15, -23.71987649689963362, -1.051034048512634156 ) ) ;
#4222=( BOUNDED_CURVE ( )  B_SPLINE_CURVE ( 2, ( #14259, #2951, #6086, #1751, #7475, #10349, #8584, #7198, #17341 ),
 .UNSPECIFIED., .F., .F. ) 
 B_SPLINE_CURVE_WITH_KNOTS ( ( 3, 2, 2, 2, 3 ),
 ( 0.5948275862068965747, 0.5977011494252874035, 0.6034482758620689502, 0.6091954022988506079, 0.6120689655172414367 ),
 .UNSPECIFIED. ) 
 CURVE ( )  GEOMETRIC_REPRESENTATION_ITEM ( )  RATIONAL_B_SPLINE_CURVE ( ( 0.9330127018922194093, 0.9330127018922194093, 1.000000000000000000, 0.8660254037844387076, 1.000000000000000000, 0.8660254037844387076, 1.000000000000000000, 0.9330127018922180770, 0.9330127018922194093 ) ) 
 REPRESENTATION_ITEM ( '' )  );
#4223=EDGE_CURVE ( 'NONE', #5777, #9873, #9773, .T. ) ;
#4224=CARTESIAN_POINT ( 'NONE',  ( 8.500000000000019540, 0.000000000000000000, 20.49999999999998934 ) ) ;
#4227=CARTESIAN_POINT ( 'NONE',  ( -8.999999999999996447, -4.000000000000000000, 30.00000000000000000 ) ) ;
#4229=CARTESIAN_POINT ( 'NONE',  ( -4.243569643750005227, -26.88587511340589131, -9.844038773665802822 ) ) ;
#4230=ORIENTED_EDGE ( 'NONE', *, *, #1117, .F. ) ;
#4233=CARTESIAN_POINT ( 'NONE',  ( 2.000000000000004441, -18.19655077534320498, -7.745364512584909988 ) ) ;
#4242=ORIENTED_EDGE ( 'NONE', *, *, #6216, .F. ) ;
#4243=CARTESIAN_POINT ( 'NONE',  ( 4.243569643750003451, -23.29141514481821318, -13.25359815749571268 ) ) ;
#4246=VECTOR ( 'NONE', #4876, 1000.000000000000000 ) ;
#4247=FACE_OUTER_BOUND ( 'NONE', #14267, .T. ) ;
#4250=CARTESIAN_POINT ( 'NONE',  ( 4.243569643750003451, -20.71032118123852683, -9.567413958195238877 ) ) ;
#4254=CARTESIAN_POINT ( 'NONE',  ( 1.999999999999994449, -27.57137062913722048, -9.055041079111724400 ) ) ;
#4257=DIRECTION ( 'NONE',  ( -0.000000000000000000, 1.000000000000000000, -0.000000000000000000 ) ) ;
#4261=CARTESIAN_POINT ( 'NONE',  ( -2.000000000000005773, -28.90493584365338720, -10.95956958208364007 ) ) ;
#4265=CARTESIAN_POINT ( 'NONE',  ( 3.999999999999996447, -25.76513066735074986, -8.488622031527665257 ) ) ;
#4269=CARTESIAN_POINT ( 'NONE',  ( 9.993653656444104527, -9.917152142463184106, 4.126537876780505876 ) ) ;
#4270=CARTESIAN_POINT ( 'NONE',  ( 4.243569643750000786, -22.70651049189163828, -8.146777631643026041 ) ) ;
#4272=CARTESIAN_POINT ( 'NONE',  ( -1.999999999999996225, -17.12109495718499375, -6.209454429543042941 ) ) ;
#4273=CARTESIAN_POINT ( 'NONE',  ( 3.579096709490575479E-14, -26.48320562484364871, -6.566670075356708658 ) ) ;
#4279=CARTESIAN_POINT ( 'NONE',  ( 3.579096709490575479E-14, -24.41833045397989821, -3.617722715916328546 ) ) ;
#4281=VERTEX_POINT ( 'NONE', #6126 ) ;
#4283=CARTESIAN_POINT ( 'NONE',  ( -2.121784821874996396, -20.38438641226084158, -11.23767592337251209 ) ) ;
#4287=CARTESIAN_POINT ( 'NONE',  ( -8.999999999999996447, -4.000000000000000000, -30.00000000000000000 ) ) ;
#4288=CARTESIAN_POINT ( 'NONE',  ( -2.121784821875005722, -25.06089824606716476, -5.101956642404802622 ) ) ;
#4289=EDGE_CURVE ( 'NONE', #7899, #1548, #16098, .T. ) ;
#4292=CYLINDRICAL_SURFACE ( 'NONE', #10302, 2.000000000000001776 ) ;
#4293=CARTESIAN_POINT ( 'NONE',  ( -4.243569643750005227, -22.23990597896245447, -3.208907214924944462 ) ) ;
#4298=CARTESIAN_POINT ( 'NONE',  ( 4.243569643750003451, -24.29158905570534088, -14.68199453472465166 ) ) ;
#4301=FACE_OUTER_BOUND ( 'NONE', #961, .T. ) ;
#4302=ORIENTED_EDGE ( 'NONE', *, *, #2083, .F. ) ;
#4303=CARTESIAN_POINT ( 'NONE',  ( 2.121784821874994176, -23.46922363519303190, -2.828809719502837439 ) ) ;
#4306=CARTESIAN_POINT ( 'NONE',  ( -5.330712181944246111E-15, -29.36601954223019462, -9.114561984482429935 ) ) ;
#4308=CARTESIAN_POINT ( 'NONE',  ( -3.706921591972381904E-14, -18.25227819420489439, -8.759261836619732122 ) ) ;
#4309=DIRECTION ( 'NONE',  ( -0.000000000000000000, -0.5735764363510414965, -0.8191520442889950182 ) ) ;
#4311=CARTESIAN_POINT ( 'NONE',  ( 4.730628863548789710E-15, -21.20918936871244043, -14.55136167740457864 ) ) ;
#4313=CARTESIAN_POINT ( 'NONE',  ( -3.999999999999997335, -21.85257474295189084, -10.95354890098744605 ) ) ;
#4314=CARTESIAN_POINT ( 'NONE',  ( -4.000000000000004441, -22.81838172630220996, -4.280228404999725456 ) ) ;
#4320=CARTESIAN_POINT ( 'NONE',  ( -4.000000000000004441, -24.88325689716596045, -7.229175764440105567 ) ) ;
#4323=ORIENTED_EDGE ( 'NONE', *, *, #7727, .F. ) ;
#4324=CARTESIAN_POINT ( 'NONE',  ( -4.243569643749998122, -21.91483169757570693, -11.28763325120213068 ) ) ;
#4330=CARTESIAN_POINT ( 'NONE',  ( 4.299564228933482956E-15, -18.70396963712639504, -9.404344070490550322 ) ) ;
#4333=CARTESIAN_POINT ( 'NONE',  ( 4.730628863548789710E-15, -17.11170270152969053, -8.699544261015072166 ) ) ;
#4334=VERTEX_POINT ( 'NONE', #10293 ) ;
#4335=CARTESIAN_POINT ( 'NONE',  ( 1.999999999999994449, -25.95818690119497418, -6.751175953542158936 ) ) ;
#4339=ORIENTED_EDGE ( 'NONE', *, *, #2858, .F. ) ;
#4340=CARTESIAN_POINT ( 'NONE',  ( -3.999999999999997335, -23.91744991381563779, -13.90249626042782971 ) ) ;
#4345=VERTEX_POINT ( 'NONE', #8378 ) ;
#4347=CARTESIAN_POINT ( 'NONE',  ( 3.999999999999996447, -24.99080247827684431, -7.382766771737521161 ) ) ;
#4348=ORIENTED_EDGE ( 'NONE', *, *, #13687, .F. ) ;
#4349=DIRECTION ( 'NONE',  ( -0.000000000000000000, -0.5735764363510414965, -0.8191520442889950182 ) ) ;
#4352=CARTESIAN_POINT ( 'NONE',  ( -6.737340654859749201, -10.37508571686348269, 2.119921479756860183 ) ) ;
#4353=CARTESIAN_POINT ( 'NONE',  ( 4.243569643750000786, -23.48083868096554028, -9.252632891433169249 ) ) ;
#4354=EDGE_CURVE ( 'NONE', #5641, #11442, #7518, .T. ) ;
#4357=ORIENTED_EDGE ( 'NONE', *, *, #1795, .T. ) ;
#4358=EDGE_LOOP ( 'NONE', ( #826, #781, #10153, #5732 ) ) ;
#4360=CARTESIAN_POINT ( 'NONE',  ( 6.428571428571432378, -14.26578344203647752, -2.827263138854379410 ) ) ;
#4361=CARTESIAN_POINT ( 'NONE',  ( -2.000000000000005773, -29.67926403272728919, -12.06542484187378506 ) ) ;
#4366=CARTESIAN_POINT ( 'NONE',  ( -4.243569643750005227, -24.30478114982620497, -6.157854574365327238 ) ) ;
#4370=LINE ( 'NONE', #116, #11715 ) ;
#4371=CARTESIAN_POINT ( 'NONE',  ( 4.243569643749996345, -25.28344594435018067, -7.555532749933418835 ) ) ;
#4374=AXIS2_PLACEMENT_3D ( 'NONE', #12071, #3918, #3824 ) ;
#4375=EDGE_CURVE ( 'NONE', #12399, #16719, #13805, .T. ) ;
#4377=CARTESIAN_POINT ( 'NONE',  ( 0.9156706748228305992, -9.999999999999090505, -4.445527249942534453 ) ) ;
#4381=CARTESIAN_POINT ( 'NONE',  ( -2.121784821874996396, -18.06140184503912494, -7.920110144002082464 ) ) ;
#4382=EDGE_CURVE ( 'NONE', #10740, #16544, #11408, .T. ) ;
#4383=DIRECTION ( 'NONE',  ( 0.000000000000000000, 0.000000000000000000, -1.000000000000000000 ) ) ;
#4396=EDGE_LOOP ( 'NONE', ( #6000, #5261, #9338, #7412 ) ) ;
#4397=CARTESIAN_POINT ( 'NONE',  ( -2.121784821874996396, -17.06122793415199723, -6.491713766773147931 ) ) ;
#4399=CARTESIAN_POINT ( 'NONE',  ( -2.121784821874996396, -23.77207223945918457, -16.07579268495438996 ) ) ;
#4401=CARTESIAN_POINT ( 'NONE',  ( -4.243569643750000786, -25.15854975729233090, -11.64865262097848309 ) ) ;
#4402=FACE_OUTER_BOUND ( 'NONE', #14788, .T. ) ;
#4405=CARTESIAN_POINT ( 'NONE',  ( 8.500000000000019540, 0.000000000000000000, 20.49999999999998934 ) ) ;
#4406=CARTESIAN_POINT ( 'NONE',  ( 4.243569643749996345, -27.05794804431121037, -10.08978438695249835 ) ) ;
#4407=FACE_OUTER_BOUND ( 'NONE', #9797, .T. ) ;
#4408=CARTESIAN_POINT ( 'NONE',  ( 4.000000000000000888, -20.81908553137646578, -5.451255436407934418 ) ) ;
#4410=ORIENTED_EDGE ( 'NONE', *, *, #103, .F. ) ;
#4417=CARTESIAN_POINT ( 'NONE',  ( 4.243569643750003451, -22.77519635210228088, -12.51636131763561721 ) ) ;
#4418=VECTOR ( 'NONE', #12468, 1000.000000000000000 ) ;
#4420=ORIENTED_EDGE ( 'NONE', *, *, #10628, .T. ) ;
#4421=FACE_OUTER_BOUND ( 'NONE', #8555, .T. ) ;
#4422=CARTESIAN_POINT ( 'NONE',  ( 1.071796769724495224, -19.48982452691913636, -10.52666116493661086 ) ) ;
#4424=CARTESIAN_POINT ( 'NONE',  ( 4.000000000000003553, -20.13184543389877490, -8.496092768120460548 ) ) ;
#4427=CARTESIAN_POINT ( 'NONE',  ( -5.330712181944245322E-15, -24.75231408233150887, -2.525507728232826210 ) ) ;
#4430=CYLINDRICAL_SURFACE ( 'NONE', #15624, 4.000000000000000000 ) ;
#4434=( BOUNDED_CURVE ( )  B_SPLINE_CURVE ( 2, ( #12856, #163, #5814, #10162, #9891, #4424, #7108, #3132, #4330 ),
 .UNSPECIFIED., .F., .T. ) 
 B_SPLINE_CURVE_WITH_KNOTS ( ( 3, 2, 2, 2, 3 ),
 ( 0.6810344827586206629, 0.6839080459770114917, 0.6896551724137931494, 0.6954022988505746961, 0.6982758620689655249 ),
 .UNSPECIFIED. ) 
 CURVE ( )  GEOMETRIC_REPRESENTATION_ITEM ( )  RATIONAL_B_SPLINE_CURVE ( ( 0.9330127018922194093, 0.9330127018922194093, 1.000000000000000000, 0.8660254037844387076, 1.000000000000000000, 0.8660254037844387076, 1.000000000000000000, 0.9330127018922194093, 0.9330127018922194093 ) ) 
 REPRESENTATION_ITEM ( '' )  );
#4442=CARTESIAN_POINT ( 'NONE',  ( 1.999999999999994449, -25.70007750483700448, -6.382557533612111200 ) ) ;
#4443=ORIENTED_EDGE ( 'NONE', *, *, #3201, .F. ) ;
#4444=EDGE_CURVE ( 'NONE', #16218, #16968, #9312, .T. ) ;
#4445=CIRCLE ( 'NONE', #3868, 4.400000000000001243 ) ;
#4449=CARTESIAN_POINT ( 'NONE',  ( -7.191589934391295458, -10.00000000000000178, 14.52136967842656645 ) ) ;
#4450=EDGE_CURVE ( 'NONE', #7294, #985, #16986, .T. ) ;
#4451=CARTESIAN_POINT ( 'NONE',  ( 2.121784821875004390, -18.62063887048139321, -8.718783387183849598 ) ) ;
#4458=CARTESIAN_POINT ( 'NONE',  ( -4.000000000000003553, 6.938893903907228378E-15, 24.28148006742132026 ) ) ;
#4460=CARTESIAN_POINT ( 'NONE',  ( -4.000000000000004441, -23.33460051901814580, -5.017465244859820039 ) ) ;
#4463=CARTESIAN_POINT ( 'NONE',  ( -4.000000000000004441, -28.23867904981954524, -12.02121522353072969 ) ) ;
#4464=CARTESIAN_POINT ( 'NONE',  ( -4.243569643749997233, -20.85013043759908413, -9.767082268990684213 ) ) ;
#4467=CARTESIAN_POINT ( 'NONE',  ( -4.000000000000004441, -23.07649112266017966, -4.648846824929771415 ) ) ;
#4468=CARTESIAN_POINT ( 'NONE',  ( 4.000000000000003553, -23.03557614363086259, -12.64304999334026114 ) ) ;
#4469=CARTESIAN_POINT ( 'NONE',  ( 4.243569643749996345, -24.76722715163424127, -6.818295910073324251 ) ) ;
#4472=CARTESIAN_POINT ( 'NONE',  ( -3.049298716197739623, -9.999999999999399591, -3.862741893372402036 ) ) ;
#4473=DIRECTION ( 'NONE',  ( 6.162975822039154730E-33, -0.5735764363510414965, -0.8191520442889950182 ) ) ;
#4474=CARTESIAN_POINT ( 'NONE',  ( -1.999999999999996225, -21.96064613819196154, -13.12104980222467532 ) ) ;
#4475=CARTESIAN_POINT ( 'NONE',  ( -4.243569643750005227, -23.01423416803636002, -4.314762474715088558 ) ) ;
#4482=CARTESIAN_POINT ( 'NONE',  ( -14.99999999999999645, -10.00000000000000000, -30.00000000000000000 ) ) ;
#4487=ORIENTED_EDGE ( 'NONE', *, *, #2542, .F. ) ;
#4488=CARTESIAN_POINT ( 'NONE',  ( -4.243569643750000786, -20.28673490103567545, -4.690979944798832513 ) ) ;
#4490=CARTESIAN_POINT ( 'NONE',  ( -5.330712181944245322E-15, -30.68883019856478711, -11.00373138662392236 ) ) ;
#4492=DIRECTION ( 'NONE',  ( -0.000000000000000000, 1.000000000000000000, -0.000000000000000000 ) ) ;
#4493=CARTESIAN_POINT ( 'NONE',  ( 2.121784821875004390, -22.23417041949295481, -13.87944126620451790 ) ) ;
#4499=CARTESIAN_POINT ( 'NONE',  ( 4.730628863548789710E-15, -20.43486117963853843, -13.44550641761443366 ) ) ;
#4501=CARTESIAN_POINT ( 'NONE',  ( -3.999999999999997335, -19.07789873280867354, -6.990900887746200887 ) ) ;
#4505=CARTESIAN_POINT ( 'NONE',  ( -2.000000000000005773, -25.03329489828385590, -5.430293283132924032 ) ) ;
#4511=CARTESIAN_POINT ( 'NONE',  ( -5.330712181944246111E-15, -27.84962683862713106, -6.948928767393399042 ) ) ;
#4513=ORIENTED_EDGE ( 'NONE', *, *, #560, .F. ) ;
#4517=CARTESIAN_POINT ( 'NONE',  ( -2.121784821875005722, -28.67442979507872636, -10.26261452142547093 ) ) ;
#4518=CARTESIAN_POINT ( 'NONE',  ( -4.000000000000007105, 6.938893903907228378E-15, -30.00000000000000000 ) ) ;
#4523=CARTESIAN_POINT ( 'NONE',  ( -4.243569643749997233, -19.33373773399602058, -7.601449051901653320 ) ) ;
#4528=ORIENTED_EDGE ( 'NONE', *, *, #17577, .F. ) ;
#4529=CARTESIAN_POINT ( 'NONE',  ( 1.533898589781675205E-14, -27.51564321027552040, -8.041143755076902266 ) ) ;
#4535=VERTEX_POINT ( 'NONE', #6320 ) ;
#4537=VECTOR ( 'NONE', #13445, 1000.000000000000000 ) ;
#4538=CARTESIAN_POINT ( 'NONE',  ( 1.999999999999994449, -25.95818690119497418, -6.751175953542158936 ) ) ;
#4539=ORIENTED_EDGE ( 'NONE', *, *, #16322, .T. ) ;
#4542=CARTESIAN_POINT ( 'NONE',  ( -7.472465112787439523, -13.11650584547975917, 4.294891433530912295 ) ) ;
#4543=CARTESIAN_POINT ( 'NONE',  ( -5.330712181944246111E-15, -25.23626920050269717, -3.216667265601667047 ) ) ;
#4548=VERTEX_POINT ( 'NONE', #3629 ) ;
#4550=CARTESIAN_POINT ( 'NONE',  ( -1.999999999999996225, -20.41198976004415044, -10.90933928264438890 ) ) ;
#4553=EDGE_LOOP ( 'NONE', ( #16641, #3896 ) ) ;
#4556=DIRECTION ( 'NONE',  ( 0.000000000000000000, 0.5150380737757255245, 0.8571673013836856869 ) ) ;
#4557=CARTESIAN_POINT ( 'NONE',  ( 2.121784821874994176, -24.21128814972218990, -3.888587676801722903 ) ) ;
#4561=CARTESIAN_POINT ( 'NONE',  ( 1.999999999999994449, -29.82982784656450193, -12.28045225249287675 ) ) ;
#4563=CARTESIAN_POINT ( 'NONE',  ( -4.243569643750000786, -22.86782886461536179, -8.377164144099308984 ) ) ;
#4564=CARTESIAN_POINT ( 'NONE',  ( -1.848264997554276867, -10.00000000000000178, -4.668605916315860860 ) ) ;
#4566=DIRECTION ( 'NONE',  ( -0.000000000000000000, -0.5735764363510414965, -0.8191520442889950182 ) ) ;
#4568=ORIENTED_EDGE ( 'NONE', *, *, #6775, .T. ) ;
#4569=CARTESIAN_POINT ( 'NONE',  ( 2.121784821874994176, -23.95317875336422020, -3.519969256871676055 ) ) ;
#4570=LINE ( 'NONE', #10027, #13898 ) ;
#4572=EDGE_LOOP ( 'NONE', ( #3845, #5311, #5006, #5396 ) ) ;
#4577=CARTESIAN_POINT ( 'NONE',  ( -3.706921591972381904E-14, -16.89720386262061425, -6.824015130980216171 ) ) ;
#4580=CARTESIAN_POINT ( 'NONE',  ( -4.243569643749997233, -24.49592566115538972, -14.97381745050260804 ) ) ;
#4581=CARTESIAN_POINT ( 'NONE',  ( -1.071796769724486564, -28.30149810006826527, -9.163460849522957474 ) ) ;
#4582=CARTESIAN_POINT ( 'NONE',  ( -4.243569643750000786, -25.93287794636623644, -12.75450788076862452 ) ) ;
#4583=CARTESIAN_POINT ( 'NONE',  ( 0.000000000000000000, 5.977523610840987267, 32.81826849749789687 ) ) ;
#4584=LINE ( 'NONE', #8941, #14518 ) ;
#4585=DIRECTION ( 'NONE',  ( -0.000000000000000000, 1.000000000000000000, -0.000000000000000000 ) ) ;
#4586=CARTESIAN_POINT ( 'NONE',  ( 4.243569643750000786, -25.28760445547132107, -11.83296183094350340 ) ) ;
#4588=CARTESIAN_POINT ( 'NONE',  ( 4.000000000000003553, -18.13149761282945960, -5.639300014669354155 ) ) ;
#4590=VERTEX_POINT ( 'NONE', #2047 ) ;
#4592=CARTESIAN_POINT ( 'NONE',  ( 3.999999999999996447, -25.82965801714518506, -8.580776637516944305 ) ) ;
#4593=CARTESIAN_POINT ( 'NONE',  ( -3.999999999999997335, -23.72386786725210328, -13.62603244648705925 ) ) ;
#4597=CARTESIAN_POINT ( 'NONE',  ( 2.121784821874994176, -26.56653639148865409, -7.252230758663410271 ) ) ;
#4600=DIRECTION ( 'NONE',  ( 1.000000000000000000, 0.000000000000000000, 0.000000000000000000 ) ) ;
#4602=CARTESIAN_POINT ( 'NONE',  ( -4.243569643750000786, -25.44892282819504459, -12.06334834339978634 ) ) ;
#4603=FACE_OUTER_BOUND ( 'NONE', #671, .T. ) ;
#4604=LINE ( 'NONE', #4798, #15994 ) ;
#4605=CARTESIAN_POINT ( 'NONE',  ( -1.999999999999996225, -22.21875553454993124, -13.48966822215472305 ) ) ;
#4606=CARTESIAN_POINT ( 'NONE',  ( 4.243569643750003451, -19.93599299216462484, -8.461558698405095669 ) ) ;
#4607=VERTEX_POINT ( 'NONE', #13341 ) ;
#4608=CARTESIAN_POINT ( 'NONE',  ( -1.071796769724486564, -28.04338870371029557, -8.794842429592909738 ) ) ;
#4610=CARTESIAN_POINT ( 'NONE',  ( 3.999999999999996447, -22.92592730741309737, -4.433819412297139273 ) ) ;
#4612=ORIENTED_EDGE ( 'NONE', *, *, #10558, .T. ) ;
#4614=AXIS2_PLACEMENT_3D ( 'NONE', #4287, #5855, #8625 ) ;
#4616=DIRECTION ( 'NONE',  ( -0.000000000000000000, -0.5735764363510414965, -0.8191520442889950182 ) ) ;
#4620=AXIS2_PLACEMENT_3D ( 'NONE', #14260, #14447, #15744 ) ;
#4622=ORIENTED_EDGE ( 'NONE', *, *, #5925, .F. ) ;
#4625=CARTESIAN_POINT ( 'NONE',  ( 2.000000000000004441, -18.64824221826470207, -8.390446746455726412 ) ) ;
#4629=CARTESIAN_POINT ( 'NONE',  ( -6.934387221018268654, -10.37764060375305064, 2.827117695748785131 ) ) ;
#4630=CARTESIAN_POINT ( 'NONE',  ( -2.121784821875005722, -25.02863457152241722, -5.055879339913546211 ) ) ;
#4636=CARTESIAN_POINT ( 'NONE',  ( -4.000000000000000888, -23.20659744698271965, -8.860975819754113303 ) ) ;
#4637=CARTESIAN_POINT ( 'NONE',  ( 3.999999999999993339, 7.428752623566170548E-15, 30.00000000000000000 ) ) ;
#4638=CARTESIAN_POINT ( 'NONE',  ( -4.000000000000004441, -28.43226109638308330, -12.29767903747149660 ) ) ;
#4639=EDGE_LOOP ( 'NONE', ( #2393, #9544, #10796 ) ) ;
#4642=CARTESIAN_POINT ( 'NONE',  ( 4.243569643750000786, -20.89974471738585748, -5.566448692132691001 ) ) ;
#4645=CARTESIAN_POINT ( 'NONE',  ( -4.243569643750000786, -26.73946980998488954, -13.90644044305002502 ) ) ;
#4647=CARTESIAN_POINT ( 'NONE',  ( 4.713407268011036227E-15, -22.84304572250594134, -16.39440596325204780 ) ) ;
#4648=CARTESIAN_POINT ( 'NONE',  ( 2.121784821875004390, -19.42723073410004986, -9.870715949465248329 ) ) ;
#4649=CARTESIAN_POINT ( 'NONE',  ( -2.343145750507623415, -3.999999999999993339, 11.59510085796834389 ) ) ;
#4658=CARTESIAN_POINT ( 'NONE',  ( -2.000000000000005773, -22.45220093470416955, -1.744109083832446894 ) ) ;
#4660=CARTESIAN_POINT ( 'NONE',  ( 4.299564228933482956E-15, -17.21984060877302269, -7.284788156899542066 ) ) ;
#4663=CARTESIAN_POINT ( 'NONE',  ( 4.243569643749996345, -27.31605744066918007, -10.45840280688254431 ) ) ;
#4665=LINE ( 'NONE', #15899, #14331 ) ;
#4666=CARTESIAN_POINT ( 'NONE',  ( -6.938893903907228378E-15, 6.938893903907228378E-15, 5.000000000000000888 ) ) ;
#4667=ORIENTED_EDGE ( 'NONE', *, *, #15316, .F. ) ;
#4669=CARTESIAN_POINT ( 'NONE',  ( -5.330712181944245322E-15, -30.17261140584885126, -10.26649454676382867 ) ) ;
#4671=EDGE_CURVE ( 'NONE', #8069, #10853, #15235, .T. ) ;
#4673=CARTESIAN_POINT ( 'NONE',  ( -4.000000000000000888, -25.07789057128293919, -11.53345936525372650 ) ) ;
#4675=CARTESIAN_POINT ( 'NONE',  ( -4.243569643750004339, -25.85343752797401606, -8.369565093945613654 ) ) ;
#4677=CARTESIAN_POINT ( 'NONE',  ( 0.000000000000000000, 5.977523610840987267, 32.81826849749789687 ) ) ;
#4678=DIRECTION ( 'NONE',  ( -0.000000000000000000, -0.5735764363510414965, -0.8191520442889950182 ) ) ;
#4679=CARTESIAN_POINT ( 'NONE',  ( 2.121784821875004390, -20.16929524862920431, -10.93049390676413601 ) ) ;
#4680=CARTESIAN_POINT ( 'NONE',  ( 4.000000000000003553, -19.93826338733523684, -8.219628954179688307 ) ) ;
#4689=CARTESIAN_POINT ( 'NONE',  ( -1.999999999999996225, -23.05761107341827199, -14.68767808793413998 ) ) ;
#4690=PLANE ( 'NONE',  #7789 ) ;
#4693=CARTESIAN_POINT ( 'NONE',  ( 2.121784821874994176, -26.30842699513068439, -6.883612338733362535 ) ) ;
#4695=VERTEX_POINT ( 'NONE', #5265 ) ;
#4699=CARTESIAN_POINT ( 'NONE',  ( 4.730628863548789710E-15, -21.24145304325719152, -14.59743897989583594 ) ) ;
#4700=CARTESIAN_POINT ( 'NONE',  ( 3.999999999999996447, -28.60433402728840591, -12.54342465075819035 ) ) ;
#4702=CARTESIAN_POINT ( 'NONE',  ( 3.999999999999996447, -25.57154862078721891, -8.212158217586894793 ) ) ;
#4703=( BOUNDED_CURVE ( )  B_SPLINE_CURVE ( 2, ( #4139, #5439, #15468, #8309, #6733, #16771, #11086, #6913, #17042 ),
 .UNSPECIFIED., .F., .T. ) 
 B_SPLINE_CURVE_WITH_KNOTS ( ( 3, 2, 2, 2, 3 ),
 ( 0.4913793103448276245, 0.4942528735632183978, 0.5000000000000000000, 0.5057471264367816577, 0.5086206896551724865 ),
 .UNSPECIFIED. ) 
 CURVE ( )  GEOMETRIC_REPRESENTATION_ITEM ( )  RATIONAL_B_SPLINE_CURVE ( ( 0.9330127018922194093, 0.9330127018922200755, 1.000000000000000000, 0.8660254037844387076, 1.000000000000000000, 0.8660254037844387076, 1.000000000000000000, 0.9330127018922180770, 0.9330127018922194093 ) ) 
 REPRESENTATION_ITEM ( '' )  );
#4704=CARTESIAN_POINT ( 'NONE',  ( -4.243569643750005227, -23.04649784258110756, -4.360839777206344081 ) ) ;
#4706=FACE_OUTER_BOUND ( 'NONE', #4997, .T. ) ;
#4708=CARTESIAN_POINT ( 'NONE',  ( -3.706921591972381904E-14, -18.96207903348436119, -9.772962490420598058 ) ) ;
#4712=CARTESIAN_POINT ( 'NONE',  ( 4.000000000000003553, -22.26124795455695704, -11.53719473355011793 ) ) ;
#4713=DIRECTION ( 'NONE',  ( 0.5735764363510414965, -0.6710100716628397688, 0.4698463103929523821 ) ) ;
#4717=VECTOR ( 'NONE', #13801, 1000.000000000000000 ) ;
#4721=CARTESIAN_POINT ( 'NONE',  ( -4.000000000000004441, -24.04440135829761616, -6.031165898660685087 ) ) ;
#4725=EDGE_CURVE ( 'NONE', #2518, #5641, #553, .T. ) ;
#4728=CARTESIAN_POINT ( 'NONE',  ( 4.730628863548789710E-15, -18.11187661241681823, -10.12794063824400581 ) ) ;
#4735=CARTESIAN_POINT ( 'NONE',  ( 1.522508701836648326, -10.00000000000000178, 22.87631747053914211 ) ) ;
#4736=CARTESIAN_POINT ( 'NONE',  ( 1.533898589781675205E-14, -26.99942441755958811, -7.303906915216807683 ) ) ;
#4737=CARTESIAN_POINT ( 'NONE',  ( 4.433153569487552126, -10.00000000000000000, 28.39434458091830393 ) ) ;
#4738=CARTESIAN_POINT ( 'NONE',  ( 4.299564228933482956E-15, -23.34993877156982833, -16.03947562923141135 ) ) ;
#4742=CARTESIAN_POINT ( 'NONE',  ( -4.243569643749997233, -18.78525526673533719, -6.818134909550300549 ) ) ;
#4747=CARTESIAN_POINT ( 'NONE',  ( -4.000000000000004441, -27.91604230366714390, -11.56044219761140290 ) ) ;
#4748=CARTESIAN_POINT ( 'NONE',  ( -4.243569643749997233, -19.59184713035399383, -7.970067471831701056 ) ) ;
#4751=CARTESIAN_POINT ( 'NONE',  ( -4.778136680858375840, -10.00000000000000178, -10.60429372729901054 ) ) ;
#4754=CARTESIAN_POINT ( 'NONE',  ( 2.599319604203554679, -24.48737926485759431, -15.99075565718284153 ) ) ;
#4757=CARTESIAN_POINT ( 'NONE',  ( 2.121784821874994176, -22.66263177157437525, -1.676877157221437376 ) ) ;
#4761=CARTESIAN_POINT ( 'NONE',  ( -5.330712181944245322E-15, -29.36601954223019462, -9.114561984482429935 ) ) ;
#4764=CARTESIAN_POINT ( 'NONE',  ( 3.412954772041557838, -15.19080604886703512, -9.070274817126225742 ) ) ;
#4767=CARTESIAN_POINT ( 'NONE',  ( -2.121784821875005722, -28.41632039872075666, -9.893996101495421414 ) ) ;
#4768=CARTESIAN_POINT ( 'NONE',  ( -8.500000000000005329, 10.00000000000000000, -20.49999999999999645 ) ) ;
#4769=CARTESIAN_POINT ( 'NONE',  ( 2.121784821875004390, -21.71795162677701896, -13.14220442634442243 ) ) ;
#4771=B_SPLINE_CURVE_WITH_KNOTS ( 'NONE', 3,
 ( #5752, #17364, #7129, #14190, #16995, #7, #10087, #4269, #13066, #9912, #97, #11389, #381, #17080 ),
 .UNSPECIFIED., .F., .F.,
 ( 4, 2, 2, 2, 2, 2, 4 ),
 ( 0.000000000000000000, 0.004742253375847067971, 0.007113380063770602391, 0.009484506751694135943, 0.01422676012754120478, 0.01659788681546473660, 0.01896901350338827189 ),
 .UNSPECIFIED. ) ;
#4772=DIRECTION ( 'NONE',  ( 0.000000000000000000, 0.5150380737757255245, 0.8571673013836856869 ) ) ;
#4774=CARTESIAN_POINT ( 'NONE',  ( -4.243569643750000786, -22.83556519007061425, -8.331086841608051685 ) ) ;
#4783=CARTESIAN_POINT ( 'NONE',  ( -5.279047395330986450E-15, -29.05497384477128975, -9.160687100776456759 ) ) ;
#4785=EDGE_CURVE ( 'NONE', #4548, #3027, #701, .T. ) ;
#4787=ORIENTED_EDGE ( 'NONE', *, *, #11122, .T. ) ;
#4788=CARTESIAN_POINT ( 'NONE',  ( 2.121784821874994176, -26.05031759877271469, -6.514993918803313910 ) ) ;
#4791=ORIENTED_EDGE ( 'NONE', *, *, #950, .T. ) ;
#4794=VECTOR ( 'NONE', #13323, 1000.000000000000000 ) ;
#4796=CARTESIAN_POINT ( 'NONE',  ( -2.121784821875005722, -28.41632039872075666, -9.893996101495421414 ) ) ;
#4798=CARTESIAN_POINT ( 'NONE',  ( -14.99999999999999645, 10.00000000000000000, 30.00000000000000000 ) ) ;
#4799=CARTESIAN_POINT ( 'NONE',  ( 1.071796769724485454, -20.32868006578746645, -11.72467103071603134 ) ) ;
#4800=CARTESIAN_POINT ( 'NONE',  ( 2.121784821875004390, -24.04093619399873560, -16.45977020571485028 ) ) ;
#4803=CARTESIAN_POINT ( 'NONE',  ( -3.999999999999997335, -21.65899269638835634, -10.67708508704667558 ) ) ;
#4805=CARTESIAN_POINT ( 'NONE',  ( 3.999999999999996447, -25.31343922442924921, -7.843539797656847057 ) ) ;
#4809=VERTEX_POINT ( 'NONE', #15829 ) ;
#4812=CARTESIAN_POINT ( 'NONE',  ( 4.299564228933482956E-15, -16.44551241969911359, -6.178932897109397970 ) ) ;
#4813=CARTESIAN_POINT ( 'NONE',  ( -1.661723472263481630E-14, -20.31715336506863778, -11.70820919606011579 ) ) ;
#4819=CARTESIAN_POINT ( 'NONE',  ( -2.000000000000005773, -25.48498634120535655, -6.075375517003743120 ) ) ;
#4820=EDGE_LOOP ( 'NONE', ( #15015, #16241, #7135, #13282, #7186 ) ) ;
#4824=( BOUNDED_CURVE ( )  B_SPLINE_CURVE ( 2, ( #1241, #2895, #9838, #14110, #17009, #8531, #4361, #5401, #12621 ),
 .UNSPECIFIED., .F., .T. ) 
 B_SPLINE_CURVE_WITH_KNOTS ( ( 3, 2, 2, 2, 3 ),
 ( 0.008620689655172418878, 0.01149425287356321823, 0.01724137931034482735, 0.02298850574712643646, 0.02586206896551724449 ),
 .UNSPECIFIED. ) 
 CURVE ( )  GEOMETRIC_REPRESENTATION_ITEM ( )  RATIONAL_B_SPLINE_CURVE ( ( 0.9330127018922192983, 0.9330127018922194093, 1.000000000000000000, 0.8660254037844387076, 1.000000000000000000, 0.8660254037844387076, 1.000000000000000000, 0.9330127018922191873, 0.9330127018922194093 ) ) 
 REPRESENTATION_ITEM ( '' )  );
#4825=CARTESIAN_POINT ( 'NONE',  ( 9.000000000000005329, -13.00000000000000178, 15.14468620625654616 ) ) ;
#4826=CARTESIAN_POINT ( 'NONE',  ( 4.243569643750000786, -21.67407290645975948, -6.672303951922835097 ) ) ;
#4828=CARTESIAN_POINT ( 'NONE',  ( 4.730628863548789710E-15, -20.20901545782531628, -13.12296530017564500 ) ) ;
#4830=CARTESIAN_POINT ( 'NONE',  ( -1.071796769724477238, -23.07478282311446449, -1.698937844932721708 ) ) ;
#4838=CARTESIAN_POINT ( 'NONE',  ( 2.121784821875004390, -18.10442007776545736, -7.981546547323755014 ) ) ;
#4841=CARTESIAN_POINT ( 'NONE',  ( 4.243569643750003451, -24.32385273025008843, -14.72807183721590718 ) ) ;
#4842=CARTESIAN_POINT ( 'NONE',  ( 2.000000000000004441, -23.81043014542407121, -15.76281514505668113 ) ) ;
#4843=CARTESIAN_POINT ( 'NONE',  ( 4.243569643750000786, -20.93200839193060148, -5.612525994623947412 ) ) ;
#4846=CARTESIAN_POINT ( 'NONE',  ( -3.999999999999997335, -23.65934051745766808, -13.53387784049778197 ) ) ;
#4847=CYLINDRICAL_SURFACE ( 'NONE', #12147, 4.000000000000000000 ) ;
#4856=CARTESIAN_POINT ( 'NONE',  ( 2.121784821875004390, -22.75038921220889065, -14.61667810606461337 ) ) ;
#4860=CARTESIAN_POINT ( 'NONE',  ( 0.000000000000000000, 9.254131787996968228, 30.52396275209373044 ) ) ;
#4862=CARTESIAN_POINT ( 'NONE',  ( -0.2621597573796389802, -10.00000000000313527, -3.075850967169316164 ) ) ;
#4863=CARTESIAN_POINT ( 'NONE',  ( -4.243569643749997233, -23.46348807572352158, -13.49934377078241710 ) ) ;
#4864=CARTESIAN_POINT ( 'NONE',  ( -4.243569643749998122, -21.62445862667299323, -10.87293752878082742 ) ) ;
#4867=CARTESIAN_POINT ( 'NONE',  ( 4.005420803925811235, -27.01550616763517709, -14.30066121701663029 ) ) ;
#4868=CARTESIAN_POINT ( 'NONE',  ( -2.121784821875005722, -26.83540034602819802, -7.636208279423879475 ) ) ;
#4870=DIRECTION ( 'NONE',  ( 0.000000000000000000, 0.8191520442889952403, -0.5735764363510413855 ) ) ;
#4875=CARTESIAN_POINT ( 'NONE',  ( 4.000000000000000888, -24.43261708038802382, -10.61191331542860183 ) ) ;
#4876=DIRECTION ( 'NONE',  ( -0.000000000000000000, -0.5735764363510414965, -0.8191520442889950182 ) ) ;
#4879=CARTESIAN_POINT ( 'NONE',  ( 2.121784821875004390, -19.42723073410004986, -9.870715949465248329 ) ) ;
#4885=CARTESIAN_POINT ( 'NONE',  ( -4.243569643750000786, -26.22325101726895369, -13.16920360318992955 ) ) ;
#4888=CARTESIAN_POINT ( 'NONE',  ( 9.973478319601003506, -9.920655051887743880, 4.109042992078629553 ) ) ;
#4890=CARTESIAN_POINT ( 'NONE',  ( 4.730628863548789710E-15, -15.82115571973984736, -6.856452161364834375 ) ) ;
#4893=CARTESIAN_POINT ( 'NONE',  ( 4.713407268011036227E-15, -19.81026031600475790, -12.06313953008074868 ) ) ;
#4894=ORIENTED_EDGE ( 'NONE', *, *, #14181, .T. ) ;
#4904=CARTESIAN_POINT ( 'NONE',  ( -1.999999999999996225, -19.12144277825430549, -9.066247182994150222 ) ) ;
#4909=EDGE_CURVE ( 'NONE', #14839, #18119, #18355, .T. ) ;
#4910=CARTESIAN_POINT ( 'NONE',  ( -5.330712181944246111E-15, -23.94572221871285578, -1.373575165951426369 ) ) ;
#4913=CARTESIAN_POINT ( 'NONE',  ( 4.243569643750003451, -21.74275876667039853, -11.04188763791542804 ) ) ;
#4914=CARTESIAN_POINT ( 'NONE',  ( 1.049162765915156337, -30.17532418831297747, -12.05880678485356583 ) ) ;
#4917=CARTESIAN_POINT ( 'NONE',  ( 6.097036691291187083, -11.55344374157293608, 15.47841750116241499 ) ) ;
#4920=CARTESIAN_POINT ( 'NONE',  ( 4.243569643749996345, -28.63886809700377611, -12.34757220902403851 ) ) ;
#4924=CARTESIAN_POINT ( 'NONE',  ( 4.730628863548789710E-15, -17.85376721605885209, -9.759322218313958075 ) ) ;
#4927=CARTESIAN_POINT ( 'NONE',  ( 2.121784821875004390, -23.81509047218551700, -16.13722908827605806 ) ) ;
#4928=CARTESIAN_POINT ( 'NONE',  ( -1.999999999999996225, -23.76741191269774234, -15.70137874173500947 ) ) ;
#4929=( BOUNDED_CURVE ( )  B_SPLINE_CURVE ( 2, ( #2850, #248, #14435, #64, #8856, #14342, #15555, #1373, #1640 ),
 .UNSPECIFIED., .F., .T. ) 
 B_SPLINE_CURVE_WITH_KNOTS ( ( 3, 2, 2, 2, 3 ),
 ( 0.5086206896551724865, 0.5114942528735632044, 0.5172413793103448620, 0.5229885057471264087, 0.5258620689655172376 ),
 .UNSPECIFIED. ) 
 CURVE ( )  GEOMETRIC_REPRESENTATION_ITEM ( )  RATIONAL_B_SPLINE_CURVE ( ( 0.9330127018922194093, 0.9330127018922206306, 1.000000000000000000, 0.8660254037844387076, 1.000000000000000000, 0.8660254037844387076, 1.000000000000000000, 0.9330127018922194093, 0.9330127018922194093 ) ) 
 REPRESENTATION_ITEM ( '' )  );
#4930=CARTESIAN_POINT ( 'NONE',  ( -5.330712181944245322E-15, -25.78475166776338412, -3.999981407953017598 ) ) ;
#4933=CARTESIAN_POINT ( 'NONE',  ( 4.000000000000003553, -25.03592396470017434, -15.49984274679136576 ) ) ;
#4936=ORIENTED_EDGE ( 'NONE', *, *, #15856, .T. ) ;
#4939=CARTESIAN_POINT ( 'NONE',  ( 7.082261791595104050, -12.11712549938399341, 11.44383700422758210 ) ) ;
#4944=CARTESIAN_POINT ( 'NONE',  ( 4.243569643750000786, -26.06193264454523018, -12.93881709073364661 ) ) ;
#4947=CARTESIAN_POINT ( 'NONE',  ( -1.998401444325281457E-14, -15.45745613286698550, -10.86990606519495195 ) ) ;
#4948=CARTESIAN_POINT ( 'NONE',  ( 4.243569643749996345, -27.34832111521392761, -10.50448010937380161 ) ) ;
#4952=CARTESIAN_POINT ( 'NONE',  ( 4.150834101209824212, -27.15734369766470380, -14.50322620280942587 ) ) ;
#4953=EDGE_CURVE ( 'NONE', #244, #2141, #4929, .T. ) ;
#4957=CARTESIAN_POINT ( 'NONE',  ( 4.243569643749996345, -26.02551045887933867, -8.615310707232305631 ) ) ;
#4959=CARTESIAN_POINT ( 'NONE',  ( -2.000000000000005773, -22.45220093470416955, -1.744109083832446894 ) ) ;
#4961=CYLINDRICAL_SURFACE ( 'NONE', #10904, 4.000000000000000000 ) ;
#4966=DIRECTION ( 'NONE',  ( -0.000000000000000000, 1.000000000000000000, -0.000000000000000000 ) ) ;
#4968=CARTESIAN_POINT ( 'NONE',  ( 2.121784821874994176, -25.27598940969881269, -5.409138659013170702 ) ) ;
#4973=EDGE_CURVE ( 'NONE', #14065, #17065, #7525, .T. ) ;
#4974=CARTESIAN_POINT ( 'NONE',  ( -3.993033241984866866, -27.55172186255954259, -14.02642606169049522 ) ) ;
#4977=CARTESIAN_POINT ( 'NONE',  ( 6.804197231186874362, -11.93903049149238527, 12.87607830000603393 ) ) ;
#4980=CARTESIAN_POINT ( 'NONE',  ( -1.071796769724496334, -24.10722040854632908, -3.173411524652919979 ) ) ;
#4981=CARTESIAN_POINT ( 'NONE',  ( -4.243569643750005227, -21.75595086079126261, -2.517747677556105845 ) ) ;
#4982=ORIENTED_EDGE ( 'NONE', *, *, #8491, .F. ) ;
#4983=DIRECTION ( 'NONE',  ( -0.000000000000000000, -0.5735764363510414965, -0.8191520442889950182 ) ) ;
#4984=CARTESIAN_POINT ( 'NONE',  ( 4.713407268011036227E-15, -19.29404152328881850, -11.32590269022065499 ) ) ;
#4986=ORIENTED_EDGE ( 'NONE', *, *, #13858, .F. ) ;
#4996=CARTESIAN_POINT ( 'NONE',  ( 4.000000000000003553, -19.87373603754079809, -8.127474348190411035 ) ) ;
#4997=EDGE_LOOP ( 'NONE', ( #8274, #5098, #11967, #6143 ) ) ;
#4998=CYLINDRICAL_SURFACE ( 'NONE', #17481, 4.000000000000000000 ) ;
#5000=CARTESIAN_POINT ( 'NONE',  ( 1.999999999999994449, -28.28117146841668728, -10.06874173291258856 ) ) ;
#5001=CARTESIAN_POINT ( 'NONE',  ( -2.121784821874996396, -17.02896425960724969, -6.445636464281891520 ) ) ;
#5002=CARTESIAN_POINT ( 'NONE',  ( -4.243569643750000786, -24.67459463912114259, -10.95749308360964136 ) ) ;
#5003=PRODUCT_DEFINITION_SHAPE ( 'NONE', 'NONE',  #3009 ) ;
#5006=ORIENTED_EDGE ( 'NONE', *, *, #3197, .F. ) ;
#5007=CARTESIAN_POINT ( 'NONE',  ( -2.531783071939982754, -10.67720498481812541, 21.39218517664744823 ) ) ;
#5009=CARTESIAN_POINT ( 'NONE',  ( -4.243569643750000786, -26.99757920634285924, -14.27505886298007276 ) ) ;
#5010=ORIENTED_EDGE ( 'NONE', *, *, #7443, .F. ) ;
#5012=CARTESIAN_POINT ( 'NONE',  ( 4.004198159875437923, -26.67562288373377299, -14.52967640179035413 ) ) ;
#5013=CARTESIAN_POINT ( 'NONE',  ( -4.243569643750005227, -22.49801537532042062, -3.577525634854993086 ) ) ;
#5015=ADVANCED_FACE ( 'NONE', ( #13214 ), #4690, .T. ) ;
#5017=EDGE_CURVE ( 'NONE', #13681, #7716, #1832, .T. ) ;
#5018=CARTESIAN_POINT ( 'NONE',  ( -4.000000000000004441, -27.65793290730917064, -11.19182377768135339 ) ) ;
#5019=ORIENTED_EDGE ( 'NONE', *, *, #778, .F. ) ;
#5022=CARTESIAN_POINT ( 'NONE',  ( -5.330712181944245322E-15, -24.75231408233150887, -2.525507728232826210 ) ) ;
#5024=EDGE_CURVE ( 'NONE', #11442, #218, #2460, .T. ) ;
#5028=ORIENTED_EDGE ( 'NONE', *, *, #8853, .F. ) ;
#5036=CARTESIAN_POINT ( 'NONE',  ( -2.121784821874996396, -22.96548037584052793, -14.92386012267298945 ) ) ;
#5038=( BOUNDED_CURVE ( )  B_SPLINE_CURVE ( 3, ( #11201, #937, #1306, #2428 ),
 .UNSPECIFIED., .F., .T. ) 
 B_SPLINE_CURVE_WITH_KNOTS ( ( 4, 4 ),
 ( 0.000000000000000000, 1.029696800837750059 ),
 .UNSPECIFIED. ) 
 CURVE ( )  GEOMETRIC_REPRESENTATION_ITEM ( )  RATIONAL_B_SPLINE_CURVE ( ( 1.000000000000000000, 0.9135782535825738293, 0.9135782535825738293, 1.000000000000000000 ) ) 
 REPRESENTATION_ITEM ( '' )  );
#5040=CARTESIAN_POINT ( 'NONE',  ( -1.661723472263481630E-14, -21.80128239342201724, -13.82776510965112671 ) ) ;
#5041=CARTESIAN_POINT ( 'NONE',  ( -4.243569643750005227, -26.91813878795063886, -9.890116076157061897 ) ) ;
#5044=CARTESIAN_POINT ( 'NONE',  ( -1.071796769724496334, -23.39741956926685518, -2.159710870852054931 ) ) ;
#5046=CARTESIAN_POINT ( 'NONE',  ( -4.243569643750000786, -23.35178398278655010, -9.068323681468148934 ) ) ;
#5048=FACE_OUTER_BOUND ( 'NONE', #15426, .T. ) ;
#5049=CARTESIAN_POINT ( 'NONE',  ( 3.064181913176683203, -21.66367673124435100, -2.174801284911689780 ) ) ;
#5051=VERTEX_POINT ( 'NONE', #13406 ) ;
#5053=CARTESIAN_POINT ( 'NONE',  ( 1.475796370471763337E-14, -22.05939178977998694, -14.19638352958117267 ) ) ;
#5059=CARTESIAN_POINT ( 'NONE',  ( -5.330712181944246111E-15, -26.55907985683728967, -5.105836667743160362 ) ) ;
#5061=ORIENTED_EDGE ( 'NONE', *, *, #1321, .F. ) ;
#5063=FACE_OUTER_BOUND ( 'NONE', #7850, .T. ) ;
#5065=CARTESIAN_POINT ( 'NONE',  ( -1.355220984792064876, -23.95640476330365587, -16.63505457156503908 ) ) ;
#5067=CARTESIAN_POINT ( 'NONE',  ( 5.992170350750239294, -10.31447287898148168, 0.09153525861095850036 ) ) ;
#5068=CARTESIAN_POINT ( 'NONE',  ( -1.999999999999996225, -18.08900519282243025, -7.591773503273958390 ) ) ;
#5069=CARTESIAN_POINT ( 'NONE',  ( 4.243569643750003451, -18.64544601037477278, -6.618466598754856101 ) ) ;
#5070=ORIENTED_EDGE ( 'NONE', *, *, #17401, .T. ) ;
#5072=CARTESIAN_POINT ( 'NONE',  ( -2.000000000000005773, -26.58195127643166700, -7.642003802713210447 ) ) ;
#5074=ORIENTED_EDGE ( 'NONE', *, *, #14025, .F. ) ;
#5075=ORIENTED_EDGE ( 'NONE', *, *, #12780, .F. ) ;
#5076=CARTESIAN_POINT ( 'NONE',  ( -3.999999999999997335, -19.52959017573017064, -7.635983121617017311 ) ) ;
#5080=VERTEX_POINT ( 'NONE', #11826 ) ;
#5083=CARTESIAN_POINT ( 'NONE',  ( 2.000000000000004441, -17.61580463283282683, -6.915973066735536356 ) ) ;
#5087=CARTESIAN_POINT ( 'NONE',  ( 4.000000000000003553, -21.93861120840455214, -11.07642170763079292 ) ) ;
#5089=CARTESIAN_POINT ( 'NONE',  ( -4.243569643750000786, -20.77069001920686375, -5.382139482167671574 ) ) ;
#5091=CARTESIAN_POINT ( 'NONE',  ( -2.121784821874996396, -21.70719706859543408, -13.12684532551400629 ) ) ;
#5093=CARTESIAN_POINT ( 'NONE',  ( -1.373763480980777274, -30.12088136896208113, -12.14767278240311654 ) ) ;
#5095=CARTESIAN_POINT ( 'NONE',  ( -7.971931588564060256, -10.00000000000000178, 17.73270869615951639 ) ) ;
#5097=CARTESIAN_POINT ( 'NONE',  ( -4.243569643750005227, -28.46679516609844995, -12.10182659573734476 ) ) ;
#5098=ORIENTED_EDGE ( 'NONE', *, *, #12016, .F. ) ;
#5100=CARTESIAN_POINT ( 'NONE',  ( 3.511779744724054186, -25.38768362883276097, -15.39278514861212699 ) ) ;
#5101=CARTESIAN_POINT ( 'NONE',  ( 2.121784821874994176, -22.66263177157437525, -1.676877157221437376 ) ) ;
#5106=CARTESIAN_POINT ( 'NONE',  ( -4.000000000000004441, -26.88360471823526865, -10.08596851789121018 ) ) ;
#5109=CARTESIAN_POINT ( 'NONE',  ( 4.243569643750000786, -21.70633658100450702, -6.718381254414091508 ) ) ;
#5116=DIRECTION ( 'NONE',  ( -0.000000000000000000, -0.000000000000000000, -1.000000000000000000 ) ) ;
#5120=DIRECTION ( 'NONE',  ( -1.000000000000000000, 0.000000000000000000, 0.000000000000000000 ) ) ;
#5121=CARTESIAN_POINT ( 'NONE',  ( -1.661723472263481630E-14, -20.76884480799014554, -12.35329142993093576 ) ) ;
#5124=CARTESIAN_POINT ( 'NONE',  ( -4.243569643750005227, -25.85343752797401606, -8.369565093945613654 ) ) ;
#5127=CARTESIAN_POINT ( 'NONE',  ( -4.000000000000003553, 6.938893903907228378E-15, 24.28148006742132026 ) ) ;
#5128=CARTESIAN_POINT ( 'NONE',  ( -1.071796769724496334, -20.75731810727131332, -12.33682959527501488 ) ) ;
#5131=CARTESIAN_POINT ( 'NONE',  ( 4.730628863548789710E-15, -20.98334364689921827, -14.22882055996578643 ) ) ;
#5134=DIRECTION ( 'NONE',  ( -0.000000000000000000, 1.000000000000000000, -0.000000000000000000 ) ) ;
#5135=EDGE_CURVE ( 'NONE', #11008, #9284, #7746, .T. ) ;
#5136=LINE ( 'NONE', #13760, #1131 ) ;
#5137=( BOUNDED_CURVE ( )  B_SPLINE_CURVE ( 2, ( #1594, #11677, #4550, #12886, #4636, #15774, #1502, #7513, #3074 ),
 .UNSPECIFIED., .F., .F. ) 
 B_SPLINE_CURVE_WITH_KNOTS ( ( 3, 2, 2, 2, 3 ),
 ( 0.5258620689655172376, 0.5287356321839080664, 0.5344827586206896131, 0.5402298850574712707, 0.5431034482758620996 ),
 .UNSPECIFIED. ) 
 CURVE ( )  GEOMETRIC_REPRESENTATION_ITEM ( )  RATIONAL_B_SPLINE_CURVE ( ( 0.9330127018922194093, 0.9330127018922194093, 1.000000000000000000, 0.8660254037844387076, 1.000000000000000000, 0.8660254037844387076, 1.000000000000000000, 0.9330127018922194093, 0.9330127018922194093 ) ) 
 REPRESENTATION_ITEM ( '' )  );
#5138=CARTESIAN_POINT ( 'NONE',  ( -4.243569643750005227, -23.78856235711026912, -5.420617734505229990 ) ) ;
#5144=CARTESIAN_POINT ( 'NONE',  ( 1.999999999999994449, -23.37709293761528784, -3.064991754241682465 ) ) ;
#5146=CARTESIAN_POINT ( 'NONE',  ( -1.999999999999996225, -17.31467700374852470, -6.485918243483816958 ) ) ;
#5150=ORIENTED_EDGE ( 'NONE', *, *, #2081, .T. ) ;
#5151=CARTESIAN_POINT ( 'NONE',  ( 4.243569643749997233, -23.47668016984440342, -4.975203810423082906 ) ) ;
#5157=EDGE_CURVE ( 'NONE', #2835, #4535, #5726, .T. ) ;
#5159=DIRECTION ( 'NONE',  ( 0.000000000000000000, -0.000000000000000000, 1.000000000000000000 ) ) ;
#5160=CARTESIAN_POINT ( 'NONE',  ( 9.828195458270586826, -9.943122604294416078, 1.729283279605983159 ) ) ;
#5162=CARTESIAN_POINT ( 'NONE',  ( -5.330712181944245322E-15, -24.49420468597353562, -2.156889308302778030 ) ) ;
#5165=CARTESIAN_POINT ( 'NONE',  ( 4.000000000000003553, -21.74502916184101764, -10.79995789369002246 ) ) ;
#5175=CARTESIAN_POINT ( 'NONE',  ( 4.000000000000000888, -20.23833938886609118, -4.621863990558560786 ) ) ;
#5180=CARTESIAN_POINT ( 'NONE',  ( 15.00000000000000355, 10.00000000000000000, 30.00000000000000000 ) ) ;
#5182=CARTESIAN_POINT ( 'NONE',  ( -4.243569643750000786, -19.99636183013295820, -4.276284222377527477 ) ) ;
#5183=CARTESIAN_POINT ( 'NONE',  ( -4.243569643750005227, -25.62759180616079746, -8.047023976506819665 ) ) ;
#5185=DIRECTION ( 'NONE',  ( 0.000000000000000000, 0.8191520442889952403, -0.5735764363510413855 ) ) ;
#5188=PRODUCT_DEFINITION_CONTEXT ( 'detailed design', #14235, 'design' ) ;
#5190=CARTESIAN_POINT ( 'NONE',  ( -8.500000000000005329, 10.00000000000000000, 18.49999999999999645 ) ) ;
#5192=CARTESIAN_POINT ( 'NONE',  ( -2.121784821874996396, -23.25585344674324162, -15.33855584509429271 ) ) ;
#5193=ORIENTED_EDGE ( 'NONE', *, *, #9036, .F. ) ;
#5197=CARTESIAN_POINT ( 'NONE',  ( 4.243569643749996345, -22.15386951350980738, -3.086034408281590036 ) ) ;
#5201=CARTESIAN_POINT ( 'NONE',  ( 3.999999999999996447, -26.53945885642465186, -9.594477291317808465 ) ) ;
#5204=CARTESIAN_POINT ( 'NONE',  ( -4.243569643750005227, -22.53027904986517527, -3.623602937346249497 ) ) ;
#5207=CARTESIAN_POINT ( 'NONE',  ( -2.121784821874996396, -21.15871460133474713, -12.34353118316265707 ) ) ;
#5210=LINE ( 'NONE', #7987, #7634 ) ;
#5214=CARTESIAN_POINT ( 'NONE',  ( 6.808477104226121845, -11.94136413928387519, 12.86032843472113818 ) ) ;
#5215=ORIENTED_EDGE ( 'NONE', *, *, #16997, .F. ) ;
#5218=CARTESIAN_POINT ( 'NONE',  ( -4.243569643750000786, -23.60989337914451625, -9.436942101398194893 ) ) ;
#5223=CARTESIAN_POINT ( 'NONE',  ( 8.500000000000019540, 10.00000000000000000, 18.49999999999998934 ) ) ;
#5224=CARTESIAN_POINT ( 'NONE',  ( -4.243569643750005227, -26.14381059887672976, -8.784260816366916913 ) ) ;
#5226=FACE_OUTER_BOUND ( 'NONE', #5366, .T. ) ;
#5230=CARTESIAN_POINT ( 'NONE',  ( 4.243569643750000786, -21.93218230281772918, -7.040922371852881945 ) ) ;
#5232=DIRECTION ( 'NONE',  ( 0.000000000000000000, -0.000000000000000000, -1.000000000000000000 ) ) ;
#5233=CARTESIAN_POINT ( 'NONE',  ( 1.071796769724485232, -28.53655409498856699, -9.499155600141175881 ) ) ;
#5235=CARTESIAN_POINT ( 'NONE',  ( 4.299564228933482956E-15, -17.15531325897858039, -7.192633550910265683 ) ) ;
#5241=ORIENTED_EDGE ( 'NONE', *, *, #10788, .T. ) ;
#5242=CARTESIAN_POINT ( 'NONE',  ( 2.121784821875004390, -17.87857435595223876, -7.659005429884962801 ) ) ;
#5248=CARTESIAN_POINT ( 'NONE',  ( -3.706921591972381904E-14, -18.44586024076842534, -9.035725650560502586 ) ) ;
#5249=DIRECTION ( 'NONE',  ( 0.000000000000000000, 0.000000000000000000, 1.000000000000000000 ) ) ;
#5250=PLANE ( 'NONE',  #13204 ) ;
#5253=CARTESIAN_POINT ( 'NONE',  ( -4.243569643750005227, -27.66020330247980041, -10.94989403345594425 ) ) ;
#5254=ORIENTED_EDGE ( 'NONE', *, *, #11755, .T. ) ;
#5256=CARTESIAN_POINT ( 'NONE',  ( -3.999999999999997335, -19.33600812916663614, -7.359519307676247735 ) ) ;
#5261=ORIENTED_EDGE ( 'NONE', *, *, #8082, .F. ) ;
#5262=CARTESIAN_POINT ( 'NONE',  ( -1.071796769724496334, -24.36532980490429878, -3.542029944582967271 ) ) ;
#5265=CARTESIAN_POINT ( 'NONE',  ( -5.577813053751546416E-15, -29.32240898478130120, -10.62147269458723464 ) ) ;
#5268=CARTESIAN_POINT ( 'NONE',  ( -2.121784821874996396, -22.99774405038527547, -14.96993742516424497 ) ) ;
#5270=CARTESIAN_POINT ( 'NONE',  ( -4.000000000000000888, -20.10928469068709745, -4.437554780593541359 ) ) ;
#5271=VERTEX_POINT ( 'NONE', #16573 ) ;
#5272=CARTESIAN_POINT ( 'NONE',  ( -3.706921591972381904E-14, -18.44586024076842534, -9.035725650560502586 ) ) ;
#5275=ADVANCED_FACE ( 'NONE', ( #994 ), #15175, .F. ) ;
#5276=CARTESIAN_POINT ( 'NONE',  ( 4.243569643750000786, -20.12541652831194838, -4.460593432342547793 ) ) ;
#5277=CARTESIAN_POINT ( 'NONE',  ( -5.330712181944245322E-15, -26.81718925319525937, -5.474455087673208986 ) ) ;
#5279=ORIENTED_EDGE ( 'NONE', *, *, #13687, .T. ) ;
#5280=CARTESIAN_POINT ( 'NONE',  ( 2.000000000000004441, -21.29386353163882717, -12.16878555174548104 ) ) ;
#5281=FACE_OUTER_BOUND ( 'NONE', #5438, .T. ) ;
#5288=VECTOR ( 'NONE', #4184, 1000.000000000000000 ) ;
#5289=CARTESIAN_POINT ( 'NONE',  ( -2.121784821875005722, -23.22186879701663642, -2.475550400403212503 ) ) ;
#5292=CARTESIAN_POINT ( 'NONE',  ( 1.999999999999994449, -27.76495267570075143, -9.331504893052493088 ) ) ;
#5295=CARTESIAN_POINT ( 'NONE',  ( 4.730628863548789710E-15, -15.82115571973984736, -6.856452161364834375 ) ) ;
#5297=EDGE_CURVE ( 'NONE', #2086, #12341, #17608, .T. ) ;
#5300=CARTESIAN_POINT ( 'NONE',  ( -4.243569643750004339, -26.62776571704792161, -9.475420353735756862 ) ) ;
#5301=CARTESIAN_POINT ( 'NONE',  ( -4.000000000000000888, -26.04580080692037569, -12.91577843898463840 ) ) ;
#5302=CARTESIAN_POINT ( 'NONE',  ( 4.000000000000003553, -19.42204459461930099, -7.482392114319592835 ) ) ;
#5303=CARTESIAN_POINT ( 'NONE',  ( -1.999999999999996225, -20.47651710983858564, -11.00149388863366440 ) ) ;
#5305=ORIENTED_EDGE ( 'NONE', *, *, #13683, .F. ) ;
#5308=CARTESIAN_POINT ( 'NONE',  ( -4.000000000000007105, 0.000000000000000000, -4.999999999999997335 ) ) ;
#5309=CARTESIAN_POINT ( 'NONE',  ( 3.999999999999996447, -28.66886137708284110, -12.63557925674746762 ) ) ;
#5310=CARTESIAN_POINT ( 'NONE',  ( 7.037197741572231990, -13.81849642415488688, -0.01350879608600348905 ) ) ;
#5311=ORIENTED_EDGE ( 'NONE', *, *, #4354, .T. ) ;
#5314=CARTESIAN_POINT ( 'NONE',  ( 4.243569643749996345, -26.28361985523730837, -8.983929127162353367 ) ) ;
#5321=CARTESIAN_POINT ( 'NONE',  ( 2.121784821874994176, -26.82464578784662379, -7.620849178593458007 ) ) ;
#5329=CARTESIAN_POINT ( 'NONE',  ( -4.243569643749997233, -20.33391164488314828, -9.029845429130588741 ) ) ;
#5330=CARTESIAN_POINT ( 'NONE',  ( 3.999999999999996447, -26.60398620621909416, -9.686631897307085737 ) ) ;
#5333=CARTESIAN_POINT ( 'NONE',  ( 1.533898589781675205E-14, -26.74131502120161841, -6.935288495286759058 ) ) ;
#5335=CARTESIAN_POINT ( 'NONE',  ( -3.706921591972381904E-14, -16.89720386262061425, -6.824015130980216171 ) ) ;
#5337=VERTEX_POINT ( 'NONE', #12558 ) ;
#5338=CARTESIAN_POINT ( 'NONE',  ( -2.121784821874996396, -18.60988431229980833, -8.703424286353433459 ) ) ;
#5341=CARTESIAN_POINT ( 'NONE',  ( 4.243569643750003451, -24.54969845206330703, -15.05061295465469762 ) ) ;
#5345=CARTESIAN_POINT ( 'NONE',  ( -4.243569643750005227, -27.91831269883777011, -11.31851245338599377 ) ) ;
#5348=CARTESIAN_POINT ( 'NONE',  ( 9.000000000000005329, -10.00000000000000000, 30.00000000000000000 ) ) ;
#5349=CARTESIAN_POINT ( 'NONE',  ( -5.279047395330986450E-15, -24.92522350304378875, -3.262792381895696092 ) ) ;
#5353=VERTEX_POINT ( 'NONE', #9775 ) ;
#5361=ORIENTED_EDGE ( 'NONE', *, *, #16558, .T. ) ;
#5362=CARTESIAN_POINT ( 'NONE',  ( 4.243569643750000786, -25.31986813001606862, -11.87903913343475892 ) ) ;
#5363=ADVANCED_FACE ( 'NONE', ( #15619 ), #129, .T. ) ;
#5365=CARTESIAN_POINT ( 'NONE',  ( -1.999999999999996225, -17.83089579646446410, -7.223155083343911542 ) ) ;
#5366=EDGE_LOOP ( 'NONE', ( #15916, #14016, #5448, #14530 ) ) ;
#5369=EDGE_CURVE ( 'NONE', #17169, #7294, #16191, .T. ) ;
#5372=CARTESIAN_POINT ( 'NONE',  ( -5.330712181944245322E-15, -27.33340804591119522, -6.211691927533303570 ) ) ;
#5373=CARTESIAN_POINT ( 'NONE',  ( 4.898587196589413815E-16, 2.700915433685006750, 35.11257424290206330 ) ) ;
#5375=CARTESIAN_POINT ( 'NONE',  ( 2.000000000000004441, -21.03575413528086102, -11.80016713181543331 ) ) ;
#5376=CARTESIAN_POINT ( 'NONE',  ( 3.999999999999996447, -27.05567764914059481, -10.33171413117790394 ) ) ;
#5382=CARTESIAN_POINT ( 'NONE',  ( 4.243569643750000786, -20.38352592466991808, -4.829211852272596417 ) ) ;
#5385=CARTESIAN_POINT ( 'NONE',  ( -3.999999999999997335, -22.36879353566782669, -11.69078574084754152 ) ) ;
#5388=CARTESIAN_POINT ( 'NONE',  ( -2.121784821874996396, -17.31933733050996338, -6.860332186703194779 ) ) ;
#5392=CARTESIAN_POINT ( 'NONE',  ( -2.121784821874996396, -20.38438641226084158, -11.23767592337251209 ) ) ;
#5393=CARTESIAN_POINT ( 'NONE',  ( 4.000000000000000888, -24.36808973059358863, -10.51975870943932456 ) ) ;
#5394=CARTESIAN_POINT ( 'NONE',  ( -3.999999999999997335, -21.40088330003039019, -10.30846666711662962 ) ) ;
#5396=ORIENTED_EDGE ( 'NONE', *, *, #8693, .F. ) ;
#5398=CARTESIAN_POINT ( 'NONE',  ( 3.579096709490575479E-14, -25.12813129325936501, -4.631423369717193594 ) ) ;
#5401=CARTESIAN_POINT ( 'NONE',  ( -1.071796769724494114, -30.10826387457404607, -11.74378978903329518 ) ) ;
#5405=CARTESIAN_POINT ( 'NONE',  ( -2.121784821875005722, -26.83540034602819802, -7.636208279423879475 ) ) ;
#5409=CARTESIAN_POINT ( 'NONE',  ( 9.000000000000005329, -10.00000000000000000, -3.713574246709344884 ) ) ;
#5412=CARTESIAN_POINT ( 'NONE',  ( -2.121784821874996396, -21.70719706859543408, -13.12684532551400629 ) ) ;
#5414=( BOUNDED_CURVE ( )  B_SPLINE_CURVE ( 2, ( #17535, #17437, #5997, #4702, #11651, #8771, #7758, #4799, #10450 ),
 .UNSPECIFIED., .F., .F. ) 
 B_SPLINE_CURVE_WITH_KNOTS ( ( 3, 2, 2, 2, 3 ),
 ( 0.4396551724137931494, 0.4425287356321839227, 0.4482758620689655249, 0.4540229885057471271, 0.4568965517241379559 ),
 .UNSPECIFIED. ) 
 CURVE ( )  GEOMETRIC_REPRESENTATION_ITEM ( )  RATIONAL_B_SPLINE_CURVE ( ( 0.9330127018922194093, 0.9330127018922200755, 1.000000000000000000, 0.8660254037844387076, 1.000000000000000000, 0.8660254037844387076, 1.000000000000000000, 0.9330127018922187432, 0.9330127018922194093 ) ) 
 REPRESENTATION_ITEM ( '' )  );
#5415=CARTESIAN_POINT ( 'NONE',  ( -6.938893903907228378E-15, 6.938893903907228378E-15, -30.00000000000000000 ) ) ;
#5418=CARTESIAN_POINT ( 'NONE',  ( 4.730628863548789710E-15, -18.62809540513275408, -10.86517747810410306 ) ) ;
#5425=CARTESIAN_POINT ( 'NONE',  ( -1.999999999999996225, -22.47686493090789739, -13.85828664208477079 ) ) ;
#5430=CARTESIAN_POINT ( 'NONE',  ( -2.121784821875005722, -23.77035126427731981, -3.258864542754563942 ) ) ;
#5432=CARTESIAN_POINT ( 'NONE',  ( -2.694913683823399353, -10.54254386713301805, 22.30101802474215233 ) ) ;
#5437=CARTESIAN_POINT ( 'NONE',  ( 4.243569643750003451, -23.77537026298940148, -13.94475769486455619 ) ) ;
#5438=EDGE_LOOP ( 'NONE', ( #1952, #5150, #11804, #1996 ) ) ;
#5439=CARTESIAN_POINT ( 'NONE',  ( -1.071796769724496334, -20.24109931455537392, -11.59959275541492119 ) ) ;
#5440=CARTESIAN_POINT ( 'NONE',  ( -5.279047395330986450E-15, -25.44144229575972460, -4.000029221755790232 ) ) ;
#5443=CARTESIAN_POINT ( 'NONE',  ( -5.577813053751546416E-15, -23.90211166126395881, -2.880485876056233518 ) ) ;
#5448=ORIENTED_EDGE ( 'NONE', *, *, #16149, .F. ) ;
#5449=CARTESIAN_POINT ( 'NONE',  ( -2.121784821875005722, -29.19064858779466221, -10.99985136128556462 ) ) ;
#5451=CARTESIAN_POINT ( 'NONE',  ( -4.000000000000000888, -21.39983167247694240, -6.280646880243780039 ) ) ;
#5452=CIRCLE ( 'NONE', #13736, 2.000000000000001776 ) ;
#5454=ADVANCED_FACE ( 'NONE', ( #17030, #14131 ), #1444, .T. ) ;
#5456=CARTESIAN_POINT ( 'NONE',  ( -1.999999999999996225, -21.25084529891249119, -12.10734914842380761 ) ) ;
#5457=DIRECTION ( 'NONE',  ( -0.000000000000000000, -0.5735764363510414965, -0.8191520442889950182 ) ) ;
#5459=CARTESIAN_POINT ( 'NONE',  ( -4.243569643749997233, -20.88239411214383523, -9.813159571481939736 ) ) ;
#5463=CARTESIAN_POINT ( 'NONE',  ( -5.279047395330986450E-15, -28.53875505205535035, -8.423450260916363064 ) ) ;
#5464=CYLINDRICAL_SURFACE ( 'NONE', #3017, 4.000000000000000000 ) ;
#5467=ORIENTED_EDGE ( 'NONE', *, *, #16182, .F. ) ;
#5470=CARTESIAN_POINT ( 'NONE',  ( 4.000000000000003553, -24.32612312542070754, -14.48614209299049804 ) ) ;
#5474=CARTESIAN_POINT ( 'NONE',  ( -5.279047395330986450E-15, -28.73233709861888485, -8.699914074857131752 ) ) ;
#5478=CARTESIAN_POINT ( 'NONE',  ( 3.250767888004682415, -21.90484815091188509, -2.246271217071878823 ) ) ;
#5482=CARTESIAN_POINT ( 'NONE',  ( 2.121784821874994176, -26.27616332058593684, -6.837535036242106123 ) ) ;
#5483=CARTESIAN_POINT ( 'NONE',  ( 4.000000000000003553, -22.45483000112048799, -11.81365854749088840 ) ) ;
#5484=CARTESIAN_POINT ( 'NONE',  ( 1.071796769724476128, -17.68305875241334491, -7.946332225426282037 ) ) ;
#5486=ORIENTED_EDGE ( 'NONE', *, *, #12314, .F. ) ;
#5494=CARTESIAN_POINT ( 'NONE',  ( -5.330712181944245322E-15, -28.59169135315628907, -8.008706724692286727 ) ) ;
#5498=FACE_OUTER_BOUND ( 'NONE', #6297, .T. ) ;
#5499=CARTESIAN_POINT ( 'NONE',  ( 2.121784821875004390, -20.45966831953192511, -11.34518962918543927 ) ) ;
#5500=LINE ( 'NONE', #2823, #14123 ) ;
#5504=CARTESIAN_POINT ( 'NONE',  ( -4.243569643750005227, -24.30478114982620497, -6.157854574365327238 ) ) ;
#5506=CARTESIAN_POINT ( 'NONE',  ( 3.999999999999993339, 7.428752623566170548E-15, 30.00000000000000000 ) ) ;
#5509=CARTESIAN_POINT ( 'NONE',  ( -1.999999999999996225, -19.37955217461227875, -9.434865602924197958 ) ) ;
#5511=CARTESIAN_POINT ( 'NONE',  ( 1.071796769724485232, -29.05277288770450639, -10.23639244000127135 ) ) ;
#5515=CARTESIAN_POINT ( 'NONE',  ( 2.121784821875004390, -18.13668375231020846, -8.027623849815011425 ) ) ;
#5517=( BOUNDED_CURVE ( )  B_SPLINE_CURVE ( 2, ( #8588, #7201, #1046, #11370, #7111, #9561, #17060, #15240, #6685 ),
 .UNSPECIFIED., .F., .T. ) 
 B_SPLINE_CURVE_WITH_KNOTS ( ( 3, 2, 2, 2, 3 ),
 ( 0.1293103448275862155, 0.1321839080459770166, 0.1379310344827586188, 0.1436781609195402210, 0.1465517241379310498 ),
 .UNSPECIFIED. ) 
 CURVE ( )  GEOMETRIC_REPRESENTATION_ITEM ( )  RATIONAL_B_SPLINE_CURVE ( ( 0.9330127018922194093, 0.9330127018922194093, 1.000000000000000000, 0.8660254037844387076, 1.000000000000000000, 0.8660254037844387076, 1.000000000000000000, 0.9330127018922189652, 0.9330127018922192983 ) ) 
 REPRESENTATION_ITEM ( '' )  );
#5518=EDGE_CURVE ( 'NONE', #7315, #4695, #17212, .T. ) ;
#5521=CARTESIAN_POINT ( 'NONE',  ( -4.243569643749998122, -24.72177138296861898, -15.29635856794140025 ) ) ;
#5525=CARTESIAN_POINT ( 'NONE',  ( -2.121784821874996396, -23.73980856491443703, -16.02971538246313443 ) ) ;
#5528=CARTESIAN_POINT ( 'NONE',  ( -5.279047395330986450E-15, -25.18333289940175845, -3.631410801825742496 ) ) ;
#5531=CARTESIAN_POINT ( 'NONE',  ( 2.000000000000004441, -22.58441051342866857, -14.01187765139572150 ) ) ;
#5537=CARTESIAN_POINT ( 'NONE',  ( -2.121784821874996396, -21.96530646495340378, -13.49546374544405403 ) ) ;
#5539=EDGE_CURVE ( 'NONE', #5080, #15989, #4665, .T. ) ;
#5545=DIRECTION ( 'NONE',  ( -0.000000000000000000, 1.000000000000000000, -0.000000000000000000 ) ) ;
#5547=( BOUNDED_CURVE ( )  B_SPLINE_CURVE ( 2, ( #11868, #8804, #17561, #14768, #14863, #2067, #9454, #6494, #10843 ),
 .UNSPECIFIED., .F., .F. ) 
 B_SPLINE_CURVE_WITH_KNOTS ( ( 3, 2, 2, 2, 3 ),
 ( 0.6465517241379310498, 0.6494252873563218786, 0.6551724137931034253, 0.6609195402298850830, 0.6637931034482759118 ),
 .UNSPECIFIED. ) 
 CURVE ( )  GEOMETRIC_REPRESENTATION_ITEM ( )  RATIONAL_B_SPLINE_CURVE ( ( 0.9330127018922194093, 0.9330127018922194093, 1.000000000000000000, 0.8660254037844387076, 1.000000000000000000, 0.8660254037844387076, 1.000000000000000000, 0.9330127018922180770, 0.9330127018922194093 ) ) 
 REPRESENTATION_ITEM ( '' )  );
#5548=CARTESIAN_POINT ( 'NONE',  ( 4.243569643749996345, -24.25100835891830542, -6.081059070213228779 ) ) ;
#5549=ORIENTED_EDGE ( 'NONE', *, *, #3031, .F. ) ;
#5550=CARTESIAN_POINT ( 'NONE',  ( 15.00000000000000355, -4.000000000000000000, 30.00000000000000000 ) ) ;
#5552=CARTESIAN_POINT ( 'NONE',  ( -4.000000000000004441, -26.69002267167174125, -9.809504703950437943 ) ) ;
#5558=CARTESIAN_POINT ( 'NONE',  ( 1.999999999999994449, -29.12002700728503513, -11.26675159869200904 ) ) ;
#5563=CARTESIAN_POINT ( 'NONE',  ( -5.279047395330986450E-15, -27.95800890954496865, -7.594058815066988544 ) ) ;
#5565=CARTESIAN_POINT ( 'NONE',  ( -1.071796769724486786, -22.37050183521355962, -14.64069472084458035 ) ) ;
#5567=CARTESIAN_POINT ( 'NONE',  ( 4.243569643750003451, -21.45238569576768484, -10.62719191549412656 ) ) ;
#5569=CARTESIAN_POINT ( 'NONE',  ( -1.999999999999996225, -22.02517348798640029, -13.21320440821394904 ) ) ;
#5570=MECHANICAL_DESIGN_GEOMETRIC_PRESENTATION_REPRESENTATION('',(#14771),#3504);
#5571=CARTESIAN_POINT ( 'NONE',  ( 1.533898589781675205E-14, -26.74131502120161841, -6.935288495286759058 ) ) ;
#5572=VERTEX_POINT ( 'NONE', #14513 ) ;
#5576=B_SPLINE_CURVE_WITH_KNOTS ( 'NONE', 1,
 ( #13305, #4867 ),
 .UNSPECIFIED., .F., .F.,
 ( 2, 2 ),
 ( 0.000000000000000000, 0.9777443369282337038 ),
 .UNSPECIFIED. ) ;
#5581=CARTESIAN_POINT ( 'NONE',  ( 1.999999999999994449, -25.76460485463143968, -6.474712139601389360 ) ) ;
#5584=ADVANCED_FACE ( 'NONE', ( #13194, #9119 ), #11897, .F. ) ;
#5585=CARTESIAN_POINT ( 'NONE',  ( 4.730628863548789710E-15, -19.40242359420666318, -11.97103273789424449 ) ) ;
#5587=EDGE_CURVE ( 'NONE', #94, #12048, #8835, .T. ) ;
#5589=DIRECTION ( 'NONE',  ( 0.000000000000000000, 0.000000000000000000, -1.000000000000000000 ) ) ;
#5590=DIRECTION ( 'NONE',  ( -1.000000000000000000, 0.000000000000000000, -0.000000000000000000 ) ) ;
#5593=CARTESIAN_POINT ( 'NONE',  ( 4.243569643750000786, -24.02932114822622722, -10.03594703378452024 ) ) ;
#5594=VECTOR ( 'NONE', #16059, 999.9999999999998863 ) ;
#5596=CARTESIAN_POINT ( 'NONE',  ( 0.000000000000000000, -9.999999999999998224, -3.075850967158335614 ) ) ;
#5598=CARTESIAN_POINT ( 'NONE',  ( -4.243569643749997233, -18.26903647401939779, -6.080898069690205965 ) ) ;
#5600=DIRECTION ( 'NONE',  ( -0.000000000000000000, -0.5735764363510414965, -0.8191520442889950182 ) ) ;
#5602=ORIENTED_EDGE ( 'NONE', *, *, #17851, .F. ) ;
#5605=CARTESIAN_POINT ( 'NONE',  ( -2.000000000000005773, -24.96876754848942070, -5.338138677143647648 ) ) ;
#5608=EDGE_LOOP ( 'NONE', ( #13833, #16361, #11582, #2797 ) ) ;
#5609=CARTESIAN_POINT ( 'NONE',  ( -2.121784821874996396, -16.80311853779403108, -6.123095346843099307 ) ) ;
#5611=AXIS2_PLACEMENT_3D ( 'NONE', #3576, #7738, #9226 ) ;
#5612=AXIS2_PLACEMENT_3D ( 'NONE', #15653, #448, #10352 ) ;
#5613=DIRECTION ( 'NONE',  ( 0.000000000000000000, 0.000000000000000000, 1.000000000000000000 ) ) ;
#5614=CARTESIAN_POINT ( 'NONE',  ( 2.121784821874994176, -29.88969486959749844, -11.99819291526277532 ) ) ;
#5618=CARTESIAN_POINT ( 'NONE',  ( 4.243569643749996345, -28.09038562974308562, -11.56425806667268752 ) ) ;
#5621=CARTESIAN_POINT ( 'NONE',  ( -2.000000000000005773, -24.77518550192588620, -5.061674863202877184 ) ) ;
#5622=AXIS2_PLACEMENT_3D ( 'NONE', #412, #7438, #14697 ) ;
#5625=ORIENTED_EDGE ( 'NONE', *, *, #15651, .F. ) ;
#5631=( BOUNDED_SURFACE ( )  B_SPLINE_SURFACE ( 3, 2, ( 
 ( #14199, #7138, #12800 ),
 ( #2982, #8613, #17655 ),
 ( #5095, #9271, #7971 ),
 ( #9358, #14954, #667 ),
 ( #13355, #14765, #16429 ),
 ( #7873, #9001, #10753 ),
 ( #15034, #758, #5007 ),
 ( #7599, #16242, #13257 ),
 ( #6218, #13444, #3537 ),
 ( #2337, #10662, #6312 ),
 ( #16155, #4735, #3623 ),
 ( #12137, #10382, #577 ),
 ( #17744, #11866, #14861 ),
 ( #17560, #9181, #476 ),
 ( #17466, #9086, #3447 ),
 ( #2065, #2248, #10568 ),
 ( #11963, #848, #4917 ),
 ( #6120, #6492, #16333 ) ),
 .UNSPECIFIED., .F., .F., .T. ) 
 B_SPLINE_SURFACE_WITH_KNOTS ( ( 4, 2, 2, 2, 2, 2, 2, 2, 4 ),
 ( 3, 3 ),
 ( 2.111895852752043279, 2.369320052961480627, 2.626744253170918419, 2.884168453380356212, 3.141592653589794004, 3.399016853799231797, 3.656441054008669145, 3.913865254218106493, 4.171289454427544285 ),
 ( 0.000000000000000000, 1.000000000000000000 ),
 .UNSPECIFIED. ) 
 GEOMETRIC_REPRESENTATION_ITEM ( )  RATIONAL_B_SPLINE_SURFACE ( (
 ( 1.000000000000000000, 0.8431867568967628124, 1.000000000000000000),
 ( 1.000000000000000000, 0.8610519948705480653, 1.000000000000000000),
 ( 1.000000000000000000, 0.8769588753629522504, 1.000000000000000000),
 ( 1.000000000000000000, 0.9044902796583812465, 1.000000000000000000),
 ( 1.000000000000000000, 0.9161132904341801053, 1.000000000000000000),
 ( 1.000000000000000000, 0.9348125421780860700, 1.000000000000000000),
 ( 1.000000000000000000, 0.9418889734927624602, 1.000000000000000000),
 ( 1.000000000000000000, 0.9513411404402907223, 1.000000000000000000),
 ( 1.000000000000000000, 0.9537169507482278208, 1.000000000000000000),
 ( 1.000000000000000000, 0.9537169507482278208, 1.000000000000000000),
 ( 1.000000000000000000, 0.9513411404402374316, 1.000000000000000000),
 ( 1.000000000000000000, 0.9418889734928156399, 1.000000000000000000),
 ( 1.000000000000000000, 0.9348125421780860700, 1.000000000000000000),
 ( 1.000000000000000000, 0.9161132904341801053, 1.000000000000000000),
 ( 1.000000000000000000, 0.9044902796583805804, 1.000000000000000000),
 ( 1.000000000000000000, 0.8769588753629515843, 1.000000000000000000),
 ( 1.000000000000000000, 0.8610519948705490645, 1.000000000000000000),
 ( 1.000000000000000000, 0.8431867568967623683, 1.000000000000000000) ) ) 
 REPRESENTATION_ITEM ( '' )  SURFACE ( )  );
#5633=CARTESIAN_POINT ( 'NONE',  ( 4.243569643749997233, -28.12264930428783671, -11.61033536916394304 ) ) ;
#5637=CARTESIAN_POINT ( 'NONE',  ( -5.577813053751546416E-15, -28.80619019206536535, -9.884235854727139170 ) ) ;
#5640=CARTESIAN_POINT ( 'NONE',  ( -2.121784821874996396, -20.15854069044762298, -10.91513480593371987 ) ) ;
#5641=VERTEX_POINT ( 'NONE', #14893 ) ;
#5644=CARTESIAN_POINT ( 'NONE',  ( 3.999999999999996447, -26.08776741350315476, -8.949395057446990265 ) ) ;
#5645=CARTESIAN_POINT ( 'NONE',  ( -1.071796769724477238, -23.65552896562483198, -2.528329290782095118 ) ) ;
#5646=CARTESIAN_POINT ( 'NONE',  ( -2.000000000000005773, -28.58229909750097875, -10.49879655616431506 ) ) ;
#5650=CARTESIAN_POINT ( 'NONE',  ( -2.000000000000005773, -29.16304524001135334, -11.32818800201368781 ) ) ;
#5653=CARTESIAN_POINT ( 'NONE',  ( 4.713407268011036227E-15, -19.48762356985234945, -11.60236650416142723 ) ) ;
#5655=CARTESIAN_POINT ( 'NONE',  ( 1.071796769724476128, -17.48947670584981751, -7.669868411485510684 ) ) ;
#5656=( BOUNDED_CURVE ( )  B_SPLINE_CURVE ( 2, ( #2088, #17490, #7718, #16086, #1805, #3379, #7811, #15991, #14884 ),
 .UNSPECIFIED., .F., .T. ) 
 B_SPLINE_CURVE_WITH_KNOTS ( ( 3, 2, 2, 2, 3 ),
 ( 0.1982758620689655249, 0.2011494252873563260, 0.2068965517241379282, 0.2126436781609195303, 0.2155172413793103592 ),
 .UNSPECIFIED. ) 
 CURVE ( )  GEOMETRIC_REPRESENTATION_ITEM ( )  RATIONAL_B_SPLINE_CURVE ( ( 0.9330127018922194093, 0.9330127018922194093, 1.000000000000000000, 0.8660254037844387076, 1.000000000000000000, 0.8660254037844387076, 1.000000000000000000, 0.9330127018922189652, 0.9330127018922192983 ) ) 
 REPRESENTATION_ITEM ( '' )  );
#5658=CARTESIAN_POINT ( 'NONE',  ( -8.999999999999998224, -10.00000000000000178, 15.14468620625656747 ) ) ;
#5659=CARTESIAN_POINT ( 'NONE',  ( 4.243569643749997233, -24.73496347708949017, -6.772218607582066952 ) ) ;
#5662=CARTESIAN_POINT ( 'NONE',  ( -4.000000000000004441, -26.69002267167174125, -9.809504703950439719 ) ) ;
#5673=CARTESIAN_POINT ( 'NONE',  ( -4.243569643749997233, -21.10823983395705383, -10.13570068892072840 ) ) ;
#5677=CARTESIAN_POINT ( 'NONE',  ( 3.579096709490575479E-14, -24.41833045397989821, -3.617722715916328546 ) ) ;
#5680=CARTESIAN_POINT ( 'NONE',  ( 2.121784821874994176, -25.53409880605677884, -5.777757078943218438 ) ) ;
#5684=LINE ( 'NONE', #3182, #6227 ) ;
#5686=CARTESIAN_POINT ( 'NONE',  ( -5.577813053751546416E-15, -24.16022105762192851, -3.249104295986281699 ) ) ;
#5687=CARTESIAN_POINT ( 'NONE',  ( 4.243569643749996345, -23.18630709894168263, -4.560508088001781424 ) ) ;
#5698=ORIENTED_EDGE ( 'NONE', *, *, #7710, .F. ) ;
#5700=CARTESIAN_POINT ( 'NONE',  ( 2.121784821875004390, -17.10424616687832966, -6.553150170094818705 ) ) ;
#5703=CARTESIAN_POINT ( 'NONE',  ( 8.500000000000019540, 0.000000000000000000, -20.49999999999998934 ) ) ;
#5706=CARTESIAN_POINT ( 'NONE',  ( 4.730628863548789710E-15, -22.24162695414431568, -16.02583535712476959 ) ) ;
#5707=LINE ( 'NONE', #17221, #6416 ) ;
#5708=DIRECTION ( 'NONE',  ( 1.049727191973305394E-16, 0.5150380737757255245, -0.8571673013836856869 ) ) ;
#5710=CARTESIAN_POINT ( 'NONE',  ( -4.243569643750000786, -24.90044036093436119, -11.28003420104843357 ) ) ;
#5714=CARTESIAN_POINT ( 'NONE',  ( 4.000000000000000888, -20.56097613501849608, -5.082637016477885794 ) ) ;
#5718=CARTESIAN_POINT ( 'NONE',  ( -4.648177544792955347E-16, -30.09673717385520675, -11.72732795437737785 ) ) ;
#5719=CARTESIAN_POINT ( 'NONE',  ( -1.999999999999996225, -20.21840771348061949, -10.63287546870361666 ) ) ;
#5722=CARTESIAN_POINT ( 'NONE',  ( 4.243569643750000786, -24.80364933730013277, -11.14180229357466345 ) ) ;
#5726=CIRCLE ( 'NONE', #10465, 3.000000000000000444 ) ;
#5727=CARTESIAN_POINT ( 'NONE',  ( 1.999999999999994449, -22.92540149469378363, -2.419909520370864264 ) ) ;
#5728=CARTESIAN_POINT ( 'NONE',  ( 1.999999999999994449, -24.15142112668919339, -4.170847014031824784 ) ) ;
#5731=CARTESIAN_POINT ( 'NONE',  ( 2.121784821874994176, -24.50166122062490359, -4.303283399223027494 ) ) ;
#5732=ORIENTED_EDGE ( 'NONE', *, *, #6928, .F. ) ;
#5733=CARTESIAN_POINT ( 'NONE',  ( -5.577813053751546416E-15, -26.41867827504920996, -6.474515469367432274 ) ) ;
#5734=ORIENTED_EDGE ( 'NONE', *, *, #4354, .F. ) ;
#5737=DIRECTION ( 'NONE',  ( 0.000000000000000000, 0.000000000000000000, 1.000000000000000000 ) ) ;
#5742=CARTESIAN_POINT ( 'NONE',  ( -2.000000000000005773, -29.42115463636932304, -11.69680642194373554 ) ) ;
#5745=CARTESIAN_POINT ( 'NONE',  ( 4.000000000000003553, -21.93861120840455214, -11.07642170763079292 ) ) ;
#5746=ORIENTED_EDGE ( 'NONE', *, *, #7254, .T. ) ;
#5752=CARTESIAN_POINT ( 'NONE',  ( 9.000000000000005329, -10.00000000000000000, 15.14468620625654616 ) ) ;
#5753=CARTESIAN_POINT ( 'NONE',  ( -4.243569643750004339, -25.33721873525807666, -7.632328254085517294 ) ) ;
#5754=ADVANCED_FACE ( 'NONE', ( #4017 ), #2464, .F. ) ;
#5758=VERTEX_POINT ( 'NONE', #5127 ) ;
#5763=EDGE_LOOP ( 'NONE', ( #12953, #18129, #643, #949 ) ) ;
#5765=CARTESIAN_POINT ( 'NONE',  ( -4.243569643749997233, -20.59202104124112154, -9.398463849060638253 ) ) ;
#5769=CARTESIAN_POINT ( 'NONE',  ( 1.071796769724494780, -28.27844469863059018, -9.130537180211129922 ) ) ;
#5770=CARTESIAN_POINT ( 'NONE',  ( -4.243569643750000786, -22.35161007189942595, -7.639927304239214401 ) ) ;
#5771=CARTESIAN_POINT ( 'NONE',  ( -4.242943609565101859, -15.02914320863489550, -7.979206348032058749 ) ) ;
#5773=CARTESIAN_POINT ( 'NONE',  ( -5.577813053751546416E-15, -23.32136551875358421, -2.051094430206859887 ) ) ;
#5774=CARTESIAN_POINT ( 'NONE',  ( -2.121784821874996396, -17.80329244868115168, -7.551491724072033840 ) ) ;
#5777=VERTEX_POINT ( 'NONE', #3925 ) ;
#5783=EDGE_CURVE ( 'NONE', #10810, #7195, #9662, .T. ) ;
#5785=CARTESIAN_POINT ( 'NONE',  ( -2.121784821875005722, -23.51224186791935011, -2.890246122824515318 ) ) ;
#5787=CARTESIAN_POINT ( 'NONE',  ( 4.243569643750003451, -24.84007152296602428, -15.46530867707600088 ) ) ;
#5789=CARTESIAN_POINT ( 'NONE',  ( -4.243569643750000786, -25.67476855000827030, -12.38588946083857856 ) ) ;
#5793=CONICAL_SURFACE ( 'NONE', #6402, 2.000000000000001776, 1.029744260000000189 ) ;
#5794=CARTESIAN_POINT ( 'NONE',  ( 2.121784821874994176, -28.34103849144968379, -9.786482395682487123 ) ) ;
#5796=CARTESIAN_POINT ( 'NONE',  ( -3.999999999999997335, -18.04546114737679474, -5.516427208026009055 ) ) ;
#5798=ORIENTED_EDGE ( 'NONE', *, *, #10968, .T. ) ;
#5800=CARTESIAN_POINT ( 'NONE',  ( 4.243569643750000786, -27.12663390452184942, -14.45936807294509308 ) ) ;
#5806=ORIENTED_EDGE ( 'NONE', *, *, #13858, .T. ) ;
#5807=CARTESIAN_POINT ( 'NONE',  ( -4.243569643750004339, -26.40191999523469946, -9.152879236296964649 ) ) ;
#5808=EDGE_CURVE ( 'NONE', #8825, #1458, #3832, .T. ) ;
#5810=AXIS2_PLACEMENT_3D ( 'NONE', #17125, #14618, #17411 ) ;
#5812=DIRECTION ( 'NONE',  ( 0.000000000000000000, 0.8191520442889952403, -0.5735764363510413855 ) ) ;
#5813=CARTESIAN_POINT ( 'NONE',  ( 4.000000000000003553, -20.90617362297267690, -9.601948027910603756 ) ) ;
#5814=CARTESIAN_POINT ( 'NONE',  ( 1.999999999999994449, -24.92574931576309538, -5.276702273821968880 ) ) ;
#5815=CARTESIAN_POINT ( 'NONE',  ( -3.706921591972381904E-14, -19.73640722255826319, -10.87881775021074127 ) ) ;
#5816=CARTESIAN_POINT ( 'NONE',  ( 6.428571428571431490, -11.73421655796352425, 14.25837509840157935 ) ) ;
#5817=CARTESIAN_POINT ( 'NONE',  ( 4.243569643749996345, -22.96046137712846047, -4.237966970562988323 ) ) ;
#5818=ORIENTED_EDGE ( 'NONE', *, *, #16301, .T. ) ;
#5823=CARTESIAN_POINT ( 'NONE',  ( -4.000000000000004441, -27.65793290730917064, -11.19182377768135161 ) ) ;
#5829=CARTESIAN_POINT ( 'NONE',  ( -4.000000000000000888, -22.94848805062475350, -8.492357399824065567 ) ) ;
#5835=CARTESIAN_POINT ( 'NONE',  ( 2.121784821875004390, -18.87874826683935936, -9.087401807113897334 ) ) ;
#5841=CLOSED_SHELL ( 'NONE', ( #16256, #13680, #13353, #8347, #7664, #5275, #1048, #14083, #3278, #5906, #16991, #14251, #3756, #12480, #7056, #9974, #15585, #30, #9862, #7992, #13011, #10103, #15120, #3764, #1928, #3104, #1406, #12430, #17952, #9351, #12248, #6362, #1811, #6547, #16352, #4045, #6675, #8872, #17956, #79, #3043, #17500, #2260, #16716, #840, #6931, #2095, #491, #16151, #11505, #17971, #3386, #7328, #9390, #615, #7604, #5754, #3436, #18357, #10399, #6139, #12717, #12110, #8432, #7833, #9095, #3307, #11645, #8628, #9982, #9140, #1124, #890, #6487, #6769, #267, #18298, #2486, #9934, #5584, #5454, #9030, #715, #17737, #9594, #1284, #6391, #5015, #1963, #9040, #15295, #18363, #15167, #1669, #3884, #17261, #9760, #16435, #5363, #13817, #6446, #8450, #9422, #2881, #15679, #8005, #15567, #14361, #9305 ) ) ;
#5843=CARTESIAN_POINT ( 'NONE',  ( -4.000000000000000888, -26.11032815671481444, -13.00793304497391567 ) ) ;
#5846=VERTEX_POINT ( 'NONE', #2639 ) ;
#5849=CARTESIAN_POINT ( 'NONE',  ( -1.071796769724486786, -23.14483002428746161, -15.74654998063472533 ) ) ;
#5850=CARTESIAN_POINT ( 'NONE',  ( 4.243569643750000786, -22.19029169917569888, -7.409540791782929681 ) ) ;
#5854=CARTESIAN_POINT ( 'NONE',  ( -1.071796769724477238, -24.42985715469874108, -3.634184550572240546 ) ) ;
#5855=DIRECTION ( 'NONE',  ( 0.000000000000000000, 0.000000000000000000, -1.000000000000000000 ) ) ;
#5856=EDGE_CURVE ( 'NONE', #6787, #14266, #2277, .T. ) ;
#5857=CARTESIAN_POINT ( 'NONE',  ( -2.121784821874996396, -19.90043129408965328, -10.54651638600367214 ) ) ;
#5858=CARTESIAN_POINT ( 'NONE',  ( -7.144308362346979635, -13.70017171021367020, 0.6967212589853186699 ) ) ;
#5862=DIRECTION ( 'NONE',  ( -0.000000000000000000, 1.000000000000000000, -0.000000000000000000 ) ) ;
#5863=CARTESIAN_POINT ( 'NONE',  ( -3.999999999999997335, -22.88501232838376254, -12.42802258070763877 ) ) ;
#5864=CARTESIAN_POINT ( 'NONE',  ( 4.243569643750003451, -18.61318233583002879, -6.572389296263599689 ) ) ;
#5867=EDGE_LOOP ( 'NONE', ( #4127, #15925, #15176, #4420 ) ) ;
#5869=CARTESIAN_POINT ( 'NONE',  ( 2.121784821875004390, -23.52471740128279620, -15.72253336585475658 ) ) ;
#5875=DIRECTION ( 'NONE',  ( 0.8191520442889951292, 0.4698463103929522156, -0.3289899283371602867 ) ) ;
#5876=VERTEX_POINT ( 'NONE', #10783 ) ;
#5877=CARTESIAN_POINT ( 'NONE',  ( 2.121784821875004390, -16.84613677052036351, -6.184531750164772745 ) ) ;
#5879=CARTESIAN_POINT ( 'NONE',  ( -5.330712181944245322E-15, -30.43072080220681386, -10.63511296669387818 ) ) ;
#5880=CARTESIAN_POINT ( 'NONE',  ( 4.243569643750000786, -25.54571385182929077, -12.20158025087355114 ) ) ;
#5881=CYLINDRICAL_SURFACE ( 'NONE', #17690, 4.000000000000000000 ) ;
#5884=CARTESIAN_POINT ( 'NONE',  ( 0.000000000000000000, 5.977523610840987267, 32.81826849749789687 ) ) ;
#5885=CARTESIAN_POINT ( 'NONE',  ( -2.121784821874996396, -22.19115218676662238, -13.81800486288284624 ) ) ;
#5886=CARTESIAN_POINT ( 'NONE',  ( 6.428571428571432378, -14.26578344203647752, -2.827263138854379410 ) ) ;
#5887=CARTESIAN_POINT ( 'NONE',  ( 4.713407268011036227E-15, -17.22916635242506800, -8.376955330780271325 ) ) ;
#5889=ORIENTED_EDGE ( 'NONE', *, *, #12881, .T. ) ;
#5891=CARTESIAN_POINT ( 'NONE',  ( 4.243569643750000786, -27.09437022997710187, -14.41329077045383578 ) ) ;
#5895=ORIENTED_EDGE ( 'NONE', *, *, #13971, .T. ) ;
#5896=CARTESIAN_POINT ( 'NONE',  ( 4.730628863548789710E-15, -19.95090606146734658, -12.75434688024559904 ) ) ;
#5897=CONICAL_SURFACE ( 'NONE', #13903, 2.000000000000001776, 1.029744260000000189 ) ;
#5901=CARTESIAN_POINT ( 'NONE',  ( 2.000000000000004441, -19.93878920005454347, -10.23353884610596509 ) ) ;
#5903=CARTESIAN_POINT ( 'NONE',  ( -5.330712181944245322E-15, -29.39828321677494216, -9.160639286973687234 ) ) ;
#5904=CARTESIAN_POINT ( 'NONE',  ( 4.299564228933482956E-15, -17.92964144805248594, -8.298488810700408891 ) ) ;
#5906=ADVANCED_FACE ( 'NONE', ( #9388 ), #975, .F. ) ;
#5907=CARTESIAN_POINT ( 'NONE',  ( -1.071796769724477238, -23.84911101218836293, -2.804793104722865582 ) ) ;
#5908=CARTESIAN_POINT ( 'NONE',  ( 4.730628863548789710E-15, -17.62792149424562638, -9.436781100875167638 ) ) ;
#5914=ORIENTED_EDGE ( 'NONE', *, *, #15782, .T. ) ;
#5915=CARTESIAN_POINT ( 'NONE',  ( 3.999999999999993339, 0.000000000000000000, -4.999999999999997335 ) ) ;
#5916=DIRECTION ( 'NONE',  ( 0.7601375407242620952, 0.6497622020259954390, 0.000000000000000000 ) ) ;
#5923=CARTESIAN_POINT ( 'NONE',  ( -5.279047395330986450E-15, -27.44179011682903635, -6.856821975206893960 ) ) ;
#5925=EDGE_CURVE ( 'NONE', #4535, #2915, #8816, .T. ) ;
#5926=AXIS2_PLACEMENT_3D ( 'NONE', #17300, #5862, #5951 ) ;
#5929=CARTESIAN_POINT ( 'NONE',  ( -7.036060484405130211, -13.81968884013468291, -0.02068784084667009762 ) ) ;
#5930=CARTESIAN_POINT ( 'NONE',  ( -2.121784821874996396, -18.31951124139709464, -8.288728563932130200 ) ) ;
#5937=CARTESIAN_POINT ( 'NONE',  ( -3.999999999999997335, -24.69177810288954333, -15.00835152021797114 ) ) ;
#5938=ORIENTED_EDGE ( 'NONE', *, *, #5024, .T. ) ;
#5941=CARTESIAN_POINT ( 'NONE',  ( 0.000000000000000000, -27.20729309053124112, -14.57456132866985499 ) ) ;
#5942=CARTESIAN_POINT ( 'NONE',  ( -2.121784821875005722, -25.80296276059631921, -6.161734599703687643 ) ) ;
#5946=CARTESIAN_POINT ( 'NONE',  ( 1.071796769724495224, -16.45703912041794936, -6.195394731765314411 ) ) ;
#5947=CARTESIAN_POINT ( 'NONE',  ( -4.000000000000004441, -28.94847988909901915, -13.03491587733159385 ) ) ;
#5948=CARTESIAN_POINT ( 'NONE',  ( -4.243569643749997233, -20.88239411214383523, -9.813159571481939736 ) ) ;
#5949=CYLINDRICAL_SURFACE ( 'NONE', #9217, 4.000000000000000000 ) ;
#5950=CARTESIAN_POINT ( 'NONE',  ( -5.562324373798915644, -10.00000000000000178, -9.830817939998720334 ) ) ;
#5951=DIRECTION ( 'NONE',  ( 0.000000000000000000, 0.000000000000000000, 1.000000000000000000 ) ) ;
#5952=ORIENTED_EDGE ( 'NONE', *, *, #17851, .T. ) ;
#5953=CARTESIAN_POINT ( 'NONE',  ( -5.330712181944245322E-15, -25.23626920050269362, -3.216667265601666603 ) ) ;
#5956=EDGE_LOOP ( 'NONE', ( #17139, #13510, #439, #7516 ) ) ;
#5959=DIRECTION ( 'NONE',  ( -0.000000000000000000, -1.000000000000000000, -0.000000000000000000 ) ) ;
#5961=CARTESIAN_POINT ( 'NONE',  ( 0.000000000000000000, 0.000000000000000000, -30.00000000000000000 ) ) ;
#5962=CARTESIAN_POINT ( 'NONE',  ( 7.951672694476628500, -10.00000000000000178, -6.265341990737701927 ) ) ;
#5965=CARTESIAN_POINT ( 'NONE',  ( 4.243569643750003451, -24.32385273025008843, -14.72807183721590718 ) ) ;
#5970=CARTESIAN_POINT ( 'NONE',  ( 2.121784821874994176, -28.85725728416562674, -10.52371923554258260 ) ) ;
#5973=CARTESIAN_POINT ( 'NONE',  ( -1.071796769724496334, -21.33806424978168081, -13.16622104112438407 ) ) ;
#5976=CARTESIAN_POINT ( 'NONE',  ( 4.243569643750000786, -24.51327626639741553, -10.72710657115335842 ) ) ;
#5978=CARTESIAN_POINT ( 'NONE',  ( -4.000000000000000888, -20.94814022955544175, -5.635564646372960951 ) ) ;
#5987=VERTEX_POINT ( 'NONE', #16834 ) ;
#5988=CARTESIAN_POINT ( 'NONE',  ( -4.243569643750004339, -26.66002939159266916, -9.521497656227012385 ) ) ;
#5990=ORIENTED_EDGE ( 'NONE', *, *, #17333, .T. ) ;
#5992=CARTESIAN_POINT ( 'NONE',  ( 1.999999999999994449, -25.70007750483700448, -6.382557533612111200 ) ) ;
#5993=CARTESIAN_POINT ( 'NONE',  ( -4.243569643750005227, -27.95057637338251411, -11.36458975587725106 ) ) ;
#5995=DIRECTION ( 'NONE',  ( -0.6427862986982413318, -0.6275077727036082464, 0.4393856727322503208 ) ) ;
#5997=CARTESIAN_POINT ( 'NONE',  ( 1.999999999999994449, -26.53893304370534523, -7.580567399391532568 ) ) ;
#5998=( BOUNDED_CURVE ( )  B_SPLINE_CURVE ( 3, ( #12612, #6867, #8434, #13331 ),
 .UNSPECIFIED., .F., .T. ) 
 B_SPLINE_CURVE_WITH_KNOTS ( ( 4, 4 ),
 ( 4.712388980384689674, 6.283185307179585344 ),
 .UNSPECIFIED. ) 
 CURVE ( )  GEOMETRIC_REPRESENTATION_ITEM ( )  RATIONAL_B_SPLINE_CURVE ( ( 1.000000000000000000, 0.8047378541243649375, 0.8047378541243649375, 1.000000000000000000 ) ) 
 REPRESENTATION_ITEM ( '' )  );
#5999=CARTESIAN_POINT ( 'NONE',  ( 2.121784821875004390, -18.39479314866817461, -8.396242269745057385 ) ) ;
#6000=ORIENTED_EDGE ( 'NONE', *, *, #5135, .F. ) ;
#6001=CARTESIAN_POINT ( 'NONE',  ( 1.071796769724476128, -18.97360573420318985, -9.789424325076520716 ) ) ;
#6011=AXIS2_PLACEMENT_3D ( 'NONE', #10987, #15083, #899 ) ;
#6015=CARTESIAN_POINT ( 'NONE',  ( -4.000000000000004441, -24.56062015101355556, -6.768402738520779671 ) ) ;
#6018=CARTESIAN_POINT ( 'NONE',  ( -5.577813053751546416E-15, -24.16022105762192851, -3.249104295986281699 ) ) ;
#6020=CARTESIAN_POINT ( 'NONE',  ( 1.071796769724494780, -27.18147976340427974, -7.563908894501662594 ) ) ;
#6021=CARTESIAN_POINT ( 'NONE',  ( 4.730628863548789710E-15, -17.59565781970088238, -9.390703798383912115 ) ) ;
#6029=CARTESIAN_POINT ( 'NONE',  ( 0.000000000000000000, 5.977523610840987267, 32.81826849749789687 ) ) ;
#6030=ORIENTED_EDGE ( 'NONE', *, *, #11119, .T. ) ;
#6033=CARTESIAN_POINT ( 'NONE',  ( 2.121784821874994176, -23.95317875336422020, -3.519969256871676055 ) ) ;
#6035=EDGE_CURVE ( 'NONE', #15989, #13645, #8698, .T. ) ;
#6038=CARTESIAN_POINT ( 'NONE',  ( 4.299564228933482956E-15, -16.44551241969911359, -6.178932897109397970 ) ) ;
#6040=CARTESIAN_POINT ( 'NONE',  ( 2.000000000000004441, -22.77799255999219952, -14.28834146533649196 ) ) ;
#6041=CARTESIAN_POINT ( 'NONE',  ( -4.243569643750000786, -22.60971946825739209, -8.008545724169261248 ) ) ;
#6044=CARTESIAN_POINT ( 'NONE',  ( -5.463737038710864802, -14.68677294254779220, -5.668536799318995456 ) ) ;
#6047=VERTEX_POINT ( 'NONE', #2733 ) ;
#6048=ORIENTED_EDGE ( 'NONE', *, *, #11270, .T. ) ;
#6051=DIRECTION ( 'NONE',  ( 1.000000000000000000, 0.000000000000000000, 0.000000000000000000 ) ) ;
#6054=CARTESIAN_POINT ( 'NONE',  ( -4.243569643750005227, -27.40209390612182716, -10.58127561352589829 ) ) ;
#6056=DIRECTION ( 'NONE',  ( -1.000000000000000000, 0.000000000000000000, -0.000000000000000000 ) ) ;
#6057=CARTESIAN_POINT ( 'NONE',  ( 5.463737038711272476, -14.68677294254804977, -5.668536799318668606 ) ) ;
#6060=CARTESIAN_POINT ( 'NONE',  ( 2.121784821875004390, -23.55698107582754730, -15.76861066834601210 ) ) ;
#6062=CARTESIAN_POINT ( 'NONE',  ( -4.243569643750004339, -27.91831269883777011, -11.31851245338599732 ) ) ;
#6063=FACE_OUTER_BOUND ( 'NONE', #3865, .T. ) ;
#6065=CARTESIAN_POINT ( 'NONE',  ( 1.071796769724490339, -22.65166463300919730, -15.04223681008646096 ) ) ;
#6066=CARTESIAN_POINT ( 'NONE',  ( -5.330712181944245322E-15, -29.36601954223019462, -9.114561984482429935 ) ) ;
#6068=CARTESIAN_POINT ( 'NONE',  ( 3.999999999999996447, -22.73234526084956286, -4.157355598356369697 ) ) ;
#6070=EDGE_LOOP ( 'NONE', ( #11748, #14296, #12022, #9434 ) ) ;
#6072=CARTESIAN_POINT ( 'NONE',  ( -2.000000000000005773, -26.58195127643166700, -7.642003802713210447 ) ) ;
#6074=CARTESIAN_POINT ( 'NONE',  ( 4.000000000000000888, -26.49749225125177432, -13.56086067486898372 ) ) ;
#6077=EDGE_CURVE ( 'NONE', #13336, #17808, #18317, .T. ) ;
#6079=CARTESIAN_POINT ( 'NONE',  ( -2.121784821875005722, -26.60955462421497586, -7.313667161985088150 ) ) ;
#6086=CARTESIAN_POINT ( 'NONE',  ( -1.999999999999996225, -19.70218892076468364, -9.895638628843521190 ) ) ;
#6087=CARTESIAN_POINT ( 'NONE',  ( 4.243569643749996345, -27.86453990792986701, -11.24171694923389531 ) ) ;
#6088=CARTESIAN_POINT ( 'NONE',  ( -3.999999999999997335, -23.46575847089413713, -13.25741402655701506 ) ) ;
#6089=CARTESIAN_POINT ( 'NONE',  ( 9.184850993605147944E-16, -10.54254386713301628, 22.30101802474215589 ) ) ;
#6091=CARTESIAN_POINT ( 'NONE',  ( -4.243569643750000786, -21.57728188282551685, -6.534072044449069416 ) ) ;
#6093=CARTESIAN_POINT ( 'NONE',  ( -1.071796769724505882, -16.69209511533825463, -6.531089482383521272 ) ) ;
#6095=CARTESIAN_POINT ( 'NONE',  ( 1.071796769724476128, -19.74793392327709540, -10.89527958486666392 ) ) ;
#6098=AXIS2_PLACEMENT_3D ( 'NONE', #6970, #1064, #4105 ) ;
#6100=FACE_OUTER_BOUND ( 'NONE', #16876, .T. ) ;
#6108=CARTESIAN_POINT ( 'NONE',  ( -4.000000000000004441, -24.30251075465558586, -6.399784318590734600 ) ) ;
#6112=( BOUNDED_CURVE ( )  B_SPLINE_CURVE ( 2, ( #1542, #5973, #15910, #1630, #3208, #7177, #12838, #17412, #8845 ),
 .UNSPECIFIED., .F., .F. ) 
 B_SPLINE_CURVE_WITH_KNOTS ( ( 3, 2, 2, 2, 3 ),
 ( 0.3189655172413793371, 0.3218390804597701105, 0.3275862068965517127, 0.3333333333333333148, 0.3362068965517241437 ),
 .UNSPECIFIED. ) 
 CURVE ( )  GEOMETRIC_REPRESENTATION_ITEM ( )  RATIONAL_B_SPLINE_CURVE ( ( 0.9330127018922194093, 0.9330127018922200755, 1.000000000000000000, 0.8660254037844387076, 1.000000000000000000, 0.8660254037844387076, 1.000000000000000000, 0.9330127018922187432, 0.9330127018922194093 ) ) 
 REPRESENTATION_ITEM ( '' )  );
#6114=CARTESIAN_POINT ( 'NONE',  ( 4.730628863548789710E-15, -17.07943902698494298, -8.653466958523816643 ) ) ;
#6120=CARTESIAN_POINT ( 'NONE',  ( 9.000000000000005329, -10.00000000000000178, 15.14468620625654083 ) ) ;
#6121=FACE_OUTER_BOUND ( 'NONE', #6861, .T. ) ;
#6123=CARTESIAN_POINT ( 'NONE',  ( -2.000000000000005773, -29.35662728657488429, -11.60465181595445650 ) ) ;
#6126=CARTESIAN_POINT ( 'NONE',  ( 4.299564228933482956E-15, -20.83337215778458074, -12.44544603592020771 ) ) ;
#6127=CARTESIAN_POINT ( 'NONE',  ( 2.121784821875004390, -19.13685766319732906, -9.456020227043945070 ) ) ;
#6130=CARTESIAN_POINT ( 'NONE',  ( 4.730628863548789710E-15, -22.53200002504703292, -16.44053107954607640 ) ) ;
#6132=CARTESIAN_POINT ( 'NONE',  ( -2.000000000000005773, -29.09851789021691815, -11.23603339602441054 ) ) ;
#6133=CARTESIAN_POINT ( 'NONE',  ( 4.730628863548789710E-15, -17.62792149424562638, -9.436781100875167638 ) ) ;
#6134=LINE ( 'NONE', #7429, #8608 ) ;
#6135=CARTESIAN_POINT ( 'NONE',  ( -0.6850780354679466555, -10.00000000000000355, -5.037014450716167602 ) ) ;
#6137=CARTESIAN_POINT ( 'NONE',  ( 0.000000000000000000, 5.977523610840987267, 32.81826849749789687 ) ) ;
#6139=ADVANCED_FACE ( 'NONE', ( #203 ), #12895, .T. ) ;
#6141=ORIENTED_EDGE ( 'NONE', *, *, #6657, .T. ) ;
#6143=ORIENTED_EDGE ( 'NONE', *, *, #8299, .T. ) ;
#6144=CARTESIAN_POINT ( 'NONE',  ( 4.243569643750003451, -17.83885414675612324, -5.466534036473456482 ) ) ;
#6145=DIRECTION ( 'NONE',  ( -0.000000000000000000, -0.5735764363510414965, -0.8191520442889950182 ) ) ;
#6150=CARTESIAN_POINT ( 'NONE',  ( 4.243569643749996345, -27.57416683702714622, -10.82702122681259205 ) ) ;
#6152=EDGE_CURVE ( 'NONE', #8381, #1806, #3141, .T. ) ;
#6154=CARTESIAN_POINT ( 'NONE',  ( 4.898587196589413815E-16, 2.700915433685006750, 35.11257424290206330 ) ) ;
#6155=VERTEX_POINT ( 'NONE', #17476 ) ;
#6158=CARTESIAN_POINT ( 'NONE',  ( -2.121784821874996396, -23.25585344674324162, -15.33855584509429271 ) ) ;
#6161=CARTESIAN_POINT ( 'NONE',  ( -5.330712181944246111E-15, -27.81736316408238352, -6.902851464902141743 ) ) ;
#6163=AXIS2_PLACEMENT_3D ( 'NONE', #3858, #1087, #9505 ) ;
#6164=CARTESIAN_POINT ( 'NONE',  ( 4.299564228933482956E-15, -16.96173121241504944, -6.916169736969493442 ) ) ;
#6166=CARTESIAN_POINT ( 'NONE',  ( 4.243569643749996345, -24.73496347708949017, -6.772218607582066952 ) ) ;
#6172=ORIENTED_EDGE ( 'NONE', *, *, #15787, .T. ) ;
#6174=FACE_OUTER_BOUND ( 'NONE', #110, .T. ) ;
#6176=CARTESIAN_POINT ( 'NONE',  ( -3.999999999999997335, -23.46575847089413713, -13.25741402655701151 ) ) ;
#6177=CARTESIAN_POINT ( 'NONE',  ( 4.299564228933482956E-15, -16.96173121241504944, -6.916169736969493442 ) ) ;
#6180=CARTESIAN_POINT ( 'NONE',  ( -2.121784821875005722, -26.09333583149904001, -6.576430322124992678 ) ) ;
#6182=EDGE_LOOP ( 'NONE', ( #3265, #18000, #13060, #2389 ) ) ;
#6184=CARTESIAN_POINT ( 'NONE',  ( 4.000000000000000888, -21.52888637065593258, -6.464956090208799466 ) ) ;
#6186=CARTESIAN_POINT ( 'NONE',  ( -5.330712181944245322E-15, -29.91450200949088156, -9.897876126833780930 ) ) ;
#6188=PLANE ( 'NONE',  #13605 ) ;
#6189=CARTESIAN_POINT ( 'NONE',  ( 1.533898589781675205E-14, -28.22544404955499786, -9.054844408877768203 ) ) ;
#6190=CARTESIAN_POINT ( 'NONE',  ( -2.121784821875005722, -23.25413247156138397, -2.521627702894468470 ) ) ;
#6192=CARTESIAN_POINT ( 'NONE',  ( -1.071796769724486564, -26.75284172192045062, -6.951750329942670170 ) ) ;
#6193=CARTESIAN_POINT ( 'NONE',  ( 2.000000000000004441, -20.00331654984898577, -10.32569345209524414 ) ) ;
#6197=CARTESIAN_POINT ( 'NONE',  ( -1.071796769724477238, -24.62343920126227559, -3.910648364513010122 ) ) ;
#6206=CARTESIAN_POINT ( 'NONE',  ( -1.999999999999996225, -19.89577096732821104, -10.17210244278429343 ) ) ;
#6209=VECTOR ( 'NONE', #11246, 1000.000000000000000 ) ;
#6213=CARTESIAN_POINT ( 'NONE',  ( 2.121784821874994176, -24.46939754608015605, -4.257206096731771083 ) ) ;
#6214=CARTESIAN_POINT ( 'NONE',  ( -2.121784821875005722, -27.64199220964684756, -8.788140841705278206 ) ) ;
#6216=EDGE_CURVE ( 'NONE', #6155, #18310, #6231, .T. ) ;
#6217=ORIENTED_EDGE ( 'NONE', *, *, #15676, .F. ) ;
#6218=CARTESIAN_POINT ( 'NONE',  ( -0.9009846993709869079, -10.00000000000000178, 24.02174733379527538 ) ) ;
#6222=ORIENTED_EDGE ( 'NONE', *, *, #5017, .T. ) ;
#6225=CARTESIAN_POINT ( 'NONE',  ( 4.730628863548789710E-15, -17.07943902698494298, -8.653466958523816643 ) ) ;
#6227=VECTOR ( 'NONE', #8823, 1000.000000000000000 ) ;
#6229=CARTESIAN_POINT ( 'NONE',  ( 4.243569643750000786, -26.35230571544794387, -13.35351281315494987 ) ) ;
#6230=CARTESIAN_POINT ( 'NONE',  ( -3.999999999999997335, -24.43366870653157363, -14.63973310028792696 ) ) ;
#6231=( BOUNDED_CURVE ( )  B_SPLINE_CURVE ( 2, ( #11596, #14588, #17572, #10395, #17292, #11689, #679, #14495, #10200, #15879, #3176, #488, #16255, #2075, #4927, #8814, #17380, #14778, #4645, #14687, #16073, #1793, #10298, #3274, #8911, #1891, #13176, #6130, #1695, #3367, #13365, #1983, #10579, #13270, #7705, #587, #6229, #4841, #10490, #11973, #17665, #3547, #9192, #2594, #5449, #8227, #6924, #5633, #1377, #7799, #2169, #13890, #5268, #13456, #16602, #9619, #9526, #7006, #12306, #12669, #14873, #768, #2686, #6413, #4151, #18359, #17997, #13797, #1201, #11096, #6837, #12579, #11275, #16964, #10923, #3878, #12487, #15206, #2507, #8135, #15293, #16689, #16782, #1105, #5362, #4243, #4051, #18180, #16873, #9703, #15387, #8318, #13979, #14063, #6745, #12400, #1292, #18092, #18267, #11009, #5537, #11184, #3968, #9798, #15479, #2776, #8406, #8486, #5722, #4417, #11362, #15558, #13130, #8668, #12939, #5988, #10060, #11546, #17052, #1469, #14158, #7472, #15737, #15645, #157, #12850, #3128, #5807, #11640, #1644, #251, #3039, #10247, #14345, #11450, #11731, #9886, #2853, #440, #1743, #2945, #8860, #7281, #14440, #7374, #10154, #17427, #5896, #14539, #4324, #7101, #17237, #13035, #4511, #12763, #8580, #1835, #9969, #67, #14253, #1555, #7193, #17140, #15832, #6079, #8763, #4597, #350, #17335, #15926, #3224, #7561, #3314, #16023, #3409, #17526, #10343, #11830, #4693, #1938, #16390, #7929, #17797, #901, #8957, #16204, #13218, #14635, #6180, #17619, #4788, #14998, #534, #2296, #6270, #3678, #3496, #10441, #6542, #9143, #10623, #13585, #12101, #12194, #16117, #7651, #9051, #14727, #6454, #13409, #14821, #2027, #3585, #5059, #720, #13317, #632, #11923, #4879, #10530, #2120, #6367, #7749, #12008, #9235, #17704, #4968, #16297, #14920, #10713, #2212, #7839, #13492, #807, #9324, #11076, #13771, #13956, #9597, #8204, #18066, #9777, #12561, #4129, #15455, #16668, #9680, #17973, #15365, #9502, #16851, #3947, #4033, #2663, #18159, #1354, #5338, #2752, #12284, #16480, #12375, #1084, #8382, #5151, #6903, #8022, #14045, #15273, #10808, #2572, #2390, #15085, #13675, #6985, #12465, #18246, #8297, #6637, #5515, #16760, #996, #1268, #10990, #6815, #15178, #3761, #11160, #17881, #13868, #9410, #5242, #10899, #16576, #3854, #1174, #2482, #5430, #8112, #6721, #3108, #11254, #13014, #133, #15538, #326, #8556, #46, #12830, #5785, #7077, #4303, #17034, #8647, #9950, #228, #11427, #17117, #14231, #4488, #7170, #15622, #8738, #1535, #1622, #1447, #7256, #5700, #14413, #4397, #14325, #12916, #15713, #12646, #10037, #1718, #12744, #16943, #3014, #5877, #11524, #5609, #17215, #2836, #7354, #10130, #4218, #15811, #8465, #9864 ),
 .UNSPECIFIED., .F., .T. ) 
 B_SPLINE_CURVE_WITH_KNOTS ( ( 3, 2, 2, 2, 2, 2, 2, 2, 2, 2, 2, 2, 2, 2, 2, 2, 2, 2, 2, 2, 2, 2, 2, 2, 2, 2, 2, 2, 2, 2, 2, 2, 2, 2, 2, 2, 2, 2, 2, 2, 2, 2, 2, 2, 2, 2, 2, 2, 2, 2, 2, 2, 2, 2, 2, 2, 2, 2, 2, 2, 2, 2, 2, 2, 2, 2, 2, 2, 2, 2, 2, 2, 2, 2, 2, 2, 2, 2, 2, 2, 2, 2, 2, 2, 2, 2, 2, 2, 2, 2, 2, 2, 2, 2, 2, 2, 2, 2, 2, 2, 2, 2, 2, 2, 2, 2, 2, 2, 2, 2, 2, 2, 2, 2, 2, 2, 2, 2, 2, 2, 2, 2, 2, 2, 2, 2, 2, 2, 2, 2, 2, 2, 2, 2, 2, 2, 2, 2, 2, 2, 2, 2, 2, 2, 2, 2, 2, 2, 2, 2, 2, 2, 2, 2, 2, 2, 2, 2, 2, 2, 2, 2, 2, 2, 2, 2, 2, 2, 2, 2, 2, 2, 2, 2, 3 ),
 ( 0.000000000000000000, 0.005769117196331985213, 0.01153823439266397043, 0.01730735158899595477, 0.02307646878532794085, 0.02884558598165992693, 0.03461470317799190954, 0.04038382037432389909, 0.04615293757065588170, 0.05192205476698786432, 0.05769117196331985387, 0.06346028915965185035, 0.06922940635598381909, 0.07499852355231581558, 0.08076764074864779819, 0.08653675794497978080, 0.09230587514131176341, 0.09807499233764375990, 0.1038441095339757286, 0.1096132267303077251, 0.1153823439266397077, 0.1211514611229717042, 0.1269205783193037007, 0.1326896955156356694, 0.1384588127119676382, 0.1442279299082996347, 0.1499970471046316312, 0.1557661643009635999, 0.1615352814972955964, 0.1673043986936275651, 0.1730735158899595616, 0.1788426330862915581, 0.1846117502826235268, 0.1903808674789554956, 0.1961499846752875198, 0.2019191018716194885, 0.2076882190679514573, 0.2134573362642834538, 0.2192264534606154502, 0.2249955706569474467, 0.2307646878532794155, 0.2365338050496113842, 0.2423029222459434084, 0.2480720394422753772, 0.2538411566386074014, 0.2596102738349393424, 0.2653793910312713389, 0.2711485082276033354, 0.2769176254239352764, 0.2826867426202672728, 0.2884558598165992693, 0.2942249770129312103, 0.2999940942092632623, 0.3057632114055952588, 0.3115323286019271998, 0.3173014457982591963, 0.3230705629945911928, 0.3288396801909231337, 0.3346087973872551302, 0.3403779145835871267, 0.3461470317799191232, 0.3519161489762511197, 0.3576852661725831162, 0.3634543833689150572, 0.3692235005652470536, 0.3749926177615790501, 0.3807617349579109911, 0.3865308521542429876, 0.3922999693505750396, 0.3980690865469069806, 0.4038382037432389771, 0.4096073209395709736, 0.4153764381359029145, 0.4211455553322349110, 0.4269146725285669075, 0.4326837897248988485, 0.4384529069212309005, 0.4442220241175628970, 0.4499911413138948935, 0.4557602585102268344, 0.4615293757065588309, 0.4672984929028908274, 0.4730676100992227684, 0.4788367272955547649, 0.4846058444918868169, 0.4903749616882187579, 0.4961440788845507543, 0.5019131960808826953, 0.5076823132772148028, 0.5134514304735466883, 0.5192205476698786848, 0.5249896648662106813, 0.5307587820625426778, 0.5365278992588745632, 0.5422970164552066707, 0.5480661336515386672, 0.5538352508478705527, 0.5596043680442026602, 0.5653734852405345457, 0.5711426024368665422, 0.5769117196331985387, 0.5826808368295305351, 0.5884499540258624206, 0.5942190712221945281, 0.5999881884185265246, 0.6057573056148584101, 0.6115264228111905176, 0.6172955400075224031, 0.6230646572038543995, 0.6288337744001863960, 0.6346028915965183925, 0.6403720087928503890, 0.6461411259891823855, 0.6519102431855143820, 0.6576793603818462675, 0.6634484775781783750, 0.6692175947745102604, 0.6749867119708422569, 0.6807558291671742534, 0.6865249463635062499, 0.6922940635598382464, 0.6980631807561702429, 0.7038322979525022394, 0.7096014151488341248, 0.7153705323451662323, 0.7211396495414981178, 0.7269087667378301143, 0.7326778839341622218, 0.7384470011304941073, 0.7442161183268261038, 0.7499852355231581003, 0.7557543527194900967, 0.7615234699158219822, 0.7672925871121540897, 0.7730617043084859752, 0.7788308215048179717, 0.7845999387011500792, 0.7903690558974819647, 0.7961381730938139611, 0.8019072902901459576, 0.8076764074864779541, 0.8134455246828098396, 0.8192146418791419471, 0.8249837590754739436, 0.8307528762718058291, 0.8365219934681379366, 0.8422911106644698220, 0.8480602278608018185, 0.8538293450571338150, 0.8595984622534658115, 0.8653675794497976970, 0.8711366966461298045, 0.8769058138424618010, 0.8826749310387936864, 0.8884440482351257939, 0.8942131654314576794, 0.8999822826277897869, 0.9057513998241216724, 0.9115205170204536689, 0.9172896342167857764, 0.9230587514131176619, 0.9288278686094496583, 0.9345969858057816548, 0.9403661030021136513, 0.9461352201984455368, 0.9519043373947776443, 0.9576734545911095298, 0.9634425717874415263, 0.9692116889837736338, 0.9749808061801055192, 0.9807499233764375157, 0.9865190405727695122, 0.9922881577691015087, 0.9980572749654333942, 1.000000000000000000 ),
 .UNSPECIFIED. ) 
 CURVE ( )  GEOMETRIC_REPRESENTATION_ITEM ( )  RATIONAL_B_SPLINE_CURVE ( ( 1.000000000000000000, 0.8660254037844387076, 1.000000000000000000, 0.8660254037844387076, 1.000000000000000000, 0.8660254037844387076, 1.000000000000000000, 0.8660254037844387076, 1.000000000000000000, 0.8660254037844387076, 1.000000000000000000, 0.8660254037844387076, 1.000000000000000000, 0.8660254037844387076, 1.000000000000000000, 0.8660254037844387076, 1.000000000000000000, 0.8660254037844387076, 1.000000000000000000, 0.8660254037844387076, 1.000000000000000000, 0.8660254037844387076, 1.000000000000000000, 0.8660254037844387076, 1.000000000000000000, 0.8660254037844387076, 1.000000000000000000, 0.8660254037844387076, 1.000000000000000000, 0.8660254037844387076, 1.000000000000000000, 0.8660254037844387076, 1.000000000000000000, 0.8660254037844387076, 1.000000000000000000, 0.8660254037844387076, 1.000000000000000000, 0.8660254037844387076, 1.000000000000000000, 0.8660254037844387076, 1.000000000000000000, 0.8660254037844387076, 1.000000000000000000, 0.8660254037844387076, 1.000000000000000000, 0.8660254037844387076, 1.000000000000000000, 0.8660254037844387076, 1.000000000000000000, 0.8660254037844387076, 1.000000000000000000, 0.8660254037844387076, 1.000000000000000000, 0.8660254037844387076, 1.000000000000000000, 0.8660254037844387076, 1.000000000000000000, 0.8660254037844387076, 1.000000000000000000, 0.8660254037844387076, 1.000000000000000000, 0.8660254037844387076, 1.000000000000000000, 0.8660254037844387076, 1.000000000000000000, 0.8660254037844387076, 1.000000000000000000, 0.8660254037844387076, 1.000000000000000000, 0.8660254037844387076, 1.000000000000000000, 0.8660254037844387076, 1.000000000000000000, 0.8660254037844387076, 1.000000000000000000, 0.8660254037844387076, 1.000000000000000000, 0.8660254037844387076, 1.000000000000000000, 0.8660254037844387076, 1.000000000000000000, 0.8660254037844387076, 1.000000000000000000, 0.8660254037844387076, 1.000000000000000000, 0.8660254037844387076, 1.000000000000000000, 0.8660254037844387076, 1.000000000000000000, 0.8660254037844387076, 1.000000000000000000, 0.8660254037844387076, 1.000000000000000000, 0.8660254037844387076, 1.000000000000000000, 0.8660254037844387076, 1.000000000000000000, 0.8660254037844387076, 1.000000000000000000, 0.8660254037844387076, 1.000000000000000000, 0.8660254037844387076, 1.000000000000000000, 0.8660254037844387076, 1.000000000000000000, 0.8660254037844387076, 1.000000000000000000, 0.8660254037844387076, 1.000000000000000000, 0.8660254037844387076, 1.000000000000000000, 0.8660254037844387076, 1.000000000000000000, 0.8660254037844387076, 1.000000000000000000, 0.8660254037844387076, 1.000000000000000000, 0.8660254037844387076, 1.000000000000000000, 0.8660254037844387076, 1.000000000000000000, 0.8660254037844387076, 1.000000000000000000, 0.8660254037844387076, 1.000000000000000000, 0.8660254037844387076, 1.000000000000000000, 0.8660254037844387076, 1.000000000000000000, 0.8660254037844387076, 1.000000000000000000, 0.8660254037844387076, 1.000000000000000000, 0.8660254037844387076, 1.000000000000000000, 0.8660254037844387076, 1.000000000000000000, 0.8660254037844387076, 1.000000000000000000, 0.8660254037844387076, 1.000000000000000000, 0.8660254037844387076, 1.000000000000000000, 0.8660254037844387076, 1.000000000000000000, 0.8660254037844387076, 1.000000000000000000, 0.8660254037844387076, 1.000000000000000000, 0.8660254037844387076, 1.000000000000000000, 0.8660254037844387076, 1.000000000000000000, 0.8660254037844387076, 1.000000000000000000, 0.8660254037844387076, 1.000000000000000000, 0.8660254037844387076, 1.000000000000000000, 0.8660254037844387076, 1.000000000000000000, 0.8660254037844387076, 1.000000000000000000, 0.8660254037844387076, 1.000000000000000000, 0.8660254037844387076, 1.000000000000000000, 0.8660254037844387076, 1.000000000000000000, 0.8660254037844387076, 1.000000000000000000, 0.8660254037844387076, 1.000000000000000000, 0.8660254037844387076, 1.000000000000000000, 0.8660254037844387076, 1.000000000000000000, 0.8660254037844387076, 1.000000000000000000, 0.8660254037844387076, 1.000000000000000000, 0.8660254037844387076, 1.000000000000000000, 0.8660254037844387076, 1.000000000000000000, 0.8660254037844387076, 1.000000000000000000, 0.8660254037844387076, 1.000000000000000000, 0.8660254037844387076, 1.000000000000000000, 0.8660254037844387076, 1.000000000000000000, 0.8660254037844387076, 1.000000000000000000, 0.8660254037844387076, 1.000000000000000000, 0.8660254037844387076, 1.000000000000000000, 0.8660254037844387076, 1.000000000000000000, 0.8660254037844387076, 1.000000000000000000, 0.8660254037844387076, 1.000000000000000000, 0.8660254037844387076, 1.000000000000000000, 0.8660254037844387076, 1.000000000000000000, 0.8660254037844387076, 1.000000000000000000, 0.8660254037844387076, 1.000000000000000000, 0.8660254037844387076, 1.000000000000000000, 0.8660254037844387076, 1.000000000000000000, 0.8660254037844387076, 1.000000000000000000, 0.8660254037844387076, 1.000000000000000000, 0.8660254037844387076, 1.000000000000000000, 0.8660254037844387076, 1.000000000000000000, 0.8660254037844387076, 1.000000000000000000, 0.8660254037844387076, 1.000000000000000000, 0.8660254037844387076, 1.000000000000000000, 0.8660254037844387076, 1.000000000000000000, 0.8660254037844387076, 1.000000000000000000, 0.8660254037844387076, 1.000000000000000000, 0.8660254037844387076, 1.000000000000000000, 0.8660254037844387076, 1.000000000000000000, 0.8660254037844387076, 1.000000000000000000, 0.8660254037844387076, 1.000000000000000000, 0.8660254037844387076, 1.000000000000000000, 0.8660254037844387076, 1.000000000000000000, 0.8660254037844387076, 1.000000000000000000, 0.8660254037844387076, 1.000000000000000000, 0.8660254037844387076, 1.000000000000000000, 0.8660254037844387076, 1.000000000000000000, 0.8660254037844387076, 1.000000000000000000, 0.8660254037844387076, 1.000000000000000000, 0.8660254037844387076, 1.000000000000000000, 0.8660254037844387076, 1.000000000000000000, 0.8660254037844387076, 1.000000000000000000, 0.8660254037844387076, 1.000000000000000000, 0.8660254037844387076, 1.000000000000000000, 0.8660254037844387076, 1.000000000000000000, 0.8660254037844387076, 1.000000000000000000, 0.8660254037844387076, 1.000000000000000000, 0.8660254037844387076, 1.000000000000000000, 0.8660254037844387076, 1.000000000000000000, 0.8660254037844387076, 1.000000000000000000, 0.8660254037844387076, 1.000000000000000000, 0.8660254037844387076, 1.000000000000000000, 0.8660254037844387076, 1.000000000000000000, 0.8660254037844387076, 1.000000000000000000, 0.8660254037844387076, 1.000000000000000000, 0.8660254037844387076, 1.000000000000000000, 0.8660254037844387076, 1.000000000000000000, 0.8660254037844387076, 1.000000000000000000, 0.8660254037844387076, 1.000000000000000000, 0.8660254037844387076, 1.000000000000000000, 0.8660254037844387076, 1.000000000000000000, 0.8660254037844387076, 1.000000000000000000, 0.8660254037844387076, 1.000000000000000000, 0.8660254037844387076, 1.000000000000000000, 0.8660254037844387076, 1.000000000000000000, 0.8660254037844387076, 1.000000000000000000, 0.8660254037844387076, 1.000000000000000000, 0.8660254037844387076, 1.000000000000000000, 0.8660254037844387076, 1.000000000000000000, 0.8660254037844387076, 1.000000000000000000, 0.8660254037844387076, 1.000000000000000000, 0.8660254037844387076, 1.000000000000000000, 0.8660254037844387076, 1.000000000000000000, 0.8660254037844387076, 1.000000000000000000, 0.8660254037844387076, 1.000000000000000000, 0.8660254037844387076, 1.000000000000000000, 0.8660254037844387076, 1.000000000000000000, 0.8660254037844387076, 1.000000000000000000, 0.8660254037844387076, 1.000000000000000000, 0.8660254037844387076, 1.000000000000000000, 0.8660254037844387076, 1.000000000000000000, 0.8660254037844387076, 1.000000000000000000, 0.9548846395026606704, 0.9401540804572323662 ) ) 
 REPRESENTATION_ITEM ( '' )  );
#6232=CARTESIAN_POINT ( 'NONE',  ( -4.243569643750005227, -23.04649784258110756, -4.360839777206344081 ) ) ;
#6233=CARTESIAN_POINT ( 'NONE',  ( -7.316366419972956336, -13.46537015260387449, 2.120294839946750720 ) ) ;
#6234=LINE ( 'NONE', #14968, #18295 ) ;
#6236=CARTESIAN_POINT ( 'NONE',  ( 2.000000000000004441, -24.06853954178204447, -16.13143356498672887 ) ) ;
#6238=ORIENTED_EDGE ( 'NONE', *, *, #11282, .F. ) ;
#6239=ORIENTED_EDGE ( 'NONE', *, *, #8243, .T. ) ;
#6240=CARTESIAN_POINT ( 'NONE',  ( -4.000000000000000888, -19.65759324776559680, -3.792472546722722715 ) ) ;
#6244=CARTESIAN_POINT ( 'NONE',  ( -2.121784821875005722, -28.90027551689194496, -10.58515563886426136 ) ) ;
#6247=CARTESIAN_POINT ( 'NONE',  ( -0.9964672492307999896, -9.999999999998728129, -3.740800554895127750 ) ) ;
#6251=CARTESIAN_POINT ( 'NONE',  ( 4.730628863548789710E-15, -20.72523425054125212, -13.86020214003574047 ) ) ;
#6253=CARTESIAN_POINT ( 'NONE',  ( -2.121784821874996396, -20.64249580861881128, -11.60629434330255982 ) ) ;
#6254=FACE_OUTER_BOUND ( 'NONE', #14439, .T. ) ;
#6257=CARTESIAN_POINT ( 'NONE',  ( -4.243569643749997233, -21.36634923031502353, -10.50431910885077791 ) ) ;
#6264=SHAPE_DEFINITION_REPRESENTATION ( #5003, #17791 ) ;
#6266=CARTESIAN_POINT ( 'NONE',  ( 1.999999999999994449, -23.18351089105175333, -2.788527940300912444 ) ) ;
#6270=CARTESIAN_POINT ( 'NONE',  ( 2.121784821875004390, -19.94344952681598926, -10.60795278932534558 ) ) ;
#6272=EDGE_CURVE ( 'NONE', #13551, #6047, #15247, .T. ) ;
#6277=CARTESIAN_POINT ( 'NONE',  ( -5.330712181944245322E-15, -28.88206442405900631, -8.423402447113588210 ) ) ;
#6279=CARTESIAN_POINT ( 'NONE',  ( 2.000000000000004441, -23.81043014542407121, -15.76281514505668113 ) ) ;
#6280=CARTESIAN_POINT ( 'NONE',  ( 6.734712607319251809, -10.37497835385873657, 2.111428012012234401 ) ) ;
#6282=CARTESIAN_POINT ( 'NONE',  ( -4.243569643749997233, -18.55940954492211503, -6.495593792111509224 ) ) ;
#6286=CARTESIAN_POINT ( 'NONE',  ( -5.279047395330986450E-15, -26.47387988119159985, -5.474502901475981176 ) ) ;
#6291=DIRECTION ( 'NONE',  ( -0.000000000000000000, -0.5735764363510414965, -0.8191520442889950182 ) ) ;
#6297=EDGE_LOOP ( 'NONE', ( #2091, #503, #1853, #11768 ) ) ;
#6300=CARTESIAN_POINT ( 'NONE',  ( 1.999999999999994449, -25.44196810847903478, -6.013939113682064352 ) ) ;
#6301=VERTEX_POINT ( 'NONE', #12710 ) ;
#6303=DIRECTION ( 'NONE',  ( -1.214671430232282197E-14, -0.8191520442889844711, 0.5735764363510568176 ) ) ;
#6304=AXIS2_PLACEMENT_3D ( 'NONE', #7485, #9830, #362 ) ;
#6308=CARTESIAN_POINT ( 'NONE',  ( 4.243569643750000786, -19.86730713195397868, -4.091975012412500945 ) ) ;
#6309=CARTESIAN_POINT ( 'NONE',  ( -4.243569643750000786, -24.15837584640520674, -10.22025624374954766 ) ) ;
#6312=CARTESIAN_POINT ( 'NONE',  ( 0.6435604995507229198, -10.54254386713301628, 22.30101802474215233 ) ) ;
#6316=CARTESIAN_POINT ( 'NONE',  ( -4.243569643750005227, -28.72490456245641965, -12.47044501566739427 ) ) ;
#6320=CARTESIAN_POINT ( 'NONE',  ( 9.000000000000005329, -10.00000000000000000, -3.713574246709344884 ) ) ;
#6321=CARTESIAN_POINT ( 'NONE',  ( -2.121784821875005722, -25.02863457152241722, -5.055879339913546211 ) ) ;
#6325=CARTESIAN_POINT ( 'NONE',  ( 2.000000000000004441, -16.90600379355336003, -5.902272412934671308 ) ) ;
#6326=CARTESIAN_POINT ( 'NONE',  ( 3.999999999999996447, -27.57189644185653066, -11.06895097103799763 ) ) ;
#6328=CARTESIAN_POINT ( 'NONE',  ( 4.730628863548789710E-15, -17.36981209788766378, -9.068162680945119902 ) ) ;
#6334=CARTESIAN_POINT ( 'NONE',  ( 3.999999999999996447, -24.53911103535534366, -6.737684537866703849 ) ) ;
#6336=ORIENTED_EDGE ( 'NONE', *, *, #15316, .T. ) ;
#6339=DIRECTION ( 'NONE',  ( 0.000000000000000000, 0.8191520442889952403, -0.5735764363510413855 ) ) ;
#6342=( NAMED_UNIT ( * ) PLANE_ANGLE_UNIT ( ) SI_UNIT ( $, .RADIAN. ) );
#6343=CARTESIAN_POINT ( 'NONE',  ( 4.243569643749996345, -27.83227623338511947, -11.19563964674263978 ) ) ;
#6345=( BOUNDED_CURVE ( )  B_SPLINE_CURVE ( 2, ( #7756, #6373, #541, #4700, #1944, #14643, #6279, #7570, #16211 ),
 .UNSPECIFIED., .F., .T. ) 
 B_SPLINE_CURVE_WITH_KNOTS ( ( 3, 2, 2, 2, 3 ),
 ( 0.06034482758620690612, 0.06321839080459770721, 0.06896551724137930939, 0.07471264367816092544, 0.07758620689655172653 ),
 .UNSPECIFIED. ) 
 CURVE ( )  GEOMETRIC_REPRESENTATION_ITEM ( )  RATIONAL_B_SPLINE_CURVE ( ( 0.9330127018922194093, 0.9330127018922195203, 1.000000000000000000, 0.8660254037844387076, 1.000000000000000000, 0.8660254037844387076, 1.000000000000000000, 0.9330127018922194093, 0.9330127018922194093 ) ) 
 REPRESENTATION_ITEM ( '' )  );
#6348=CARTESIAN_POINT ( 'NONE',  ( 3.973088838427932590, -15.08697326462720056, -8.369503528065322939 ) ) ;
#6350=CARTESIAN_POINT ( 'NONE',  ( -4.243569643749997233, -22.94726928300758217, -12.76210693092232162 ) ) ;
#6351=DIRECTION ( 'NONE',  ( 0.000000000000000000, 0.000000000000000000, -1.000000000000000000 ) ) ;
#6352=CARTESIAN_POINT ( 'NONE',  ( -1.999999999999996225, -17.37920435354295989, -6.578072849473089789 ) ) ;
#6354=CARTESIAN_POINT ( 'NONE',  ( -4.243569643750005227, -25.33721873525807666, -7.632328254085517294 ) ) ;
#6360=VERTEX_POINT ( 'NONE', #18131 ) ;
#6362=ADVANCED_FACE ( 'NONE', ( #8174 ), #13931, .F. ) ;
#6363=DIRECTION ( 'NONE',  ( 0.000000000000000000, 0.8191520442889952403, -0.5735764363510413855 ) ) ;
#6367=CARTESIAN_POINT ( 'NONE',  ( -4.243569643749998122, -20.36617531942789938, -9.075922731621842487 ) ) ;
#6369=ORIENTED_EDGE ( 'NONE', *, *, #10366, .T. ) ;
#6373=CARTESIAN_POINT ( 'NONE',  ( 1.071796769724487675, -30.02068312334193934, -11.61871151373218503 ) ) ;
#6374=CARTESIAN_POINT ( 'NONE',  ( 6.428571428571432378, -14.26578344203647930, -2.827263138854382074 ) ) ;
#6375=CARTESIAN_POINT ( 'NONE',  ( -3.999999999999997335, -23.14312172474173224, -12.79664100063768650 ) ) ;
#6376=CARTESIAN_POINT ( 'NONE',  ( -4.243569643750000786, -20.02862550467770220, -4.322361524868783889 ) ) ;
#6378=VERTEX_POINT ( 'NONE', #4096 ) ;
#6380=CARTESIAN_POINT ( 'NONE',  ( 4.000000000000000888, -22.62585130588224658, -8.031584375918267682 ) ) ;
#6381=EDGE_CURVE ( 'NONE', #1052, #18219, #17124, .T. ) ;
#6382=VERTEX_POINT ( 'NONE', #5308 ) ;
#6383=VERTEX_POINT ( 'NONE', #10866 ) ;
#6391=ADVANCED_FACE ( 'NONE', ( #4189 ), #13835, .T. ) ;
#6393=CARTESIAN_POINT ( 'NONE',  ( 4.713407268011036227E-15, -18.71329538077844390, -10.49651124437128225 ) ) ;
#6397=CYLINDRICAL_SURFACE ( 'NONE', #12631, 2.000000000000001776 ) ;
#6398=CARTESIAN_POINT ( 'NONE',  ( -4.243569643749998122, -17.75281768130346194, -5.343661229830111381 ) ) ;
#6399=CARTESIAN_POINT ( 'NONE',  ( -2.121784821875005722, -26.86766402057294556, -7.682285581915135886 ) ) ;
#6400=CARTESIAN_POINT ( 'NONE',  ( -4.648177544792955347E-16, -29.83862777749724060, -11.35870953444733011 ) ) ;
#6402=AXIS2_PLACEMENT_3D ( 'NONE', #12770, #73, #2126 ) ;
#6403=CARTESIAN_POINT ( 'NONE',  ( -1.071796769724486786, -16.62756776554380878, -6.438934876394256435 ) ) ;
#6404=LINE ( 'NONE', #5190, #17598 ) ;
#6405=CARTESIAN_POINT ( 'NONE',  ( -4.433153569487539691, -10.00000000000000000, 28.39434458091831459 ) ) ;
#6406=CARTESIAN_POINT ( 'NONE',  ( 2.121784821875004390, -23.29887167946958115, -15.39999224841596437 ) ) ;
#6407=ORIENTED_EDGE ( 'NONE', *, *, #10920, .F. ) ;
#6410=CARTESIAN_POINT ( 'NONE',  ( 4.730628863548789710E-15, -17.33754842334290913, -9.022085378453862603 ) ) ;
#6413=CARTESIAN_POINT ( 'NONE',  ( 4.730628863548789710E-15, -21.75767183597313092, -15.33467581975593141 ) ) ;
#6414=CARTESIAN_POINT ( 'NONE',  ( -3.999999999999997335, -24.69177810288953978, -15.00835152021797114 ) ) ;
#6415=CARTESIAN_POINT ( 'NONE',  ( 4.243569643749996345, -23.73478956620236957, -5.343822230353133307 ) ) ;
#6416=VECTOR ( 'NONE', #17319, 1000.000000000000000 ) ;
#6420=CARTESIAN_POINT ( 'NONE',  ( 4.000000000000000888, -22.62585130588224658, -8.031584375918267682 ) ) ;
#6423=CARTESIAN_POINT ( 'NONE',  ( 4.898587196589413815E-16, 2.700915433685006750, 35.11257424290206330 ) ) ;
#6424=CARTESIAN_POINT ( 'NONE',  ( -5.577813053751546416E-15, -24.67643985033786791, -3.986341135846375838 ) ) ;
#6428=DIRECTION ( 'NONE',  ( 1.000000000000000000, 0.000000000000000000, 0.000000000000000000 ) ) ;
#6430=CARTESIAN_POINT ( 'NONE',  ( -4.243569643749997233, -22.91500560846283463, -12.71602962843106432 ) ) ;
#6434=CARTESIAN_POINT ( 'NONE',  ( -4.000000000000004441, -25.85116713280339340, -8.611494838171019239 ) ) ;
#6435=CARTESIAN_POINT ( 'NONE',  ( 2.121784821874994176, -28.37330216599443489, -9.832559698173744422 ) ) ;
#6436=VECTOR ( 'NONE', #10934, 1000.000000000000000 ) ;
#6441=CARTESIAN_POINT ( 'NONE',  ( 4.243569643749996345, -25.50929166616339572, -7.878073867372210159 ) ) ;
#6446=ADVANCED_FACE ( 'NONE', ( #16457 ), #14029, .T. ) ;
#6451=VECTOR ( 'NONE', #15266, 1000.000000000000000 ) ;
#6454=CARTESIAN_POINT ( 'NONE',  ( -2.121784821874996396, -19.64232189773168358, -10.17789796607362618 ) ) ;
#6458=CARTESIAN_POINT ( 'NONE',  ( -1.840775681772796268, -24.12649185032508825, -16.50800845489187196 ) ) ;
#6460=CARTESIAN_POINT ( 'NONE',  ( 9.666809584889323403, -9.963386536547416128, 0.1573640763989413160 ) ) ;
#6461=AXIS2_PLACEMENT_3D ( 'NONE', #3282, #4566, #1992 ) ;
#6463=CARTESIAN_POINT ( 'NONE',  ( -5.330712181944245322E-15, -23.97798589325759977, -1.419652468442682558 ) ) ;
#6466=CARTESIAN_POINT ( 'NONE',  ( -5.279047395330986450E-15, -26.99009867390753925, -6.211739741336077536 ) ) ;
#6476=CARTESIAN_POINT ( 'NONE',  ( -5.279047395330986450E-15, -24.34447736053341416, -2.433400936046320684 ) ) ;
#6478=EDGE_CURVE ( 'NONE', #8773, #12774, #6699, .T. ) ;
#6482=DIRECTION ( 'NONE',  ( 0.9454169814551710571, 0.000000000000000000, 0.3258630558627237384 ) ) ;
#6483=EDGE_CURVE ( 'NONE', #13448, #10757, #8927, .T. ) ;
#6484=CARTESIAN_POINT ( 'NONE',  ( -2.121784821874996396, -17.80329244868115168, -7.551491724072033840 ) ) ;
#6485=CARTESIAN_POINT ( 'NONE',  ( 4.243569643749996345, -25.79966473706612007, -8.292769589793513418 ) ) ;
#6487=ADVANCED_FACE ( 'NONE', ( #5498 ), #10972, .F. ) ;
#6489=CARTESIAN_POINT ( 'NONE',  ( 1.907117511807822519, -29.88501818502292906, -12.24335744624743860 ) ) ;
#6492=CARTESIAN_POINT ( 'NONE',  ( 7.191589934391298122, -10.00000000000000178, 14.52136967842653981 ) ) ;
#6493=DIRECTION ( 'NONE',  ( -0.000000000000000000, 1.000000000000000000, -0.000000000000000000 ) ) ;
#6494=CARTESIAN_POINT ( 'NONE',  ( 1.071796769724476128, -18.78002368763965890, -9.512960511135750252 ) ) ;
#6495=CARTESIAN_POINT ( 'NONE',  ( -4.243569643749997233, -24.75403505751336297, -15.34243587043265755 ) ) ;
#6498=ADVANCED_BREP_SHAPE_REPRESENTATION ( '', ( #13901, #16940 ), #12175 ) ;
#6499=CARTESIAN_POINT ( 'NONE',  ( 3.694449856179180092, -25.69578722143081251, -15.18691654432904947 ) ) ;
#6500=CARTESIAN_POINT ( 'NONE',  ( -4.243569643749997233, -18.26903647401939779, -6.080898069690205965 ) ) ;
#6503=CARTESIAN_POINT ( 'NONE',  ( 2.000000000000004441, -22.51988316363423337, -13.91972304540644245 ) ) ;
#6505=CIRCLE ( 'NONE', #11233, 2.000000000000001776 ) ;
#6506=CARTESIAN_POINT ( 'NONE',  ( 4.243569643750003451, -19.67788359580665869, -8.092940278475046156 ) ) ;
#6510=CARTESIAN_POINT ( 'NONE',  ( 0.000000000000000000, -15.45745613286697839, -10.86990606519494129 ) ) ;
#6513=ORIENTED_EDGE ( 'NONE', *, *, #2527, .T. ) ;
#6516=CARTESIAN_POINT ( 'NONE',  ( 2.000000000000004441, -18.71276956805914082, -8.482601352445005460 ) ) ;
#6517=CARTESIAN_POINT ( 'NONE',  ( 0.000000000000000000, 3.771166001944911361, 16.59141230903429687 ) ) ;
#6520=CARTESIAN_POINT ( 'NONE',  ( -2.121784821875005722, -27.35161913874413386, -8.373445119283974947 ) ) ;
#6523=CARTESIAN_POINT ( 'NONE',  ( 4.371749249414307315, -10.00000000000000178, -10.94697576041283682 ) ) ;
#6524=CARTESIAN_POINT ( 'NONE',  ( -5.330712181944245322E-15, -29.65639261313291541, -9.529257706903733194 ) ) ;
#6526=CIRCLE ( 'NONE', #12457, 4.000000000000000000 ) ;
#6531=CARTESIAN_POINT ( 'NONE',  ( -2.121784821875005722, -25.02863457152241722, -5.055879339913546211 ) ) ;
#6533=PLANE ( 'NONE',  #12716 ) ;
#6534=CARTESIAN_POINT ( 'NONE',  ( 3.999999999999996447, -27.12020499893503001, -10.42386873716718121 ) ) ;
#6538=CARTESIAN_POINT ( 'NONE',  ( -4.648177544792955347E-16, -29.83862777749724060, -11.35870953444733011 ) ) ;
#6542=CARTESIAN_POINT ( 'NONE',  ( -4.243569643750000786, -22.86782886461536179, -8.377164144099308984 ) ) ;
#6547=ADVANCED_FACE ( 'NONE', ( #1338 ), #8001, .F. ) ;
#6549=CARTESIAN_POINT ( 'NONE',  ( 1.261028757266463796, -23.92767164650701872, -16.69611796327299658 ) ) ;
#6551=CARTESIAN_POINT ( 'NONE',  ( 9.889275785751310721, -9.933886151507580919, 2.519662976721114944 ) ) ;
#6553=CARTESIAN_POINT ( 'NONE',  ( 3.579096709490575479E-14, -24.93454924669583406, -4.354959555776423130 ) ) ;
#6554=CARTESIAN_POINT ( 'NONE',  ( 2.121784821874994176, -22.95300484247709250, -2.091572879642740634 ) ) ;
#6557=CARTESIAN_POINT ( 'NONE',  ( -1.999999999999996225, -20.47651710983858564, -11.00149388863366440 ) ) ;
#6561=CARTESIAN_POINT ( 'NONE',  ( -1.999999999999996225, -18.34711458918039995, -7.960391923204007014 ) ) ;
#6563=CARTESIAN_POINT ( 'NONE',  ( 3.999999999999996447, -25.50702127099278371, -8.120003611597617521 ) ) ;
#6565=ORIENTED_EDGE ( 'NONE', *, *, #10558, .F. ) ;
#6568=CARTESIAN_POINT ( 'NONE',  ( -5.279047395330986450E-15, -24.08636796417544446, -2.064782516116274280 ) ) ;
#6570=CARTESIAN_POINT ( 'NONE',  ( -4.000000000000004441, -23.52818256558168031, -5.293929058800590504 ) ) ;
#6572=DIRECTION ( 'NONE',  ( 0.000000000000000000, 1.000000000000000000, 0.000000000000000000 ) ) ;
#6574=CARTESIAN_POINT ( 'NONE',  ( 2.121784821874994176, -23.43695996064828435, -2.782732417011581028 ) ) ;
#6576=CARTESIAN_POINT ( 'NONE',  ( 2.121784821875004390, -20.71777771588989125, -11.71380804911548701 ) ) ;
#6577=CARTESIAN_POINT ( 'NONE',  ( 0.1370520045797951059, -30.29850743920613709, -11.99201766838188554 ) ) ;
#6582=CARTESIAN_POINT ( 'NONE',  ( -1.071796769724477238, -25.91398618305211343, -5.753740464163247914 ) ) ;
#6583=CARTESIAN_POINT ( 'NONE',  ( 2.121784821874994176, -29.92195854414224598, -12.04427021775403084 ) ) ;
#6584=VERTEX_POINT ( 'NONE', #9482 ) ;
#6587=CARTESIAN_POINT ( 'NONE',  ( -2.121784821875005722, -23.47997819337460257, -2.844168820333258907 ) ) ;
#6592=AXIS2_PLACEMENT_3D ( 'NONE', #15407, #9812, #15493 ) ;
#6594=CARTESIAN_POINT ( 'NONE',  ( -2.000000000000005773, -28.06608030478504290, -9.761559716304219592 ) ) ;
#6596=CARTESIAN_POINT ( 'NONE',  ( 4.730628863548789710E-15, -16.33737451245578498, -7.593689001224928958 ) ) ;
#6599=CARTESIAN_POINT ( 'NONE',  ( -4.243569643750000786, -24.12611217186045565, -10.17417894125829037 ) ) ;
#6600=LINE ( 'NONE', #3461, #10563 ) ;
#6602=CARTESIAN_POINT ( 'NONE',  ( 2.000000000000004441, -18.45466017170117112, -8.113982932514955948 ) ) ;
#6604=CARTESIAN_POINT ( 'NONE',  ( 2.000000000000004441, -19.74520715349101607, -9.957075032165194628 ) ) ;
#6607=( BOUNDED_CURVE ( )  B_SPLINE_CURVE ( 2, ( #15913, #8656, #11817, #7364, #11629, #4680, #8569, #13120, #17323 ),
 .UNSPECIFIED., .F., .F. ) 
 B_SPLINE_CURVE_WITH_KNOTS ( ( 3, 2, 2, 2, 3 ),
 ( 0.6810344827586206629, 0.6839080459770114917, 0.6896551724137931494, 0.6954022988505746961, 0.6982758620689655249 ),
 .UNSPECIFIED. ) 
 CURVE ( )  GEOMETRIC_REPRESENTATION_ITEM ( )  RATIONAL_B_SPLINE_CURVE ( ( 0.9330127018922194093, 0.9330127018922194093, 1.000000000000000000, 0.8660254037844387076, 1.000000000000000000, 0.8660254037844387076, 1.000000000000000000, 0.9330127018922194093, 0.9330127018922194093 ) ) 
 REPRESENTATION_ITEM ( '' )  );
#6612=CARTESIAN_POINT ( 'NONE',  ( 6.618852602794225604, -14.16203062248956712, -2.127031534456948147 ) ) ;
#6616=CARTESIAN_POINT ( 'NONE',  ( -2.121784821874996396, -20.64249580861881128, -11.60629434330255982 ) ) ;
#6620=CARTESIAN_POINT ( 'NONE',  ( 4.898587196589409870E-16, 4.000000000000007105, -4.000000000000000000 ) ) ;
#6622=CARTESIAN_POINT ( 'NONE',  ( -4.243569643750005227, -26.66002939159267271, -9.521497656227012385 ) ) ;
#6627=CARTESIAN_POINT ( 'NONE',  ( 2.121784821875004390, -18.36252947412342351, -8.350164967253801862 ) ) ;
#6628=VERTEX_POINT ( 'NONE', #15522 ) ;
#6629=CARTESIAN_POINT ( 'NONE',  ( -14.99999999999999645, 10.00000000000000000, 30.00000000000000000 ) ) ;
#6632=CARTESIAN_POINT ( 'NONE',  ( 4.000000000000003553, -21.48691976548304439, -10.43133947375997472 ) ) ;
#6637=CARTESIAN_POINT ( 'NONE',  ( 4.243569643750003451, -19.16166480309071218, -7.355703438614951573 ) ) ;
#6641=CARTESIAN_POINT ( 'NONE',  ( 4.730628863548789710E-15, -22.75784574686024797, -16.76307219698486506 ) ) ;
#6642=CARTESIAN_POINT ( 'NONE',  ( 3.046716722576175318, -24.86286735169470319, -16.06997776478271334 ) ) ;
#6643=CARTESIAN_POINT ( 'NONE',  ( 7.502920075503393349, -12.79035154381909756, 6.457010517113837444 ) ) ;
#6644=CARTESIAN_POINT ( 'NONE',  ( -5.330712181944245322E-15, -30.65656652402004312, -10.95765408413266861 ) ) ;
#6647=CARTESIAN_POINT ( 'NONE',  ( 3.999999999999996447, -23.76478284628143811, -5.631829278076560641 ) ) ;
#6651=CARTESIAN_POINT ( 'NONE',  ( -4.000000000000000888, -21.14172227611897270, -5.912028460313731415 ) ) ;
#6652=EDGE_CURVE ( 'NONE', #1834, #14266, #15816, .T. ) ;
#6655=CARTESIAN_POINT ( 'NONE',  ( 1.533898589781675205E-14, -26.93489706776514581, -7.211752309227528634 ) ) ;
#6657=EDGE_CURVE ( 'NONE', #13482, #12581, #12608, .T. ) ;
#6660=CARTESIAN_POINT ( 'NONE',  ( 1.999999999999994449, -23.89331173033122369, -3.802228594101777492 ) ) ;
#6662=CARTESIAN_POINT ( 'NONE',  ( -4.000000000000000888, -21.65794106883490855, -6.649265300173826887 ) ) ;
#6664=CARTESIAN_POINT ( 'NONE',  ( -14.99999999999999645, -10.00000000000000000, -30.00000000000000000 ) ) ;
#6665=CARTESIAN_POINT ( 'NONE',  ( -4.243569643750004339, -22.75612477167839387, -3.946144054785039934 ) ) ;
#6666=CARTESIAN_POINT ( 'NONE',  ( 4.243569643750003451, -20.19410238852258743, -8.830177118335141628 ) ) ;
#6669=CARTESIAN_POINT ( 'NONE',  ( 1.999999999999994449, -27.31326123277925433, -8.686422659181676664 ) ) ;
#6675=ADVANCED_FACE ( 'NONE', ( #12811 ), #11236, .F. ) ;
#6676=CARTESIAN_POINT ( 'NONE',  ( -5.330712181944245322E-15, -24.72005040778675777, -2.479430425741570243 ) ) ;
#6679=CARTESIAN_POINT ( 'NONE',  ( -1.999999999999996225, -22.21875553454993124, -13.48966822215472305 ) ) ;
#6681=CARTESIAN_POINT ( 'NONE',  ( 4.730628863548789710E-15, -16.07926511609781528, -7.225070581294880334 ) ) ;
#6683=AXIS2_PLACEMENT_3D ( 'NONE', #18221, #11051, #11226 ) ;
#6684=CARTESIAN_POINT ( 'NONE',  ( -4.243569643749998122, -22.91500560846283463, -12.71602962843106432 ) ) ;
#6685=CARTESIAN_POINT ( 'NONE',  ( -6.158835246850665095E-15, -22.83371997885389604, -15.30223878937131587 ) ) ;
#6691=CARTESIAN_POINT ( 'NONE',  ( 4.000000000000003553, -19.68015399097727069, -7.851010534249639683 ) ) ;
#6692=CARTESIAN_POINT ( 'NONE',  ( 1.071796769724495224, -22.58713728321475855, -14.95008220409718369 ) ) ;
#6695=CARTESIAN_POINT ( 'NONE',  ( -4.243569643750000786, -24.12611217186045565, -10.17417894125829037 ) ) ;
#6699=LINE ( 'NONE', #5223, #13495 ) ;
#6700=CARTESIAN_POINT ( 'NONE',  ( -2.121784821874996396, -20.93286887952152497, -12.02099006572386486 ) ) ;
#6702=EDGE_CURVE ( 'NONE', #12103, #2069, #4370, .T. ) ;
#6703=( BOUNDED_CURVE ( )  B_SPLINE_CURVE ( 2, ( #14692, #17936, #13642, #9740, #5393, #5483, #14010, #15051, #10861 ),
 .UNSPECIFIED., .F., .F. ) 
 B_SPLINE_CURVE_WITH_KNOTS ( ( 3, 2, 2, 2, 3 ),
 ( 0.3706896551724138122, 0.3735632183908045856, 0.3793103448275861878, 0.3850574712643677899, 0.3879310344827586188 ),
 .UNSPECIFIED. ) 
 CURVE ( )  GEOMETRIC_REPRESENTATION_ITEM ( )  RATIONAL_B_SPLINE_CURVE ( ( 0.9330127018922194093, 0.9330127018922200755, 1.000000000000000000, 0.8660254037844387076, 1.000000000000000000, 0.8660254037844387076, 1.000000000000000000, 0.9330127018922194093, 0.9330127018922194093 ) ) 
 REPRESENTATION_ITEM ( '' )  );
#6710=CARTESIAN_POINT ( 'NONE',  ( 4.243569643749996345, -24.47685408073152402, -6.403600187652020992 ) ) ;
#6711=CARTESIAN_POINT ( 'NONE',  ( 1.071796769724494780, -28.02033530227262048, -8.761918760281082186 ) ) ;
#6717=CARTESIAN_POINT ( 'NONE',  ( -2.000000000000005773, -29.42115463636932304, -11.69680642194373554 ) ) ;
#6720=EDGE_LOOP ( 'NONE', ( #1304, #11478, #13465 ) ) ;
#6721=CARTESIAN_POINT ( 'NONE',  ( 2.121784821874994176, -23.72733303155099804, -3.197428139432884286 ) ) ;
#6726=CARTESIAN_POINT ( 'NONE',  ( -6.428571428571423496, -11.73421655796351892, 14.25837509840161310 ) ) ;
#6728=CARTESIAN_POINT ( 'NONE',  ( -3.877086799165925690, -27.97239129529922508, -13.72246263182690917 ) ) ;
#6729=CARTESIAN_POINT ( 'NONE',  ( 1.999999999999994449, -29.31360905384856608, -11.54321541263277950 ) ) ;
#6731=CARTESIAN_POINT ( 'NONE',  ( 2.121784821874994176, -28.85725728416562674, -10.52371923554258260 ) ) ;
#6733=CARTESIAN_POINT ( 'NONE',  ( -4.000000000000000888, -23.46470684334068935, -9.229594239684162815 ) ) ;
#6734=CARTESIAN_POINT ( 'NONE',  ( -4.000000000000000888, -21.20624962591340790, -6.004183066303009575 ) ) ;
#6737=CONICAL_SURFACE ( 'NONE', #1722, 2.000000000000001776, 1.029744260000000189 ) ;
#6742=CARTESIAN_POINT ( 'NONE',  ( -3.999999999999997335, -18.49715259029829539, -6.161509441896827255 ) ) ;
#6745=CARTESIAN_POINT ( 'NONE',  ( 2.121784821874994176, -28.11519276963646519, -9.463941278243694910 ) ) ;
#6747=CARTESIAN_POINT ( 'NONE',  ( -3.999999999999997335, -19.27148077937220449, -7.267364701686970463 ) ) ;
#6753=CARTESIAN_POINT ( 'NONE',  ( 4.243569643750000786, -22.48066477007841613, -7.824236514204232940 ) ) ;
#6754=LINE ( 'NONE', #5373, #6436 ) ;
#6756=CARTESIAN_POINT ( 'NONE',  ( -3.999999999999997335, -22.17521148910429574, -11.41432192690677283 ) ) ;
#6758=CARTESIAN_POINT ( 'NONE',  ( -14.99999999999999645, -10.00000000000000000, 30.00000000000000000 ) ) ;
#6759=ORIENTED_EDGE ( 'NONE', *, *, #2858, .T. ) ;
#6764=CARTESIAN_POINT ( 'NONE',  ( 3.250767337421092140, -21.87258502241503066, -2.200193550433863887 ) ) ;
#6767=CARTESIAN_POINT ( 'NONE',  ( -4.000000000000000888, -24.75525382513053430, -11.07268633933439972 ) ) ;
#6769=ADVANCED_FACE ( 'NONE', ( #1794 ), #10001, .T. ) ;
#6770=CARTESIAN_POINT ( 'NONE',  ( -4.243569643750000786, -20.54484429739364515, -5.059598364728879361 ) ) ;
#6773=VECTOR ( 'NONE', #6843, 1000.000000000000000 ) ;
#6774=CARTESIAN_POINT ( 'NONE',  ( 2.121784821874994176, -26.79238211330187625, -7.574771876102201595 ) ) ;
#6775=EDGE_CURVE ( 'NONE', #16719, #8888, #13921, .T. ) ;
#6781=ORIENTED_EDGE ( 'NONE', *, *, #17289, .F. ) ;
#6786=CARTESIAN_POINT ( 'NONE',  ( 4.000000000000003553, -20.97070097276711209, -9.694102633899875698 ) ) ;
#6787=VERTEX_POINT ( 'NONE', #8344 ) ;
#6789=VECTOR ( 'NONE', #16843, 1000.000000000000000 ) ;
#6790=CARTESIAN_POINT ( 'NONE',  ( 4.243569643750003451, -22.22671388484159039, -11.73304717528426977 ) ) ;
#6798=CARTESIAN_POINT ( 'NONE',  ( 4.730628863548789710E-15, -20.46712485418328242, -13.49158372010569273 ) ) ;
#6799=EDGE_CURVE ( 'NONE', #4066, #8485, #11905, .T. ) ;
#6802=CYLINDRICAL_SURFACE ( 'NONE', #18084, 4.000000000000000000 ) ;
#6804=CARTESIAN_POINT ( 'NONE',  ( 4.243569643750000786, -22.19029169917569888, -7.409540791782929681 ) ) ;
#6805=DIRECTION ( 'NONE',  ( 0.000000000000000000, 0.8191520442889952403, -0.5735764363510413855 ) ) ;
#6806=DIRECTION ( 'NONE',  ( -6.162975822039154730E-33, 0.5735764363510414965, 0.8191520442889950182 ) ) ;
#6815=CARTESIAN_POINT ( 'NONE',  ( -4.243569643750004339, -23.04649784258110756, -4.360839777206344081 ) ) ;
#6817=( BOUNDED_CURVE ( )  B_SPLINE_CURVE ( 2, ( #3777, #2407, #9518, #13883, #12395, #13604, #15104, #2678, #8039 ),
 .UNSPECIFIED., .F., .T. ) 
 B_SPLINE_CURVE_WITH_KNOTS ( ( 3, 2, 2, 2, 3 ),
 ( 0.6120689655172414367, 0.6149425287356321546, 0.6206896551724138122, 0.6264367816091953589, 0.6293103448275861878 ),
 .UNSPECIFIED. ) 
 CURVE ( )  GEOMETRIC_REPRESENTATION_ITEM ( )  RATIONAL_B_SPLINE_CURVE ( ( 0.9330127018922194093, 0.9330127018922206306, 1.000000000000000000, 0.8660254037844387076, 1.000000000000000000, 0.8660254037844387076, 1.000000000000000000, 0.9330127018922194093, 0.9330127018922194093 ) ) 
 REPRESENTATION_ITEM ( '' )  );
#6818=DIRECTION ( 'NONE',  ( -0.000000000000000000, -0.5735764363510414965, -0.8191520442889950182 ) ) ;
#6819=CARTESIAN_POINT ( 'NONE',  ( 4.243569643750003451, -24.80780784842128028, -15.41923137458474535 ) ) ;
#6821=CARTESIAN_POINT ( 'NONE',  ( 4.898587196589413815E-16, 2.700915433685006750, 35.11257424290206330 ) ) ;
#6823=CARTESIAN_POINT ( 'NONE',  ( -2.121784821875005722, -29.67460370596585406, -11.69101089865440457 ) ) ;
#6824=ORIENTED_EDGE ( 'NONE', *, *, #15188, .F. ) ;
#6826=CARTESIAN_POINT ( 'NONE',  ( 4.000000000000003553, -19.93826338733523684, -8.219628954179688307 ) ) ;
#6829=ORIENTED_EDGE ( 'NONE', *, *, #337, .F. ) ;
#6830=CARTESIAN_POINT ( 'NONE',  ( -6.158835246850665095E-15, -22.12391913957442213, -14.28853813557044639 ) ) ;
#6831=EDGE_CURVE ( 'NONE', #13588, #17004, #9821, .T. ) ;
#6833=CARTESIAN_POINT ( 'NONE',  ( -1.071796769724486786, -17.14378655825974818, -7.176171716254351018 ) ) ;
#6837=CARTESIAN_POINT ( 'NONE',  ( 2.121784821874994176, -28.63141156235240459, -10.20117811810379216 ) ) ;
#6839=CARTESIAN_POINT ( 'NONE',  ( -5.279047395330986450E-15, -25.11880554960731970, -3.539256195836466112 ) ) ;
#6840=ORIENTED_EDGE ( 'NONE', *, *, #18289, .F. ) ;
#6842=CARTESIAN_POINT ( 'NONE',  ( 0.000000000000000000, -13.00000000000000178, -12.59063537424807677 ) ) ;
#6843=DIRECTION ( 'NONE',  ( 0.000000000000000000, -0.5735764363510413855, -0.8191520442889951292 ) ) ;
#6846=CARTESIAN_POINT ( 'NONE',  ( -2.121784821874996396, -19.38421250137371388, -9.809279546143578443 ) ) ;
#6850=CARTESIAN_POINT ( 'NONE',  ( -1.999999999999996225, -21.25084529891249119, -12.10734914842380761 ) ) ;
#6853=CARTESIAN_POINT ( 'NONE',  ( -1.071796769724486786, -22.56408388177708702, -14.91715853478535436 ) ) ;
#6857=CARTESIAN_POINT ( 'NONE',  ( 2.121784821875004390, -16.81387309597561242, -6.138454447673516334 ) ) ;
#6860=CARTESIAN_POINT ( 'NONE',  ( -4.000000000000004441, -26.10927652916136310, -8.980113258101068752 ) ) ;
#6861=EDGE_LOOP ( 'NONE', ( #11132, #387, #9553, #17347 ) ) ;
#6863=CARTESIAN_POINT ( 'NONE',  ( -4.243569643750000786, -20.28673490103567545, -4.690979944798832513 ) ) ;
#6865=CARTESIAN_POINT ( 'NONE',  ( -1.999999999999996225, -21.50895469527046444, -12.47596756835385534 ) ) ;
#6866=CARTESIAN_POINT ( 'NONE',  ( 2.121784821874994176, -25.75994452787000100, -6.100298196382009763 ) ) ;
#6867=CARTESIAN_POINT ( 'NONE',  ( 3.999999999999995559, 2.343145750507625191, -2.343145750507618086 ) ) ;
#6869=ORIENTED_EDGE ( 'NONE', *, *, #12152, .F. ) ;
#6870=ORIENTED_EDGE ( 'NONE', *, *, #14627, .T. ) ;
#6874=CARTESIAN_POINT ( 'NONE',  ( -2.465190328815646976E-33, -26.97786251599082519, -14.24690051095425858 ) ) ;
#6878=CARTESIAN_POINT ( 'NONE',  ( 4.243569643750000786, -24.77138566275538523, -11.09572499108340793 ) ) ;
#6882=EDGE_CURVE ( 'NONE', #18179, #16392, #1774, .T. ) ;
#6884=CARTESIAN_POINT ( 'NONE',  ( 4.243569643750000786, -23.51310235551028782, -9.298710193924424772 ) ) ;
#6886=AXIS2_PLACEMENT_3D ( 'NONE', #11562, #4713, #5916 ) ;
#6887=CARTESIAN_POINT ( 'NONE',  ( -1.281796014810987483, -15.42359483004433507, -10.64137488400932696 ) ) ;
#6891=CARTESIAN_POINT ( 'NONE',  ( -4.243569643750000786, -22.57745579371264455, -7.962468421678005726 ) ) ;
#6894=CARTESIAN_POINT ( 'NONE',  ( 0.000000000000000000, 5.977523610840987267, 32.81826849749789687 ) ) ;
#6903=CARTESIAN_POINT ( 'NONE',  ( 4.243569643750000786, -21.44822718464654088, -6.349762834484042884 ) ) ;
#6906=CARTESIAN_POINT ( 'NONE',  ( -8.500000000000005329, 0.000000000000000000, 18.49999999999999645 ) ) ;
#6910=LINE ( 'NONE', #18346, #9392 ) ;
#6911=CARTESIAN_POINT ( 'NONE',  ( -2.121784821874996396, -22.44926158312459208, -14.18662328281289398 ) ) ;
#6913=CARTESIAN_POINT ( 'NONE',  ( -1.071796769724477238, -26.68831437212602609, -6.859595723953392010 ) ) ;
#6914=CARTESIAN_POINT ( 'NONE',  ( 4.000000000000000888, -22.36774190952427688, -7.662965955988220834 ) ) ;
#6918=CARTESIAN_POINT ( 'NONE',  ( 1.071796769724485232, -28.79466349134653669, -9.867774020071223617 ) ) ;
#6920=DIRECTION ( 'NONE',  ( 0.000000000000000000, 0.000000000000000000, 1.000000000000000000 ) ) ;
#6922=( BOUNDED_CURVE ( )  B_SPLINE_CURVE ( 2, ( #5053, #3941, #5425, #17968, #9677, #4030, #13862, #15359, #16385 ),
 .UNSPECIFIED., .F., .T. ) 
 B_SPLINE_CURVE_WITH_KNOTS ( ( 3, 2, 2, 2, 3 ),
 ( 0.2500000000000000000, 0.2528735632183908288, 0.2586206896551724310, 0.2643678160919540332, 0.2672413793103448620 ),
 .UNSPECIFIED. ) 
 CURVE ( )  GEOMETRIC_REPRESENTATION_ITEM ( )  RATIONAL_B_SPLINE_CURVE ( ( 0.9330127018922194093, 0.9330127018922190762, 1.000000000000000000, 0.8660254037844387076, 1.000000000000000000, 0.8660254037844387076, 1.000000000000000000, 0.9330127018922187432, 0.9330127018922194093 ) ) 
 REPRESENTATION_ITEM ( '' )  );
#6923=ORIENTED_EDGE ( 'NONE', *, *, #17154, .F. ) ;
#6924=CARTESIAN_POINT ( 'NONE',  ( 2.121784821874994176, -29.14763035506834044, -10.93841495796388763 ) ) ;
#6926=ORIENTED_EDGE ( 'NONE', *, *, #14043, .F. ) ;
#6928=EDGE_CURVE ( 'NONE', #16586, #1458, #15702, .T. ) ;
#6929=CARTESIAN_POINT ( 'NONE',  ( -5.577813053751546416E-15, -26.16056887869124381, -6.105897049437384538 ) ) ;
#6930=DIRECTION ( 'NONE',  ( 0.000000000000000000, 0.000000000000000000, 1.000000000000000000 ) ) ;
#6931=ADVANCED_FACE ( 'NONE', ( #1405 ), #15764, .F. ) ;
#6932=CARTESIAN_POINT ( 'NONE',  ( -5.330712181944245322E-15, -26.30097046047931997, -4.737218247813111738 ) ) ;
#6937=CARTESIAN_POINT ( 'NONE',  ( 4.713407268011036227E-15, -21.10080729779459574, -13.90623162973098559 ) ) ;
#6938=DIRECTION ( 'NONE',  ( 0.000000000000000000, 0.8191520442889952403, -0.5735764363510413855 ) ) ;
#6941=EDGE_CURVE ( 'NONE', #5271, #16039, #4178, .T. ) ;
#6944=CARTESIAN_POINT ( 'NONE',  ( 2.000000000000004441, -23.87495749521851351, -15.85496975104595840 ) ) ;
#6948=CARTESIAN_POINT ( 'NONE',  ( 1.999999999999994449, -26.99062448662684943, -8.225649633262349880 ) ) ;
#6949=ORIENTED_EDGE ( 'NONE', *, *, #14842, .T. ) ;
#6950=CARTESIAN_POINT ( 'NONE',  ( 4.243569643749996345, -22.18613318805455847, -3.132111710772846891 ) ) ;
#6952=CARTESIAN_POINT ( 'NONE',  ( -5.577813053751546416E-15, -23.12778347219005681, -1.774630616266089866 ) ) ;
#6954=CARTESIAN_POINT ( 'NONE',  ( 4.243569643749997233, -24.21874468437355432, -6.034981767721972368 ) ) ;
#6957=ORIENTED_EDGE ( 'NONE', *, *, #11270, .F. ) ;
#6958=ORIENTED_EDGE ( 'NONE', *, *, #2424, .F. ) ;
#6960=CARTESIAN_POINT ( 'NONE',  ( -1.999999999999996225, -19.12144277825430549, -9.066247182994150222 ) ) ;
#6962=CARTESIAN_POINT ( 'NONE',  ( -4.000000000000000888, -21.46435902227137760, -6.372801486233056423 ) ) ;
#6964=ORIENTED_EDGE ( 'NONE', *, *, #15676, .T. ) ;
#6966=CARTESIAN_POINT ( 'NONE',  ( 4.243569643750000786, -22.44840109553366858, -7.778159211712977417 ) ) ;
#6969=CARTESIAN_POINT ( 'NONE',  ( 0.000000000000000000, -10.00000000000000178, -12.59063537424807677 ) ) ;
#6970=CARTESIAN_POINT ( 'NONE',  ( 0.000000000000000000, 5.977523610840987267, 32.81826849749789687 ) ) ;
#6971=CARTESIAN_POINT ( 'NONE',  ( -4.243569643750000786, -24.41648524276317289, -10.58887466367959540 ) ) ;
#6974=CARTESIAN_POINT ( 'NONE',  ( -4.243569643750000786, -21.02879941556483345, -5.750757902097718421 ) ) ;
#6980=AXIS2_PLACEMENT_3D ( 'NONE', #10447, #16125, #3415 ) ;
#6981=CARTESIAN_POINT ( 'NONE',  ( -2.121784821875005722, -29.41649430960788081, -11.32239247872435506 ) ) ;
#6983=CARTESIAN_POINT ( 'NONE',  ( -9.891620614305184134, -9.933529378329316373, 2.554464806243397224 ) ) ;
#6985=CARTESIAN_POINT ( 'NONE',  ( -5.330712181944246111E-15, -25.26853287504744472, -3.262744568092922570 ) ) ;
#6989=DIRECTION ( 'NONE',  ( -0.000000000000000000, -0.5735764363510414965, -0.8191520442889950182 ) ) ;
#6991=CARTESIAN_POINT ( 'NONE',  ( 1.071796769724487675, -29.76257372698396964, -11.25009309380213551 ) ) ;
#6994=CARTESIAN_POINT ( 'NONE',  ( 4.243569643750003451, -24.03347965934736763, -14.31337611479460037 ) ) ;
#6997=CARTESIAN_POINT ( 'NONE',  ( -1.999999999999996225, -19.44407952440671039, -9.527020208913473454 ) ) ;
#7000=FACE_OUTER_BOUND ( 'NONE', #12210, .T. ) ;
#7006=CARTESIAN_POINT ( 'NONE',  ( -5.330712181944246111E-15, -29.91450200949087801, -9.897876126833780930 ) ) ;
#7009=CARTESIAN_POINT ( 'NONE',  ( 1.533898589781675205E-14, -27.25753381391755426, -7.672525335146852754 ) ) ;
#7010=CARTESIAN_POINT ( 'NONE',  ( 1.071796769724504328, -24.60038579982458984, -3.877724695201188787 ) ) ;
#7014=CARTESIAN_POINT ( 'NONE',  ( -2.121784821875005722, -26.35144522785700616, -6.945048742055040414 ) ) ;
#7015=ORIENTED_EDGE ( 'NONE', *, *, #4382, .F. ) ;
#7018=CARTESIAN_POINT ( 'NONE',  ( -2.000000000000005773, -27.09817006914760640, -8.379240642573305919 ) ) ;
#7019=( BOUNDED_CURVE ( )  B_SPLINE_CURVE ( 3, ( #9339, #9429, #15379, #10823 ),
 .UNSPECIFIED., .F., .T. ) 
 B_SPLINE_CURVE_WITH_KNOTS ( ( 4, 4 ),
 ( 4.712388980384689674, 6.283185307179586232 ),
 .UNSPECIFIED. ) 
 CURVE ( )  GEOMETRIC_REPRESENTATION_ITEM ( )  RATIONAL_B_SPLINE_CURVE ( ( 1.000000000000000000, 0.8047378541243649375, 0.8047378541243649375, 1.000000000000000000 ) ) 
 REPRESENTATION_ITEM ( '' )  );
#7026=CARTESIAN_POINT ( 'NONE',  ( -1.999999999999996225, -23.57382986613421139, -15.42491492779423723 ) ) ;
#7033=CARTESIAN_POINT ( 'NONE',  ( -2.000000000000005773, -26.25931453027926210, -7.181230776793885440 ) ) ;
#7038=CARTESIAN_POINT ( 'NONE',  ( 4.243569643749997233, -25.25118226980542957, -7.509455447442163312 ) ) ;
#7040=CARTESIAN_POINT ( 'NONE',  ( -2.000000000000005773, -22.71031033106213570, -2.112727503762495296 ) ) ;
#7042=CARTESIAN_POINT ( 'NONE',  ( 2.000000000000004441, -19.42257040733860762, -9.496302006245869620 ) ) ;
#7049=CARTESIAN_POINT ( 'NONE',  ( -1.071796769724496334, -24.68796655105670013, -4.002802970502292723 ) ) ;
#7051=ORIENTED_EDGE ( 'NONE', *, *, #18132, .T. ) ;
#7053=CARTESIAN_POINT ( 'NONE',  ( 2.121784821874994176, -25.50183513151203130, -5.731679776451962915 ) ) ;
#7056=ADVANCED_FACE ( 'NONE', ( #1492 ), #7127, .F. ) ;
#7059=CARTESIAN_POINT ( 'NONE',  ( 4.243569643750000786, -22.73877416643638227, -8.192854934134281564 ) ) ;
#7065=CARTESIAN_POINT ( 'NONE',  ( -2.121784821874996396, -17.54518305232318554, -7.182873304141986992 ) ) ;
#7067=DIRECTION ( 'NONE',  ( 0.000000000000000000, -0.5735764363510414965, -0.8191520442889950182 ) ) ;
#7071=CARTESIAN_POINT ( 'NONE',  ( -4.243569643749997233, -24.72177138296861898, -15.29635856794139848 ) ) ;
#7075=CARTESIAN_POINT ( 'NONE',  ( 8.500000000000019540, 10.00000000000000000, -22.49999999999999289 ) ) ;
#7077=CARTESIAN_POINT ( 'NONE',  ( -5.330712181944246111E-15, -24.49420468597354272, -2.156889308302777586 ) ) ;
#7079=VECTOR ( 'NONE', #1613, 999.9999999999998863 ) ;
#7083=CARTESIAN_POINT ( 'NONE',  ( -2.121784821875005722, -28.90027551689194496, -10.58515563886426136 ) ) ;
#7085=CARTESIAN_POINT ( 'NONE',  ( -1.071796769724496334, -25.65587678669413663, -5.385122044233206395 ) ) ;
#7087=CARTESIAN_POINT ( 'NONE',  ( -2.121784821875005722, -28.38405672417600911, -9.847918799004165891 ) ) ;
#7090=CARTESIAN_POINT ( 'NONE',  ( 4.713407268011036227E-15, -15.93861937063522483, -6.533863231130032645 ) ) ;
#7100=ORIENTED_EDGE ( 'NONE', *, *, #2083, .T. ) ;
#7101=CARTESIAN_POINT ( 'NONE',  ( -4.243569643750000786, -23.90026645004723704, -9.851637823819498152 ) ) ;
#7108=CARTESIAN_POINT ( 'NONE',  ( 2.000000000000004441, -19.16446101098063792, -9.127683586315821884 ) ) ;
#7111=CARTESIAN_POINT ( 'NONE',  ( 4.000000000000000888, -26.17485550509936942, -13.10008764894965871 ) ) ;
#7112=CARTESIAN_POINT ( 'NONE',  ( -4.243569643750005227, -23.56271663529704696, -5.098076617066438665 ) ) ;
#7117=FACE_OUTER_BOUND ( 'NONE', #12464, .T. ) ;
#7120=CARTESIAN_POINT ( 'NONE',  ( -3.999999999999997335, -24.75630545268398208, -15.10050612620725197 ) ) ;
#7124=CARTESIAN_POINT ( 'NONE',  ( -4.000000000000004441, -25.07683894372948785, -7.505639578380876031 ) ) ;
#7127=CYLINDRICAL_SURFACE ( 'NONE', #3814, 4.000000000000000000 ) ;
#7129=CARTESIAN_POINT ( 'NONE',  ( 9.609723682702158598, -9.971172948454899654, 12.03203570040726511 ) ) ;
#7130=CARTESIAN_POINT ( 'NONE',  ( -2.121784821874996396, -19.61005822318693248, -10.13182066358236888 ) ) ;
#7135=ORIENTED_EDGE ( 'NONE', *, *, #15672, .F. ) ;
#7137=EDGE_CURVE ( 'NONE', #16218, #10036, #12106, .T. ) ;
#7138=CARTESIAN_POINT ( 'NONE',  ( -7.191589934391292793, -10.00000000000000178, 14.52136967842657000 ) ) ;
#7140=CARTESIAN_POINT ( 'NONE',  ( -1.071796769724486564, -27.72075195755788712, -8.334069403673582954 ) ) ;
#7142=ORIENTED_EDGE ( 'NONE', *, *, #5297, .F. ) ;
#7144=CARTESIAN_POINT ( 'NONE',  ( -2.121784821874996396, -19.35194882682896633, -9.763202243652322920 ) ) ;
#7148=CARTESIAN_POINT ( 'NONE',  ( 2.000000000000004441, -22.06819172071273272, -13.27464081153562425 ) ) ;
#7149=CARTESIAN_POINT ( 'NONE',  ( -5.330712181944245322E-15, -27.33340804591119522, -6.211691927533303570 ) ) ;
#7151=CARTESIAN_POINT ( 'NONE',  ( -3.122678035296125643, -15.23680830283799281, -9.380745725236772969 ) ) ;
#7154=DIRECTION ( 'NONE',  ( -0.000000000000000000, -0.5735764363510414965, -0.8191520442889950182 ) ) ;
#7158=CARTESIAN_POINT ( 'NONE',  ( 4.243569643750000786, -20.64163532102788778, -5.197830272202643265 ) ) ;
#7159=CARTESIAN_POINT ( 'NONE',  ( -8.999999999999996447, -10.00000000000000000, 30.00000000000000000 ) ) ;
#7164=CARTESIAN_POINT ( 'NONE',  ( 4.243569643750000786, -27.09437022997710187, -14.41329077045383578 ) ) ;
#7166=CARTESIAN_POINT ( 'NONE',  ( -9.356479678992938531, -9.999999999999996447, 13.59332006026303574 ) ) ;
#7169=AXIS2_PLACEMENT_3D ( 'NONE', #15945, #84, #5737 ) ;
#7170=CARTESIAN_POINT ( 'NONE',  ( -4.243569643750004339, -22.27216965350720557, -3.254984517416200873 ) ) ;
#7172=VECTOR ( 'NONE', #7388, 1000.000000000000000 ) ;
#7173=CARTESIAN_POINT ( 'NONE',  ( -1.999999999999996225, -17.05656760739055500, -6.117299823553768334 ) ) ;
#7175=CARTESIAN_POINT ( 'NONE',  ( 2.121784821874994176, -28.08292909509171764, -9.417863975752439387 ) ) ;
#7177=CARTESIAN_POINT ( 'NONE',  ( -4.000000000000004441, -26.43191327531376800, -9.440886284020393759 ) ) ;
#7179=CARTESIAN_POINT ( 'NONE',  ( -5.330712181944245322E-15, -28.07547256044035322, -7.271469884832189479 ) ) ;
#7181=CARTESIAN_POINT ( 'NONE',  ( 2.694913683823408235, -15.45745613286698550, -10.86990606519495195 ) ) ;
#7183=CARTESIAN_POINT ( 'NONE',  ( -2.000000000000005773, -23.48463852013604480, -3.218582763552638948 ) ) ;
#7186=ORIENTED_EDGE ( 'NONE', *, *, #1434, .F. ) ;
#7193=CARTESIAN_POINT ( 'NONE',  ( -4.243569643749998122, -21.65672230121773723, -10.91901483127208294 ) ) ;
#7195=VERTEX_POINT ( 'NONE', #14665 ) ;
#7197=CARTESIAN_POINT ( 'NONE',  ( -6.938893903907228378E-15, 6.938893903907228378E-15, 30.00000000000000000 ) ) ;
#7198=CARTESIAN_POINT ( 'NONE',  ( -1.071796769724477238, -25.72040413648858603, -5.477276650222477450 ) ) ;
#7200=CARTESIAN_POINT ( 'NONE',  ( -2.000000000000005773, -28.64682644729541749, -10.59095116215359234 ) ) ;
#7201=CARTESIAN_POINT ( 'NONE',  ( 1.071796769724485232, -29.50446433062600349, -10.88147467387208955 ) ) ;
#7202=CARTESIAN_POINT ( 'NONE',  ( -5.330712181944245322E-15, -26.04286106412135027, -4.368599827883064890 ) ) ;
#7206=ORIENTED_EDGE ( 'NONE', *, *, #7600, .T. ) ;
#7208=CYLINDRICAL_SURFACE ( 'NONE', #74, 4.000000000000000000 ) ;
#7217=CARTESIAN_POINT ( 'NONE',  ( 1.999999999999994449, -26.21629629755294033, -7.119794373472207560 ) ) ;
#7221=CARTESIAN_POINT ( 'NONE',  ( -4.551717183842042047, -10.00000000000000000, -2.180355508048917201 ) ) ;
#7222=CARTESIAN_POINT ( 'NONE',  ( -4.243569643749998122, -20.59202104124112154, -9.398463849060636477 ) ) ;
#7229=CARTESIAN_POINT ( 'NONE',  ( -3.999999999999997335, -19.59411752552461294, -7.728137727606295471 ) ) ;
#7234=CARTESIAN_POINT ( 'NONE',  ( 4.243569643749996345, -24.73496347708949017, -6.772218607582066952 ) ) ;
#7240=CARTESIAN_POINT ( 'NONE',  ( 4.243569643750003451, -20.71032118123852683, -9.567413958195238877 ) ) ;
#7241=CARTESIAN_POINT ( 'NONE',  ( 0.000000000000000000, 4.000000000000007105, 4.000000000000000000 ) ) ;
#7242=CARTESIAN_POINT ( 'NONE',  ( -3.108848142585320939, -10.00000000000000178, -11.78746955954697739 ) ) ;
#7243=DIRECTION ( 'NONE',  ( 0.8191520442889951292, 0.4698463103929521600, -0.3289899283371603422 ) ) ;
#7245=CARTESIAN_POINT ( 'NONE',  ( 2.121784821875004390, -17.07198249233357856, -6.507072867603563182 ) ) ;
#7247=DIRECTION ( 'NONE',  ( 0.000000000000000000, 0.000000000000000000, 1.000000000000000000 ) ) ;
#7250=CARTESIAN_POINT ( 'NONE',  ( -2.121784821875005722, -29.67460370596585406, -11.69101089865440457 ) ) ;
#7253=DIRECTION ( 'NONE',  ( 8.673617379884034239E-17, 0.000000000000000000, 1.000000000000000000 ) ) ;
#7254=EDGE_CURVE ( 'NONE', #8704, #17065, #13157, .T. ) ;
#7255=ORIENTED_EDGE ( 'NONE', *, *, #3864, .F. ) ;
#7256=CARTESIAN_POINT ( 'NONE',  ( 4.243569643750003451, -18.12922721765884049, -5.881229758894760629 ) ) ;
#7258=CARTESIAN_POINT ( 'NONE',  ( 2.121784821874994176, -29.40573975142631014, -11.30703337789393359 ) ) ;
#7262=CARTESIAN_POINT ( 'NONE',  ( -4.243569643749998122, -23.68933379753673663, -13.82188488822120753 ) ) ;
#7264=FACE_OUTER_BOUND ( 'NONE', #3165, .T. ) ;
#7265=EDGE_CURVE ( 'NONE', #244, #12707, #750, .T. ) ;
#7266=FACE_OUTER_BOUND ( 'NONE', #7305, .T. ) ;
#7269=CARTESIAN_POINT ( 'NONE',  ( 2.121784821874994176, -28.08292909509171764, -9.417863975752439387 ) ) ;
#7270=DIRECTION ( 'NONE',  ( -0.000000000000000000, -0.5735764363510414965, -0.8191520442889950182 ) ) ;
#7271=CARTESIAN_POINT ( 'NONE',  ( 4.713407268011036227E-15, -16.97105695606709830, -8.008336910850223589 ) ) ;
#7276=CARTESIAN_POINT ( 'NONE',  ( -4.000000000000000888, -23.78734358949309424, -9.690367265603486047 ) ) ;
#7281=CARTESIAN_POINT ( 'NONE',  ( 2.121784821874994176, -27.08275518420459349, -7.989467598523504854 ) ) ;
#7286=CARTESIAN_POINT ( 'NONE',  ( 2.121784821875004390, -22.52454349039567205, -14.29413698862582294 ) ) ;
#7288=FACE_OUTER_BOUND ( 'NONE', #14278, .T. ) ;
#7290=( BOUNDED_CURVE ( )  B_SPLINE_CURVE ( 2, ( #15465, #2759, #3116, #1821, #8749, #12924, #10517, #6065, #10329 ),
 .UNSPECIFIED., .F., .T. ) 
 B_SPLINE_CURVE_WITH_KNOTS ( ( 3, 2, 2, 2, 3 ),
 ( 0.1293103448275862155, 0.1321839080459770166, 0.1379310344827586188, 0.1436781609195402210, 0.1465517241379310498 ),
 .UNSPECIFIED. ) 
 CURVE ( )  GEOMETRIC_REPRESENTATION_ITEM ( )  RATIONAL_B_SPLINE_CURVE ( ( 0.9330127018922194093, 0.9330127018922194093, 1.000000000000000000, 0.8660254037844387076, 1.000000000000000000, 0.8660254037844387076, 1.000000000000000000, 0.9330127018922189652, 0.9330127018922192983 ) ) 
 REPRESENTATION_ITEM ( '' )  );
#7291=CARTESIAN_POINT ( 'NONE',  ( -5.330712181944245322E-15, -25.52664227140541797, -3.631362988022969862 ) ) ;
#7292=ORIENTED_EDGE ( 'NONE', *, *, #150, .F. ) ;
#7294=VERTEX_POINT ( 'NONE', #3612 ) ;
#7296=ORIENTED_EDGE ( 'NONE', *, *, #1520, .T. ) ;
#7302=ORIENTED_EDGE ( 'NONE', *, *, #11437, .T. ) ;
#7304=CARTESIAN_POINT ( 'NONE',  ( -2.000000000000005773, -26.00120513392129240, -6.812612356863837704 ) ) ;
#7305=EDGE_LOOP ( 'NONE', ( #11922, #8056, #6759, #3763 ) ) ;
#7310=CARTESIAN_POINT ( 'NONE',  ( 1.533898589781675205E-14, -27.19300646412311551, -7.580370729157575482 ) ) ;
#7311=CARTESIAN_POINT ( 'NONE',  ( -4.243569643750000786, -21.02879941556483345, -5.750757902097718421 ) ) ;
#7314=ORIENTED_EDGE ( 'NONE', *, *, #13044, .T. ) ;
#7315=VERTEX_POINT ( 'NONE', #12038 ) ;
#7319=CARTESIAN_POINT ( 'NONE',  ( -4.000000000000004441, -26.36738592551933280, -9.348731678031116488 ) ) ;
#7321=AXIS2_PLACEMENT_3D ( 'NONE', #12551, #16752, #7247 ) ;
#7323=CARTESIAN_POINT ( 'NONE',  ( 3.999999999999996447, -27.63642379165096585, -11.16110557702728023 ) ) ;
#7325=CARTESIAN_POINT ( 'NONE',  ( -4.243569643750000786, -22.83556519007061425, -8.331086841608051685 ) ) ;
#7326=( BOUNDED_CURVE ( )  B_SPLINE_CURVE ( 2, ( #15353, #986, #14036, #13856, #1164, #15168, #9491, #18150, #2473 ),
 .UNSPECIFIED., .F., .F. ) 
 B_SPLINE_CURVE_WITH_KNOTS ( ( 3, 2, 2, 2, 3 ),
 ( 0.04310344827586207184, 0.04597701149425287293, 0.05172413793103448204, 0.05747126436781609116, 0.06034482758620690612 ),
 .UNSPECIFIED. ) 
 CURVE ( )  GEOMETRIC_REPRESENTATION_ITEM ( )  RATIONAL_B_SPLINE_CURVE ( ( 0.9330127018922194093, 0.9330127018922194093, 1.000000000000000000, 0.8660254037844387076, 1.000000000000000000, 0.8660254037844387076, 1.000000000000000000, 0.9330127018922191873, 0.9330127018922194093 ) ) 
 REPRESENTATION_ITEM ( '' )  );
#7328=ADVANCED_FACE ( 'NONE', ( #17732 ), #4998, .F. ) ;
#7330=CARTESIAN_POINT ( 'NONE',  ( 4.000000000000000888, -19.78664794594458698, -3.976781756687743918 ) ) ;
#7331=CARTESIAN_POINT ( 'NONE',  ( 1.071796769724485454, -21.61922704757731140, -13.56776313036627002 ) ) ;
#7332=CARTESIAN_POINT ( 'NONE',  ( -5.330712181944245322E-15, -26.81718925319525937, -5.474455087673208986 ) ) ;
#7335=CARTESIAN_POINT ( 'NONE',  ( -6.808698206972851885, -11.94148469789129763, 12.85951478023477712 ) ) ;
#7337=EDGE_CURVE ( 'NONE', #2970, #9801, #14521, .T. ) ;
#7338=CARTESIAN_POINT ( 'NONE',  ( -4.551717183842047376, -10.00000000000000178, -2.180355508048917201 ) ) ;
#7341=CARTESIAN_POINT ( 'NONE',  ( 4.243569643749996345, -22.15386951350980738, -3.086034408281590036 ) ) ;
#7342=CARTESIAN_POINT ( 'NONE',  ( 0.000000000000000000, 9.254131787996968228, 30.52396275209373044 ) ) ;
#7346=CARTESIAN_POINT ( 'NONE',  ( -4.000000000000000888, -22.17415986155084795, -7.386502140033922359 ) ) ;
#7350=CARTESIAN_POINT ( 'NONE',  ( -9.933259399355584662, -9.929220090424015766, 8.891678395390737677 ) ) ;
#7351=CONICAL_SURFACE ( 'NONE', #13539, 2.000000000000001776, 1.029744260000000189 ) ;
#7352=CARTESIAN_POINT ( 'NONE',  ( 6.262826437386884493, -14.35615764868780708, -3.437201991564796444 ) ) ;
#7354=CARTESIAN_POINT ( 'NONE',  ( -4.243569643750004339, -21.75595086079126261, -2.517747677556105845 ) ) ;
#7356=CARTESIAN_POINT ( 'NONE',  ( -4.243569643749997233, -25.01214445387132912, -15.71105429036270351 ) ) ;
#7357=CARTESIAN_POINT ( 'NONE',  ( 4.730628863548789710E-15, -21.46729876507041013, -14.91998009733462816 ) ) ;
#7358=CARTESIAN_POINT ( 'NONE',  ( 2.610818894029696136, -22.30731640688717121, -2.152030296976241708 ) ) ;
#7362=CARTESIAN_POINT ( 'NONE',  ( -2.121784821875005722, -27.09350974238616416, -8.004826699353927211 ) ) ;
#7364=CARTESIAN_POINT ( 'NONE',  ( 3.999999999999996447, -23.76478284628143456, -5.631829278076560641 ) ) ;
#7365=CARTESIAN_POINT ( 'NONE',  ( 3.999999999999996447, -22.21612646813362346, -3.420118758496274225 ) ) ;
#7367=ORIENTED_EDGE ( 'NONE', *, *, #11282, .T. ) ;
#7369=CARTESIAN_POINT ( 'NONE',  ( -5.577813053751546416E-15, -25.45076803941176991, -5.092196395636519490 ) ) ;
#7373=ORIENTED_EDGE ( 'NONE', *, *, #16662, .T. ) ;
#7374=CARTESIAN_POINT ( 'NONE',  ( 4.243569643750000786, -24.02932114822622722, -10.03594703378452024 ) ) ;
#7377=VERTEX_POINT ( 'NONE', #10833 ) ;
#7379=DIRECTION ( 'NONE',  ( 0.000000000000000000, 1.000000000000000000, 0.000000000000000000 ) ) ;
#7380=CARTESIAN_POINT ( 'NONE',  ( -5.330712181944245322E-15, -29.14017382041697601, -8.792020867043637722 ) ) ;
#7383=LINE ( 'NONE', #9060, #214 ) ;
#7384=CARTESIAN_POINT ( 'NONE',  ( 4.243569643750003451, -19.16166480309071574, -7.355703438614951573 ) ) ;
#7388=DIRECTION ( 'NONE',  ( -0.000000000000000000, -0.5735764363510414965, -0.8191520442889950182 ) ) ;
#7392=EDGE_LOOP ( 'NONE', ( #11545, #2321, #11951, #38, #11570 ) ) ;
#7402=CARTESIAN_POINT ( 'NONE',  ( 4.000000000000003553, -19.61562664118283195, -7.758855928260364188 ) ) ;
#7403=ORIENTED_EDGE ( 'NONE', *, *, #16258, .T. ) ;
#7407=( BOUNDED_CURVE ( )  B_SPLINE_CURVE ( 2, ( #6400, #10477, #11864, #574, #11961, #7870, #7693, #2154, #846 ),
 .UNSPECIFIED., .F., .T. ) 
 B_SPLINE_CURVE_WITH_KNOTS ( ( 3, 2, 2, 2, 3 ),
 ( 0.06034482758620690612, 0.06321839080459770721, 0.06896551724137930939, 0.07471264367816092544, 0.07758620689655172653 ),
 .UNSPECIFIED. ) 
 CURVE ( )  GEOMETRIC_REPRESENTATION_ITEM ( )  RATIONAL_B_SPLINE_CURVE ( ( 0.9330127018922194093, 0.9330127018922195203, 1.000000000000000000, 0.8660254037844387076, 1.000000000000000000, 0.8660254037844387076, 1.000000000000000000, 0.9330127018922194093, 0.9330127018922194093 ) ) 
 REPRESENTATION_ITEM ( '' )  );
#7408=CARTESIAN_POINT ( 'NONE',  ( -7.382399764659552943, -13.34693800548101095, 2.845224196420926610 ) ) ;
#7409=CARTESIAN_POINT ( 'NONE',  ( 4.730628863548789710E-15, -17.33754842334290913, -9.022085378453862603 ) ) ;
#7412=ORIENTED_EDGE ( 'NONE', *, *, #8820, .T. ) ;
#7416=CARTESIAN_POINT ( 'NONE',  ( -4.000000000000007105, 6.938893903907228378E-15, 30.00000000000000000 ) ) ;
#7422=CARTESIAN_POINT ( 'NONE',  ( -4.243569643750000786, -21.28690881192279960, -6.119376322027766157 ) ) ;
#7426=CARTESIAN_POINT ( 'NONE',  ( -5.577813053751546416E-15, -23.12778347219005681, -1.774630616266089866 ) ) ;
#7427=CARTESIAN_POINT ( 'NONE',  ( -5.279047395330986450E-15, -30.79721226948262824, -11.64886143429751542 ) ) ;
#7428=CARTESIAN_POINT ( 'NONE',  ( 4.243569643750003451, -20.45221178488055713, -9.198795538265191141 ) ) ;
#7429=CARTESIAN_POINT ( 'NONE',  ( 4.898587196589413815E-16, 2.700915433685006750, 35.11257424290206330 ) ) ;
#7434=( BOUNDED_CURVE ( )  B_SPLINE_CURVE ( 2, ( #12139, #10755, #3710, #9360, #7973, #13626, #938, #6582, #12233 ),
 .UNSPECIFIED., .F., .F. ) 
 B_SPLINE_CURVE_WITH_KNOTS ( ( 3, 2, 2, 2, 3 ),
 ( 0.5948275862068965747, 0.5977011494252874035, 0.6034482758620689502, 0.6091954022988506079, 0.6120689655172414367 ),
 .UNSPECIFIED. ) 
 CURVE ( )  GEOMETRIC_REPRESENTATION_ITEM ( )  RATIONAL_B_SPLINE_CURVE ( ( 0.9330127018922194093, 0.9330127018922194093, 1.000000000000000000, 0.8660254037844387076, 1.000000000000000000, 0.8660254037844387076, 1.000000000000000000, 0.9330127018922180770, 0.9330127018922194093 ) ) 
 REPRESENTATION_ITEM ( '' )  );
#7436=CARTESIAN_POINT ( 'NONE',  ( -4.243569643750000786, -19.73825243377498850, -3.907665802447479297 ) ) ;
#7438=DIRECTION ( 'NONE',  ( -0.000000000000000000, -0.000000000000000000, -1.000000000000000000 ) ) ;
#7439=CARTESIAN_POINT ( 'NONE',  ( 3.999999999999996447, -22.47423586449159671, -3.788737178426322849 ) ) ;
#7443=EDGE_CURVE ( 'NONE', #1052, #10458, #2512, .T. ) ;
#7444=CARTESIAN_POINT ( 'NONE',  ( -5.330712181944245322E-15, -29.62412893858816076, -9.483180404412477671 ) ) ;
#7448=CARTESIAN_POINT ( 'NONE',  ( 7.649231854195297942, -10.00000000000000178, -6.849627928938597066 ) ) ;
#7449=EDGE_LOOP ( 'NONE', ( #13796, #1636, #1188, #15944 ) ) ;
#7451=CARTESIAN_POINT ( 'NONE',  ( -4.243569643750005227, -28.20868576974048025, -11.73320817580729880 ) ) ;
#7452=VECTOR ( 'NONE', #11614, 1000.000000000000000 ) ;
#7455=CARTESIAN_POINT ( 'NONE',  ( 4.243569643750000786, -26.06193264454523018, -12.93881709073364661 ) ) ;
#7459=CARTESIAN_POINT ( 'NONE',  ( -2.121784821875005722, -27.86783793146007326, -9.110681959144070419 ) ) ;
#7461=CARTESIAN_POINT ( 'NONE',  ( -4.000000000000000888, -20.17381204048153265, -4.529709386582819519 ) ) ;
#7467=CARTESIAN_POINT ( 'NONE',  ( 2.000000000000004441, -23.10062930614460797, -14.74911449125581520 ) ) ;
#7468=AXIS2_PLACEMENT_3D ( 'NONE', #14362, #4257, #2702 ) ;
#7472=CARTESIAN_POINT ( 'NONE',  ( 4.243569643750003451, -22.51708695574430763, -12.14774289770557303 ) ) ;
#7475=CARTESIAN_POINT ( 'NONE',  ( -4.000000000000000888, -22.49679660770325285, -7.847275165953248255 ) ) ;
#7476=CARTESIAN_POINT ( 'NONE',  ( 2.121784821874994176, -28.63141156235240459, -10.20117811810379216 ) ) ;
#7481=CARTESIAN_POINT ( 'NONE',  ( 4.000000000000000888, -22.56132395608780783, -7.939429769928989522 ) ) ;
#7482=CARTESIAN_POINT ( 'NONE',  ( 4.243569643749996345, -23.47668016984439632, -4.975203810423082906 ) ) ;
#7484=DIRECTION ( 'NONE',  ( 0.000000000000000000, 0.000000000000000000, 1.000000000000000000 ) ) ;
#7485=CARTESIAN_POINT ( 'NONE',  ( 0.000000000000000000, 5.977523610840987267, 32.81826849749789687 ) ) ;
#7488=EDGE_LOOP ( 'NONE', ( #6238, #17361, #9256, #4487 ) ) ;
#7489=CARTESIAN_POINT ( 'NONE',  ( 1.071796769724495224, -20.84489885850341651, -12.46190787057612681 ) ) ;
#7490=DIRECTION ( 'NONE',  ( 0.9454169814551708351, 0.000000000000000000, 0.3258630558627246820 ) ) ;
#7496=CARTESIAN_POINT ( 'NONE',  ( 3.999999999999996447, -23.70025549648700292, -5.539674672087284257 ) ) ;
#7503=EDGE_CURVE ( 'NONE', #2915, #6628, #13320, .T. ) ;
#7504=CARTESIAN_POINT ( 'NONE',  ( 4.243569643750003451, -19.12940112854596819, -7.309626136123695161 ) ) ;
#7513=CARTESIAN_POINT ( 'NONE',  ( -1.071796769724496334, -26.43020497576804217, -6.490977304023350491 ) ) ;
#7516=ORIENTED_EDGE ( 'NONE', *, *, #17101, .F. ) ;
#7518=LINE ( 'NONE', #3362, #3942 ) ;
#7519=CARTESIAN_POINT ( 'NONE',  ( 4.243569643750003451, -18.87129173218799849, -6.941007716193646537 ) ) ;
#7524=CARTESIAN_POINT ( 'NONE',  ( 3.999999999999996447, -28.34622463093043621, -12.17480623082814262 ) ) ;
#7525=( BOUNDED_CURVE ( )  B_SPLINE_CURVE ( 2, ( #11542, #2942, #5719, #11359, #17048, #4320, #10150, #8577, #3125 ),
 .UNSPECIFIED., .F., .F. ) 
 B_SPLINE_CURVE_WITH_KNOTS ( ( 3, 2, 2, 2, 3 ),
 ( 0.5258620689655172376, 0.5287356321839080664, 0.5344827586206896131, 0.5402298850574712707, 0.5431034482758620996 ),
 .UNSPECIFIED. ) 
 CURVE ( )  GEOMETRIC_REPRESENTATION_ITEM ( )  RATIONAL_B_SPLINE_CURVE ( ( 0.9330127018922194093, 0.9330127018922194093, 1.000000000000000000, 0.8660254037844387076, 1.000000000000000000, 0.8660254037844387076, 1.000000000000000000, 0.9330127018922194093, 0.9330127018922194093 ) ) 
 REPRESENTATION_ITEM ( '' )  );
#7526=CARTESIAN_POINT ( 'NONE',  ( 4.730628863548789710E-15, -17.88603089060359963, -9.805399520805213598 ) ) ;
#7527=CYLINDRICAL_SURFACE ( 'NONE', #640, 4.000000000000000000 ) ;
#7529=CARTESIAN_POINT ( 'NONE',  ( -8.999999999999996447, -10.00000000000000000, 30.00000000000000000 ) ) ;
#7536=ORIENTED_EDGE ( 'NONE', *, *, #4113, .F. ) ;
#7538=CARTESIAN_POINT ( 'NONE',  ( -4.243569643750000786, -25.67476855000827030, -12.38588946083857856 ) ) ;
#7541=CARTESIAN_POINT ( 'NONE',  ( 5.940121053391558270, -10.00000000000000178, -9.400027718824636835 ) ) ;
#7542=ORIENTED_EDGE ( 'NONE', *, *, #1117, .T. ) ;
#7544=CARTESIAN_POINT ( 'NONE',  ( 3.999999999999996447, -21.89348972198121857, -2.959345732576948773 ) ) ;
#7545=CARTESIAN_POINT ( 'NONE',  ( -3.999999999999997335, -23.20764907453616743, -12.88879560662696200 ) ) ;
#7546=CARTESIAN_POINT ( 'NONE',  ( 2.121784821874994176, -27.82481969873374794, -9.049245555822391651 ) ) ;
#7547=DIRECTION ( 'NONE',  ( 0.000000000000000000, 0.000000000000000000, 1.000000000000000000 ) ) ;
#7550=CARTESIAN_POINT ( 'NONE',  ( -5.330712181944245322E-15, -27.30114437136644767, -6.165614625042047159 ) ) ;
#7557=CARTESIAN_POINT ( 'NONE',  ( 4.000000000000003553, -23.55179493634680199, -13.38028683320035483 ) ) ;
#7558=CARTESIAN_POINT ( 'NONE',  ( 4.898587196589413815E-16, 2.700915433685006750, 35.11257424290206330 ) ) ;
#7561=CARTESIAN_POINT ( 'NONE',  ( 4.730628863548789710E-15, -19.43468726875141073, -12.01711004038550001 ) ) ;
#7563=ORIENTED_EDGE ( 'NONE', *, *, #10366, .F. ) ;
#7565=CARTESIAN_POINT ( 'NONE',  ( -4.648177544792955347E-16, -29.83862777749724060, -11.35870953444733011 ) ) ;
#7569=CARTESIAN_POINT ( 'NONE',  ( 4.243569643750000786, -26.09419631908997772, -12.98489439322490213 ) ) ;
#7570=CARTESIAN_POINT ( 'NONE',  ( 1.071796769724495224, -23.36146547228866410, -16.05593746388732868 ) ) ;
#7571=CARTESIAN_POINT ( 'NONE',  ( -3.999999999999997335, -23.98197726361007298, -13.99465086641710698 ) ) ;
#7572=CARTESIAN_POINT ( 'NONE',  ( 4.299564228933482956E-15, -19.22018842984233089, -10.14158091035064579 ) ) ;
#7573=CARTESIAN_POINT ( 'NONE',  ( -4.243569643750000786, -20.54484429739364515, -5.059598364728879361 ) ) ;
#7576=CARTESIAN_POINT ( 'NONE',  ( 1.999999999999994449, -25.76460485463143968, -6.474712139601389360 ) ) ;
#7578=ORIENTED_EDGE ( 'NONE', *, *, #17316, .F. ) ;
#7579=ORIENTED_EDGE ( 'NONE', *, *, #8820, .F. ) ;
#7581=CARTESIAN_POINT ( 'NONE',  ( -14.99999999999999645, -10.00000000000000000, 30.00000000000000000 ) ) ;
#7587=CARTESIAN_POINT ( 'NONE',  ( -5.279047395330986450E-15, -25.63502434232325911, -4.276493035696559808 ) ) ;
#7589=CARTESIAN_POINT ( 'NONE',  ( 4.898587196589413815E-16, 2.700915433685006750, 35.11257424290206330 ) ) ;
#7591=DIRECTION ( 'NONE',  ( -0.000000000000000000, 1.000000000000000000, -0.000000000000000000 ) ) ;
#7593=CARTESIAN_POINT ( 'NONE',  ( -5.330712181944246111E-15, -24.97815980414473103, -2.848048845671618423 ) ) ;
#7596=CARTESIAN_POINT ( 'NONE',  ( -3.999999999999997335, -21.07824655387798174, -9.847693641197304615 ) ) ;
#7597=ORIENTED_EDGE ( 'NONE', *, *, #8491, .T. ) ;
#7599=CARTESIAN_POINT ( 'NONE',  ( -1.801903668194536401, -10.00000000000000178, 23.81845480839542972 ) ) ;
#7600=EDGE_CURVE ( 'NONE', #18352, #8879, #3036, .T. ) ;
#7601=FACE_OUTER_BOUND ( 'NONE', #14468, .T. ) ;
#7604=ADVANCED_FACE ( 'NONE', ( #4421 ), #4154, .F. ) ;
#7606=CARTESIAN_POINT ( 'NONE',  ( -2.121784821875005722, -24.25430638244851167, -3.950024080123402559 ) ) ;
#7609=CARTESIAN_POINT ( 'NONE',  ( 3.999999999999996447, -21.69990767541768761, -2.682881918636179197 ) ) ;
#7611=CARTESIAN_POINT ( 'NONE',  ( -1.999999999999996225, -22.73497432726586709, -14.22690506201481853 ) ) ;
#7612=CARTESIAN_POINT ( 'NONE',  ( 4.730628863548789710E-15, -17.11170270152969053, -8.699544261015072166 ) ) ;
#7613=CARTESIAN_POINT ( 'NONE',  ( 3.250767888004682415, -21.90484815091188509, -2.246271217071878823 ) ) ;
#7614=CARTESIAN_POINT ( 'NONE',  ( -4.000000000000000888, -25.52958201420443984, -12.17854159912454293 ) ) ;
#7615=VECTOR ( 'NONE', #17442, 1000.000000000000000 ) ;
#7618=AXIS2_PLACEMENT_3D ( 'NONE', #7734, #887, #16657 ) ;
#7620=CARTESIAN_POINT ( 'NONE',  ( 3.579096709490575479E-14, -22.86967407583208711, -1.406012196336041020 ) ) ;
#7626=CARTESIAN_POINT ( 'NONE',  ( 4.243569643749996345, -27.05794804431121037, -10.08978438695249835 ) ) ;
#7628=( BOUNDED_CURVE ( )  B_SPLINE_CURVE ( 2, ( #10479, #9542, #9718, #5376, #3982, #13812, #13993, #12415, #15219 ),
 .UNSPECIFIED., .F., .T. ) 
 B_SPLINE_CURVE_WITH_KNOTS ( ( 3, 2, 2, 2, 3 ),
 ( 0.2672413793103448620, 0.2701149425287356354, 0.2758620689655172376, 0.2816091954022988397, 0.2844827586206896686 ),
 .UNSPECIFIED. ) 
 CURVE ( )  GEOMETRIC_REPRESENTATION_ITEM ( )  RATIONAL_B_SPLINE_CURVE ( ( 0.9330127018922194093, 0.9330127018922200755, 1.000000000000000000, 0.8660254037844387076, 1.000000000000000000, 0.8660254037844387076, 1.000000000000000000, 0.9330127018922187432, 0.9330127018922194093 ) ) 
 REPRESENTATION_ITEM ( '' )  );
#7629=DIRECTION ( 'NONE',  ( -0.000000000000000000, -0.5735764363510414965, -0.8191520442889950182 ) ) ;
#7633=CARTESIAN_POINT ( 'NONE',  ( 4.243569643750003451, -22.77519635210228088, -12.51636131763562076 ) ) ;
#7634=VECTOR ( 'NONE', #5116, 1000.000000000000000 ) ;
#7636=CARTESIAN_POINT ( 'NONE',  ( -4.243569643750004339, -26.36965632068995191, -9.106801933805707350 ) ) ;
#7637=CYLINDRICAL_SURFACE ( 'NONE', #17082, 4.000000000000000000 ) ;
#7638=DIRECTION ( 'NONE',  ( -0.000000000000000000, -0.5735764363510414965, -0.8191520442889950182 ) ) ;
#7640=CARTESIAN_POINT ( 'NONE',  ( -2.121784821874996396, -20.64249580861881128, -11.60629434330255982 ) ) ;
#7642=CARTESIAN_POINT ( 'NONE',  ( -5.279047395330986450E-15, -23.37656712489597410, -1.051081862315407234 ) ) ;
#7645=EDGE_LOOP ( 'NONE', ( #1741, #6222, #10732, #4513 ) ) ;
#7647=CARTESIAN_POINT ( 'NONE',  ( 2.000000000000004441, -21.55197292799679687, -12.53740397167552878 ) ) ;
#7648=CARTESIAN_POINT ( 'NONE',  ( 3.579096709490575479E-14, -23.64400226490599266, -2.511867456126184894 ) ) ;
#7651=CARTESIAN_POINT ( 'NONE',  ( 4.243569643750003451, -20.71032118123852683, -9.567413958195238877 ) ) ;
#7656=CARTESIAN_POINT ( 'NONE',  ( -4.243569643750000786, -24.93270403547910874, -11.32611150353969087 ) ) ;
#7658=CARTESIAN_POINT ( 'NONE',  ( 9.849679380115679450, -9.940103771709287273, 9.708927138098026433 ) ) ;
#7659=DIRECTION ( 'NONE',  ( -0.000000000000000000, 1.000000000000000000, -0.000000000000000000 ) ) ;
#7660=CARTESIAN_POINT ( 'NONE',  ( -4.243569643750000786, -20.28673490103567545, -4.690979944798832513 ) ) ;
#7662=CARTESIAN_POINT ( 'NONE',  ( -4.000000000000004441, -21.78594414087033471, -2.805754725279534956 ) ) ;
#7664=ADVANCED_FACE ( 'NONE', ( #4247 ), #9889, .F. ) ;
#7665=CARTESIAN_POINT ( 'NONE',  ( -2.000000000000005773, -26.06573248371572760, -6.904766962853115864 ) ) ;
#7667=CARTESIAN_POINT ( 'NONE',  ( -2.465190328815646976E-33, -26.97786251599082519, -14.24690051095425858 ) ) ;
#7681=ORIENTED_EDGE ( 'NONE', *, *, #9909, .F. ) ;
#7683=CARTESIAN_POINT ( 'NONE',  ( 1.999999999999994449, -24.66763991940512568, -4.908083853891920256 ) ) ;
#7685=ORIENTED_EDGE ( 'NONE', *, *, #2931, .T. ) ;
#7690=CARTESIAN_POINT ( 'NONE',  ( -4.243569643750004339, -21.98179658260448832, -2.840288794994898058 ) ) ;
#7692=CARTESIAN_POINT ( 'NONE',  ( 4.243569643750000786, -23.51310235551028782, -9.298710193924424772 ) ) ;
#7693=CARTESIAN_POINT ( 'NONE',  ( 2.000000000000004441, -23.61684809886054381, -15.48635133111591067 ) ) ;
#7694=ORIENTED_EDGE ( 'NONE', *, *, #9322, .T. ) ;
#7697=CARTESIAN_POINT ( 'NONE',  ( 4.730628863548789710E-15, -22.79010942140500262, -16.80914949947612413 ) ) ;
#7701=CARTESIAN_POINT ( 'NONE',  ( -4.243569643750005227, -23.78856235711026912, -5.420617734505229990 ) ) ;
#7705=CARTESIAN_POINT ( 'NONE',  ( 2.121784821874994176, -29.40573975142631014, -11.30703337789393359 ) ) ;
#7706=CARTESIAN_POINT ( 'NONE',  ( -4.000000000000000888, -26.30391020327834539, -13.28439685891468613 ) ) ;
#7708=CARTESIAN_POINT ( 'NONE',  ( 2.121784821874994176, -24.75977061698287329, -4.671901819153075230 ) ) ;
#7710=EDGE_CURVE ( 'NONE', #1376, #1446, #11543, .T. ) ;
#7711=CARTESIAN_POINT ( 'NONE',  ( -6.158835246850665095E-15, -22.31750118613795664, -14.56500194951122218 ) ) ;
#7712=VECTOR ( 'NONE', #1545, 1000.000000000000000 ) ;
#7716=VERTEX_POINT ( 'NONE', #7565 ) ;
#7717=CARTESIAN_POINT ( 'NONE',  ( 2.769793372871041104, -22.34959508723814992, -1.882086548653340019 ) ) ;
#7718=CARTESIAN_POINT ( 'NONE',  ( 1.999999999999994449, -28.53928086477465698, -10.43736015284263807 ) ) ;
#7719=ORIENTED_EDGE ( 'NONE', *, *, #10628, .F. ) ;
#7721=CARTESIAN_POINT ( 'NONE',  ( -2.121784821874996396, -22.19115218676662238, -13.81800486288284624 ) ) ;
#7724=CARTESIAN_POINT ( 'NONE',  ( -0.5553297335970074355, -9.999999999999142020, -4.810349131758192343 ) ) ;
#7725=STYLED_ITEM ( 'NONE', ( #10690 ), #6498 ) ;
#7726=CARTESIAN_POINT ( 'NONE',  ( -4.243569643750005227, -27.43435758066657471, -10.62735291601715382 ) ) ;
#7727=EDGE_CURVE ( 'NONE', #9801, #5271, #17739, .T. ) ;
#7729=EDGE_CURVE ( 'NONE', #5758, #6383, #10348, .T. ) ;
#7730=CARTESIAN_POINT ( 'NONE',  ( -5.330712181944246111E-15, -28.84980074951425877, -8.377325144622332687 ) ) ;
#7733=DIRECTION ( 'NONE',  ( 0.000000000000000000, 0.8191520442889952403, -0.5735764363510413855 ) ) ;
#7734=CARTESIAN_POINT ( 'NONE',  ( 8.500000000000019540, 10.00000000000000000, 20.49999999999998934 ) ) ;
#7735=CARTESIAN_POINT ( 'NONE',  ( 2.121784821874994176, -26.53427271694390299, -7.206153456172153859 ) ) ;
#7736=ORIENTED_EDGE ( 'NONE', *, *, #4444, .T. ) ;
#7737=CARTESIAN_POINT ( 'NONE',  ( -6.158835246850665095E-15, -22.83371997885389248, -15.30223878937131587 ) ) ;
#7738=DIRECTION ( 'NONE',  ( -0.000000000000000000, 1.000000000000000000, -0.000000000000000000 ) ) ;
#7744=CARTESIAN_POINT ( 'NONE',  ( 1.743066579297358403E-15, -23.41446612136426708, -16.13163023522068684 ) ) ;
#7746=LINE ( 'NONE', #8954, #10141 ) ;
#7749=CARTESIAN_POINT ( 'NONE',  ( -4.243569643750000786, -22.35161007189942595, -7.639927304239214401 ) ) ;
#7755=CARTESIAN_POINT ( 'NONE',  ( -4.025001148619858249, -27.33870370935842686, -14.18005106542060467 ) ) ;
#7756=CARTESIAN_POINT ( 'NONE',  ( -4.648177544792955347E-16, -30.03220982406077155, -11.63517334838810058 ) ) ;
#7757=CARTESIAN_POINT ( 'NONE',  ( 7.496325586166000754, -13.00735673026645856, 5.000734971399987572 ) ) ;
#7758=CARTESIAN_POINT ( 'NONE',  ( 2.000000000000004441, -20.77764473892288777, -11.43154871188538557 ) ) ;
#7759=CARTESIAN_POINT ( 'NONE',  ( 4.243569643749996345, -22.70235198077049787, -3.869348550632942363 ) ) ;
#7763=CARTESIAN_POINT ( 'NONE',  ( -4.000000000000000888, -23.78734358949309424, -9.690367265603486047 ) ) ;
#7765=ORIENTED_EDGE ( 'NONE', *, *, #1981, .T. ) ;
#7766=EDGE_LOOP ( 'NONE', ( #16332, #4622, #13343, #5602 ) ) ;
#7774=CARTESIAN_POINT ( 'NONE',  ( 1.999999999999994449, -24.40953052304715953, -4.539465433961872520 ) ) ;
#7782=CARTESIAN_POINT ( 'NONE',  ( 3.999999999999996447, -26.60398620621909416, -9.686631897307085737 ) ) ;
#7783=CARTESIAN_POINT ( 'NONE',  ( -5.330712181944246111E-15, -24.46194101142878807, -2.110812005811521619 ) ) ;
#7784=CARTESIAN_POINT ( 'NONE',  ( -4.243569643749997233, -22.68915988664961247, -12.39348851099227389 ) ) ;
#7787=CARTESIAN_POINT ( 'NONE',  ( 4.299564228933482956E-15, -16.63909446626264454, -6.455396711050170211 ) ) ;
#7788=CARTESIAN_POINT ( 'NONE',  ( 4.898587196589413815E-16, 2.700915433685006750, 35.11257424290206330 ) ) ;
#7789=AXIS2_PLACEMENT_3D ( 'NONE', #13127, #16019, #9048 ) ;
#7790=DIRECTION ( 'NONE',  ( 0.000000000000000000, 0.8191520442889952403, -0.5735764363510413855 ) ) ;
#7791=CARTESIAN_POINT ( 'NONE',  ( -4.243569643750000786, -26.48136041362692339, -13.53782202311997551 ) ) ;
#7795=DIRECTION ( 'NONE',  ( -0.9454169814551723894, 0.000000000000000000, 0.3258630558627204632 ) ) ;
#7796=CARTESIAN_POINT ( 'NONE',  ( 4.243569643749996345, -23.70252589165761492, -5.297744927861876896 ) ) ;
#7799=CARTESIAN_POINT ( 'NONE',  ( 4.243569643750003451, -24.06574333389211873, -14.35945341728585767 ) ) ;
#7800=CARTESIAN_POINT ( 'NONE',  ( 4.000000000000000888, -26.69107429781530527, -13.83732448880975419 ) ) ;
#7801=CARTESIAN_POINT ( 'NONE',  ( -2.121784821874996396, -17.83555612322590278, -7.597569026563290251 ) ) ;
#7806=CARTESIAN_POINT ( 'NONE',  ( 4.000000000000000888, -20.23833938886609118, -4.621863990558560786 ) ) ;
#7807=CYLINDRICAL_SURFACE ( 'NONE', #15363, 4.000000000000000000 ) ;
#7810=CARTESIAN_POINT ( 'NONE',  ( -1.999999999999996225, -16.86298556082702760, -5.840836009612994317 ) ) ;
#7811=CARTESIAN_POINT ( 'NONE',  ( 2.000000000000004441, -22.77799255999219952, -14.28834146533649196 ) ) ;
#7814=FILL_AREA_STYLE ('',( #3288 ) ) ;
#7815=CARTESIAN_POINT ( 'NONE',  ( -4.243569643749997233, -23.17311500482080433, -13.08464804836111206 ) ) ;
#7820=CARTESIAN_POINT ( 'NONE',  ( -2.121784821875005722, -28.93253919143669251, -10.63123294135551689 ) ) ;
#7821=DIRECTION ( 'NONE',  ( -1.000000000000000000, 0.000000000000000000, 0.000000000000000000 ) ) ;
#7823=DIRECTION ( 'NONE',  ( -6.162975822039154730E-33, 0.5735764363510414965, 0.8191520442889950182 ) ) ;
#7825=CARTESIAN_POINT ( 'NONE',  ( -2.121784821874996396, -20.38438641226084158, -11.23767592337251209 ) ) ;
#7826=ORIENTED_EDGE ( 'NONE', *, *, #813, .T. ) ;
#7827=DIRECTION ( 'NONE',  ( -0.000000000000000000, -0.5735764363510414965, -0.8191520442889950182 ) ) ;
#7830=ORIENTED_EDGE ( 'NONE', *, *, #12879, .F. ) ;
#7832=DIRECTION ( 'NONE',  ( 1.049727191973305394E-16, 0.5150380737757255245, -0.8571673013836856869 ) ) ;
#7833=ADVANCED_FACE ( 'NONE', ( #15003 ), #3412, .F. ) ;
#7835=EDGE_CURVE ( 'NONE', #8639, #985, #10110, .T. ) ;
#7839=CARTESIAN_POINT ( 'NONE',  ( 4.730628863548789710E-15, -18.14414028696156578, -10.17401794073526311 ) ) ;
#7842=VERTEX_POINT ( 'NONE', #2300 ) ;
#7846=CARTESIAN_POINT ( 'NONE',  ( -3.577231619497362125, -28.57177006857940782, -13.28786742256294495 ) ) ;
#7847=CARTESIAN_POINT ( 'NONE',  ( 7.252352847715823891, -10.36846725531173163, 4.245760260470595071 ) ) ;
#7848=CARTESIAN_POINT ( 'NONE',  ( -1.999999999999996225, -18.92786073169077454, -8.789783369053376205 ) ) ;
#7849=CARTESIAN_POINT ( 'NONE',  ( 4.730628863548789710E-15, -16.59548390881375468, -7.962307421154977582 ) ) ;
#7850=EDGE_LOOP ( 'NONE', ( #10725, #8342, #8661, #7681 ) ) ;
#7852=CARTESIAN_POINT ( 'NONE',  ( -2.000000000000005773, -25.54951369099979175, -6.167530122993019503 ) ) ;
#7855=DIRECTION ( 'NONE',  ( 0.000000000000000000, 0.000000000000000000, 1.000000000000000000 ) ) ;
#7860=EDGE_LOOP ( 'NONE', ( #5305, #8129, #11187, #10956 ) ) ;
#7862=CARTESIAN_POINT ( 'NONE',  ( 4.713407268011036227E-15, -17.16463900263063636, -8.284800724790995829 ) ) ;
#7866=CARTESIAN_POINT ( 'NONE',  ( 8.500000000000019540, 10.00000000000000000, 22.49999999999999289 ) ) ;
#7868=AXIS2_PLACEMENT_3D ( 'NONE', #10875, #8367, #17950 ) ;
#7869=CARTESIAN_POINT ( 'NONE',  ( -5.330712181944245322E-15, -28.10773623498509721, -7.317547187323446778 ) ) ;
#7870=CARTESIAN_POINT ( 'NONE',  ( 4.000000000000003553, -24.58423252177867369, -14.85476051292054578 ) ) ;
#7873=CARTESIAN_POINT ( 'NONE',  ( -4.386042834387951395, -10.00000000000000178, 22.42214358049744760 ) ) ;
#7876=CARTESIAN_POINT ( 'NONE',  ( 4.243569643750003451, -24.84007152296602428, -15.46530867707600088 ) ) ;
#7877=ORIENTED_EDGE ( 'NONE', *, *, #6882, .F. ) ;
#7880=CARTESIAN_POINT ( 'NONE',  ( -2.121784821875005722, -23.73808758973257227, -3.212787240263307531 ) ) ;
#7883=CARTESIAN_POINT ( 'NONE',  ( 4.000000000000000888, -25.65863671238343358, -12.36285080908956502 ) ) ;
#7885=CARTESIAN_POINT ( 'NONE',  ( 4.243569643750000786, -20.67389899557263533, -5.243907574693898788 ) ) ;
#7888=B_SPLINE_CURVE_WITH_KNOTS ( 'NONE', 3,
 ( #13778, #17710, #7846, #15006, #6728, #4974, #7755, #18072, #16673, #2125, #10630, #2302, #16304, #3590, #9242, #3683, #13499, #814, #6458, #5065, #10721, #10813, #9329, #3860, #16396, #17980, #6549, #16488, #3766, #2396, #13685, #6642, #1001, #15186 ),
 .UNSPECIFIED., .F., .F.,
 ( 4, 2, 2, 2, 2, 2, 2, 2, 2, 2, 2, 2, 2, 2, 2, 2, 4 ),
 ( 0.007412722934092349537, 0.008215427948509459316, 0.009018132962926569962, 0.009820837977343680608, 0.01062354299176079125, 0.01142624800617790190, 0.01222895302059501255, 0.01303165803501212319, 0.01383436304942923384, 0.01463706806384634448, 0.01543977307826345513, 0.01624247809268056578, 0.01704518310709767295, 0.01784788812151478360, 0.01865059313593189425, 0.01945329815034900489, 0.02025600316476611554 ),
 .UNSPECIFIED. ) ;
#7889=DIRECTION ( 'NONE',  ( 0.000000000000000000, 0.000000000000000000, 1.000000000000000000 ) ) ;
#7893=ORIENTED_EDGE ( 'NONE', *, *, #1626, .F. ) ;
#7894=( BOUNDED_CURVE ( )  B_SPLINE_CURVE ( 2, ( #1849, #15588, #3236, #4803, #547, #11840, #9915, #6192, #17440 ),
 .UNSPECIFIED., .F., .T. ) 
 B_SPLINE_CURVE_WITH_KNOTS ( ( 3, 2, 2, 2, 3 ),
 ( 0.4568965517241379559, 0.4597701149425287293, 0.4655172413793103314, 0.4712643678160919336, 0.4741379310344827624 ),
 .UNSPECIFIED. ) 
 CURVE ( )  GEOMETRIC_REPRESENTATION_ITEM ( )  RATIONAL_B_SPLINE_CURVE ( ( 0.9330127018922194093, 0.9330127018922200755, 1.000000000000000000, 0.8660254037844387076, 1.000000000000000000, 0.8660254037844387076, 1.000000000000000000, 0.9330127018922187432, 0.9330127018922194093 ) ) 
 REPRESENTATION_ITEM ( '' )  );
#7897=CARTESIAN_POINT ( 'NONE',  ( 4.000000000000003553, -24.84234191813664339, -15.22337893285059707 ) ) ;
#7898=CARTESIAN_POINT ( 'NONE',  ( 2.000000000000004441, -21.22933618184438842, -12.07663094575620377 ) ) ;
#7899=VERTEX_POINT ( 'NONE', #10992 ) ;
#7901=SURFACE_STYLE_USAGE ( .BOTH. , #874 ) ;
#7903=CARTESIAN_POINT ( 'NONE',  ( -4.243569643749997233, -22.39878681574689523, -11.97879278857096885 ) ) ;
#7905=DIRECTION ( 'NONE',  ( 0.000000000000000000, 0.8191520442889952403, -0.5735764363510413855 ) ) ;
#7907=CARTESIAN_POINT ( 'NONE',  ( -1.661723472263481630E-14, -20.76884480799014554, -12.35329142993093576 ) ) ;
#7908=CARTESIAN_POINT ( 'NONE',  ( -2.121784821874996396, -22.22341586131136992, -13.86408216537410354 ) ) ;
#7911=CARTESIAN_POINT ( 'NONE',  ( 3.497645065122034769, -25.34683430723604403, -15.74138193774221328 ) ) ;
#7913=LINE ( 'NONE', #11813, #9176 ) ;
#7915=CARTESIAN_POINT ( 'NONE',  ( -2.121784821874996396, -19.86816761954490573, -10.50043908351241662 ) ) ;
#7923=CARTESIAN_POINT ( 'NONE',  ( -4.000000000000004441, -21.97952618743386566, -3.082218539220304976 ) ) ;
#7927=AXIS2_PLACEMENT_3D ( 'NONE', #14122, #16841, #14034 ) ;
#7929=CARTESIAN_POINT ( 'NONE',  ( 4.243569643750003451, -21.22653997395446623, -10.30465079805533080 ) ) ;
#7935=CIRCLE ( 'NONE', #4374, 0.4000000000000006883 ) ;
#7936=CARTESIAN_POINT ( 'NONE',  ( 6.772399938786841211, -14.05066417492660591, -1.433852700220792142 ) ) ;
#7939=CARTESIAN_POINT ( 'NONE',  ( -4.243569643749997233, -24.97988077932658513, -15.66497698787144977 ) ) ;
#7942=CARTESIAN_POINT ( 'NONE',  ( -5.577813053751546416E-15, -28.54808079570739920, -9.515617434797091434 ) ) ;
#7943=CARTESIAN_POINT ( 'NONE',  ( -1.999999999999996225, -20.73462650619655534, -11.37011230856371036 ) ) ;
#7945=ORIENTED_EDGE ( 'NONE', *, *, #548, .F. ) ;
#7952=EDGE_LOOP ( 'NONE', ( #14881, #6957, #3541, #11741 ) ) ;
#7955=CARTESIAN_POINT ( 'NONE',  ( -3.999999999999997335, -18.75526198665626154, -6.530127861826874103 ) ) ;
#7961=EDGE_CURVE ( 'NONE', #18219, #2970, #10606, .T. ) ;
#7964=CARTESIAN_POINT ( 'NONE',  ( 2.121784821874994176, -27.08275518420459349, -7.989467598523504854 ) ) ;
#7967=CARTESIAN_POINT ( 'NONE',  ( -1.071796769724505882, -19.72488052183944163, -10.86235591555482038 ) ) ;
#7968=VECTOR ( 'NONE', #14853, 1000.000000000000000 ) ;
#7971=CARTESIAN_POINT ( 'NONE',  ( -5.694236848974727927, -11.38679575279407530, 16.60313092159233861 ) ) ;
#7972=DIRECTION ( 'NONE',  ( -0.000000000000000000, 1.000000000000000000, -0.000000000000000000 ) ) ;
#7973=CARTESIAN_POINT ( 'NONE',  ( -4.000000000000000888, -22.69037865426678380, -8.123738979894017831 ) ) ;
#7974=CARTESIAN_POINT ( 'NONE',  ( 4.730628863548789710E-15, -22.27389062868906677, -16.07191265961602511 ) ) ;
#7978=CARTESIAN_POINT ( 'NONE',  ( 4.243569643750003451, -18.35507293947206264, -6.203770876333551954 ) ) ;
#7981=CARTESIAN_POINT ( 'NONE',  ( -1.999999999999996225, -21.70253674183399184, -12.75243138229462758 ) ) ;
#7983=CARTESIAN_POINT ( 'NONE',  ( -5.577813053751546416E-15, -28.80619019206536535, -9.884235854727139170 ) ) ;
#7985=CARTESIAN_POINT ( 'NONE',  ( -4.000000000000007105, 0.000000000000000000, 30.00000000000000000 ) ) ;
#7986=CARTESIAN_POINT ( 'NONE',  ( 1.071796769724485232, -24.66491314961903569, -3.969879301190459842 ) ) ;
#7987=CARTESIAN_POINT ( 'NONE',  ( 3.999999999999993339, 7.428752623566170548E-15, 30.00000000000000000 ) ) ;
#7988=ORIENTED_EDGE ( 'NONE', *, *, #11691, .F. ) ;
#7992=ADVANCED_FACE ( 'NONE', ( #5063 ), #2574, .F. ) ;
#7993=CARTESIAN_POINT ( 'NONE',  ( 2.000000000000004441, -23.03610195635016922, -14.65695988526653792 ) ) ;
#7997=CARTESIAN_POINT ( 'NONE',  ( -4.243569643750000786, -23.86800277550248950, -9.805560521328242629 ) ) ;
#8001=CYLINDRICAL_SURFACE ( 'NONE', #6098, 4.000000000000000000 ) ;
#8002=CARTESIAN_POINT ( 'NONE',  ( 4.243569643750003451, -23.03330574846024703, -12.88497973756566672 ) ) ;
#8003=( BOUNDED_CURVE ( )  B_SPLINE_CURVE ( 2, ( #6164, #519, #6352, #17510, #886, #705, #15072, #5044, #10793 ),
 .UNSPECIFIED., .F., .F. ) 
 B_SPLINE_CURVE_WITH_KNOTS ( ( 3, 2, 2, 2, 3 ),
 ( 0.9051724137931034253, 0.9080459770114942541, 0.9137931034482759118, 0.9195402298850574585, 0.9224137931034482873 ),
 .UNSPECIFIED. ) 
 CURVE ( )  GEOMETRIC_REPRESENTATION_ITEM ( )  RATIONAL_B_SPLINE_CURVE ( ( 0.9330127018922194093, 0.9330127018922194093, 1.000000000000000000, 0.8660254037844387076, 1.000000000000000000, 0.8660254037844387076, 1.000000000000000000, 0.9330127018922194093, 0.9330127018922194093 ) ) 
 REPRESENTATION_ITEM ( '' )  );
#8005=ADVANCED_FACE ( 'NONE', ( #15183 ), #8207, .F. ) ;
#8009=CARTESIAN_POINT ( 'NONE',  ( 4.243569643750000786, -21.41596351010179333, -6.303685531992786473 ) ) ;
#8012=CARTESIAN_POINT ( 'NONE',  ( -1.999999999999996225, -19.18597012804874069, -9.158401788983423941 ) ) ;
#8015=CARTESIAN_POINT ( 'NONE',  ( 4.000000000000000888, -20.49644878522406088, -4.990482410488609410 ) ) ;
#8022=CARTESIAN_POINT ( 'NONE',  ( 4.243569643750003451, -19.41977419944868544, -7.724321858545000197 ) ) ;
#8024=ORIENTED_EDGE ( 'NONE', *, *, #718, .F. ) ;
#8025=CARTESIAN_POINT ( 'NONE',  ( 3.999999999999996447, -23.70025549648699936, -5.539674672087284257 ) ) ;
#8026=CARTESIAN_POINT ( 'NONE',  ( 2.121784821875004390, -23.78282679764076590, -16.09115178578480254 ) ) ;
#8029=CARTESIAN_POINT ( 'NONE',  ( 7.467138643671723308, -10.10634134916229598, 13.07939629701359152 ) ) ;
#8031=CARTESIAN_POINT ( 'NONE',  ( -5.577813053751546416E-15, -24.09569370782749331, -3.156949689997003539 ) ) ;
#8032=CARTESIAN_POINT ( 'NONE',  ( 4.243569643749996345, -27.83227623338511947, -11.19563964674263978 ) ) ;
#8035=CARTESIAN_POINT ( 'NONE',  ( 3.999999999999996447, -24.28100163899737396, -6.369066117936657001 ) ) ;
#8038=ORIENTED_EDGE ( 'NONE', *, *, #17289, .T. ) ;
#8039=CARTESIAN_POINT ( 'NONE',  ( 4.299564228933482956E-15, -19.02660638327880349, -9.865117096409875330 ) ) ;
#8045=CARTESIAN_POINT ( 'NONE',  ( 1.999999999999994449, -23.63520233397325399, -3.433610174171729312 ) ) ;
#8049=CARTESIAN_POINT ( 'NONE',  ( 0.000000000000000000, 9.254131787996968228, 30.52396275209373044 ) ) ;
#8051=CARTESIAN_POINT ( 'NONE',  ( 4.243569643749997233, -22.67008830622574322, -3.823271248141685508 ) ) ;
#8053=CARTESIAN_POINT ( 'NONE',  ( -4.243569643750005227, -25.88570120251876361, -8.415642396436870953 ) ) ;
#8056=ORIENTED_EDGE ( 'NONE', *, *, #16997, .T. ) ;
#8057=CARTESIAN_POINT ( 'NONE',  ( -8.500000000000005329, 10.00000000000000000, -18.49999999999999645 ) ) ;
#8061=CARTESIAN_POINT ( 'NONE',  ( 4.243569643750003451, -18.61318233583002879, -6.572389296263599689 ) ) ;
#8066=AXIS2_PLACEMENT_3D ( 'NONE', #16222, #1955, #556 ) ;
#8068=CARTESIAN_POINT ( 'NONE',  ( 2.000000000000004441, -21.48744557820235457, -12.44524936568625151 ) ) ;
#8069=VERTEX_POINT ( 'NONE', #17219 ) ;
#8071=CARTESIAN_POINT ( 'NONE',  ( -4.000000000000004441, -27.46435086074564680, -10.91535996374058293 ) ) ;
#8076=CARTESIAN_POINT ( 'NONE',  ( 4.243569643750000786, -23.73894807732350998, -9.621251311363216985 ) ) ;
#8077=CARTESIAN_POINT ( 'NONE',  ( -4.000000000000004441, -22.49574498014980151, -3.819455379080400004 ) ) ;
#8079=CARTESIAN_POINT ( 'NONE',  ( 8.500000000000019540, -1.201721234452885367, -20.49999999999998934 ) ) ;
#8080=ORIENTED_EDGE ( 'NONE', *, *, #2647, .F. ) ;
#8082=EDGE_CURVE ( 'NONE', #4334, #11008, #12408, .T. ) ;
#8088=CARTESIAN_POINT ( 'NONE',  ( 4.243569643750000786, -24.25516687003944938, -10.35848815122331068 ) ) ;
#8094=CARTESIAN_POINT ( 'NONE',  ( -4.243569643750005227, -25.88570120251876361, -8.415642396436870953 ) ) ;
#8099=CARTESIAN_POINT ( 'NONE',  ( -2.121784821875005722, -24.51241577880647782, -4.318642500053448963 ) ) ;
#8100=EDGE_LOOP ( 'NONE', ( #7988, #16976 ) ) ;
#8106=CARTESIAN_POINT ( 'NONE',  ( 8.500000000000019540, 10.00000000000000000, -18.49999999999998934 ) ) ;
#8112=CARTESIAN_POINT ( 'NONE',  ( -5.330712181944246111E-15, -24.75231408233150887, -2.525507728232826210 ) ) ;
#8115=( BOUNDED_CURVE ( )  B_SPLINE_CURVE ( 2, ( #14630, #2019, #3308, #17518, #4875, #8949, #7647, #8852, #434 ),
 .UNSPECIFIED., .F., .T. ) 
 B_SPLINE_CURVE_WITH_KNOTS ( ( 3, 2, 2, 2, 3 ),
 ( 0.3362068965517241437, 0.3390804597701149170, 0.3448275862068965747, 0.3505747126436781769, 0.3534482758620690057 ),
 .UNSPECIFIED. ) 
 CURVE ( )  GEOMETRIC_REPRESENTATION_ITEM ( )  RATIONAL_B_SPLINE_CURVE ( ( 0.9330127018922194093, 0.9330127018922200755, 1.000000000000000000, 0.8660254037844387076, 1.000000000000000000, 0.8660254037844387076, 1.000000000000000000, 0.9330127018922187432, 0.9330127018922194093 ) ) 
 REPRESENTATION_ITEM ( '' )  );
#8116=ORIENTED_EDGE ( 'NONE', *, *, #2965, .F. ) ;
#8119=DIRECTION ( 'NONE',  ( 0.000000000000000000, 0.8191520442889952403, -0.5735764363510413855 ) ) ;
#8121=CARTESIAN_POINT ( 'NONE',  ( 3.250767888004682415, -21.90484815091188509, -2.246271217071878379 ) ) ;
#8123=CARTESIAN_POINT ( 'NONE',  ( 2.121784821874994176, -28.59914788780765704, -10.15510081561253664 ) ) ;
#8126=CARTESIAN_POINT ( 'NONE',  ( 4.000000000000000888, -21.33530432409240163, -6.188492276268029890 ) ) ;
#8129=ORIENTED_EDGE ( 'NONE', *, *, #10920, .T. ) ;
#8133=VECTOR ( 'NONE', #15814, 1000.000000000000000 ) ;
#8135=CARTESIAN_POINT ( 'NONE',  ( -4.243569643750004339, -27.43435758066658181, -10.62735291601715382 ) ) ;
#8138=CARTESIAN_POINT ( 'NONE',  ( -1.999999999999996225, -18.34711458918039995, -7.960391923204007014 ) ) ;
#8140=CARTESIAN_POINT ( 'NONE',  ( 0.000000000000000000, 9.254131787996968228, 30.52396275209373044 ) ) ;
#8144=CARTESIAN_POINT ( 'NONE',  ( -2.121784821875005722, -25.31900764242513091, -5.470575062334849470 ) ) ;
#8146=ORIENTED_EDGE ( 'NONE', *, *, #12602, .F. ) ;
#8147=CARTESIAN_POINT ( 'NONE',  ( -2.000000000000005773, -27.61438886186354225, -9.116477482433401391 ) ) ;
#8155=CARTESIAN_POINT ( 'NONE',  ( -2.121784821874996396, -16.77085486324927999, -6.077018044351843784 ) ) ;
#8158=CARTESIAN_POINT ( 'NONE',  ( -3.999999999999997335, -23.14312172474173224, -12.79664100063768650 ) ) ;
#8159=ORIENTED_EDGE ( 'NONE', *, *, #6799, .T. ) ;
#8160=CARTESIAN_POINT ( 'NONE',  ( 2.343145750507618530, -3.999999999999991562, 11.59510085796835099 ) ) ;
#8163=CARTESIAN_POINT ( 'NONE',  ( -8.999999999999996447, -10.00000000000000000, -3.713574246709372417 ) ) ;
#8164=CARTESIAN_POINT ( 'NONE',  ( -2.121784821875005722, -27.35161913874413386, -8.373445119283974947 ) ) ;
#8166=CARTESIAN_POINT ( 'NONE',  ( 4.299564228933482956E-15, -17.41342265533655009, -7.561251970840314307 ) ) ;
#8174=FACE_OUTER_BOUND ( 'NONE', #1527, .T. ) ;
#8175=CARTESIAN_POINT ( 'NONE',  ( -4.648177544792955347E-16, -30.09673717385520675, -11.72732795437737785 ) ) ;
#8179=CARTESIAN_POINT ( 'NONE',  ( 4.730628863548789710E-15, -19.91864238692259903, -12.70826957775434352 ) ) ;
#8182=DIRECTION ( 'NONE',  ( -0.000000000000000000, -0.5735764363510414965, -0.8191520442889950182 ) ) ;
#8185=CARTESIAN_POINT ( 'NONE',  ( 2.121784821874994176, -27.34086458056255964, -8.358086018453551702 ) ) ;
#8186=CARTESIAN_POINT ( 'NONE',  ( -0.4504932947034102630, -10.00000000000000178, -12.59063537424963997 ) ) ;
#8189=CARTESIAN_POINT ( 'NONE',  ( -4.000000000000000888, -20.69003083319747205, -5.266946226442914991 ) ) ;
#8193=CARTESIAN_POINT ( 'NONE',  ( 4.243569643749996345, -24.21874468437355432, -6.034981767721971480 ) ) ;
#8195=CARTESIAN_POINT ( 'NONE',  ( 3.579096709490575479E-14, -24.41833045397989821, -3.617722715916328546 ) ) ;
#8197=CARTESIAN_POINT ( 'NONE',  ( 3.579096709490575479E-14, -23.83758431146952361, -2.788331270066955359 ) ) ;
#8200=CARTESIAN_POINT ( 'NONE',  ( -1.071796769724494114, -29.85015447821607637, -11.37517136910324744 ) ) ;
#8204=CARTESIAN_POINT ( 'NONE',  ( 4.243569643749997233, -23.99289896256033572, -5.712440650283180155 ) ) ;
#8207=CYLINDRICAL_SURFACE ( 'NONE', #2940, 4.000000000000000000 ) ;
#8208=CARTESIAN_POINT ( 'NONE',  ( -2.121784821875005722, -29.41649430960788081, -11.32239247872435506 ) ) ;
#8212=CARTESIAN_POINT ( 'NONE',  ( -5.330712181944245322E-15, -30.14034773130410372, -10.22041724427257137 ) ) ;
#8213=ORIENTED_EDGE ( 'NONE', *, *, #17316, .T. ) ;
#8214=DIRECTION ( 'NONE',  ( 0.000000000000000000, 0.000000000000000000, -1.000000000000000000 ) ) ;
#8215=CARTESIAN_POINT ( 'NONE',  ( -2.000000000000005773, -25.03329489828385590, -5.430293283132924032 ) ) ;
#8218=VECTOR ( 'NONE', #4309, 1000.000000000000000 ) ;
#8219=ORIENTED_EDGE ( 'NONE', *, *, #2090, .T. ) ;
#8220=CARTESIAN_POINT ( 'NONE',  ( 1.999999999999994449, -28.34569881821112602, -10.16089633890186761 ) ) ;
#8225=( BOUNDED_CURVE ( )  B_SPLINE_CURVE ( 2, ( #7787, #6403, #16062, #13531, #12049, #3708, #17830, #4830, #3354 ),
 .UNSPECIFIED., .F., .T. ) 
 B_SPLINE_CURVE_WITH_KNOTS ( ( 3, 2, 2, 2, 3 ),
 ( 0.9741379310344827624, 0.9770114942528735913, 0.9827586206896551380, 0.9885057471264367956, 0.9913793103448276245 ),
 .UNSPECIFIED. ) 
 CURVE ( )  GEOMETRIC_REPRESENTATION_ITEM ( )  RATIONAL_B_SPLINE_CURVE ( ( 0.9330127018922194093, 0.9330127018922194093, 1.000000000000000000, 0.8660254037844387076, 1.000000000000000000, 0.8660254037844387076, 1.000000000000000000, 0.9330127018922180770, 0.9330127018922194093 ) ) 
 REPRESENTATION_ITEM ( '' )  );
#8227=CARTESIAN_POINT ( 'NONE',  ( -5.330712181944246111E-15, -30.17261140584885126, -10.26649454676382867 ) ) ;
#8229=CARTESIAN_POINT ( 'NONE',  ( -3.999999999999997335, -19.01337138301423479, -6.898746281756922727 ) ) ;
#8235=DIRECTION ( 'NONE',  ( -0.000000000000000000, -0.5735764363510414965, -0.8191520442889950182 ) ) ;
#8236=CARTESIAN_POINT ( 'NONE',  ( 0.000000000000000000, 5.977523610840987267, 32.81826849749789687 ) ) ;
#8239=CARTESIAN_POINT ( 'NONE',  ( 2.121784821874994176, -26.05031759877271469, -6.514993918803313910 ) ) ;
#8240=EDGE_CURVE ( 'NONE', #4607, #18076, #50, .T. ) ;
#8243=EDGE_CURVE ( 'NONE', #159, #9984, #14802, .T. ) ;
#8245=CARTESIAN_POINT ( 'NONE',  ( 4.000000000000000888, -24.43261708038802382, -10.61191331542860183 ) ) ;
#8246=LINE ( 'NONE', #2701, #14585 ) ;
#8254=CARTESIAN_POINT ( 'NONE',  ( -2.121784821874996396, -17.28707365596521939, -6.814254884211938368 ) ) ;
#8257=UNCERTAINTY_MEASURE_WITH_UNIT (LENGTH_MEASURE( 1.000000000000000082E-05 ), #8924, 'distance_accuracy_value', 'NONE');
#8258=CARTESIAN_POINT ( 'NONE',  ( -2.000000000000005773, -27.54986151206910350, -9.024322876444124120 ) ) ;
#8259=ORIENTED_EDGE ( 'NONE', *, *, #3999, .T. ) ;
#8262=CARTESIAN_POINT ( 'NONE',  ( 0.000000000000000000, 5.977523610840987267, 32.81826849749789687 ) ) ;
#8264=CARTESIAN_POINT ( 'NONE',  ( -4.243569643750004339, -24.56289054618417111, -6.526472994295373198 ) ) ;
#8271=DIRECTION ( 'NONE',  ( -0.000000000000000000, -0.5735764363510414965, -0.8191520442889950182 ) ) ;
#8273=CARTESIAN_POINT ( 'NONE',  ( 1.071796769724476128, -19.55435187671356800, -10.61881577092589524 ) ) ;
#8274=ORIENTED_EDGE ( 'NONE', *, *, #18132, .F. ) ;
#8277=CARTESIAN_POINT ( 'NONE',  ( -5.330712181944245322E-15, -28.07547256044035322, -7.271469884832189479 ) ) ;
#8283=CARTESIAN_POINT ( 'NONE',  ( 2.121784821874994176, -26.56653639148865409, -7.252230758663410271 ) ) ;
#8287=CARTESIAN_POINT ( 'NONE',  ( -4.000000000000000888, -20.94814022955544175, -5.635564646372960951 ) ) ;
#8288=CARTESIAN_POINT ( 'NONE',  ( -5.330712181944245322E-15, -26.01059738957660272, -4.322522525391808479 ) ) ;
#8297=CARTESIAN_POINT ( 'NONE',  ( 4.243569643750000786, -21.19011778828857118, -5.981144414553994260 ) ) ;
#8299=EDGE_CURVE ( 'NONE', #3027, #4548, #5452, .T. ) ;
#8300=EDGE_CURVE ( 'NONE', #1591, #1834, #14637, .T. ) ;
#8302=CARTESIAN_POINT ( 'NONE',  ( 4.243569643749997233, -28.34849502610105176, -11.93287648660273526 ) ) ;
#8307=CARTESIAN_POINT ( 'NONE',  ( 4.243569643750000786, -25.54571385182929077, -12.20158025087355114 ) ) ;
#8308=ORIENTED_EDGE ( 'NONE', *, *, #16301, .F. ) ;
#8309=CARTESIAN_POINT ( 'NONE',  ( -3.999999999999997335, -21.59446534659392114, -10.58493048105740009 ) ) ;
#8310=CARTESIAN_POINT ( 'NONE',  ( -3.999999999999997335, -19.85222692188257554, -8.096756147536344983 ) ) ;
#8311=VECTOR ( 'NONE', #15192, 1000.000000000000000 ) ;
#8317=ORIENTED_EDGE ( 'NONE', *, *, #4973, .F. ) ;
#8318=CARTESIAN_POINT ( 'NONE',  ( -4.243569643750004339, -27.17624818430860500, -10.25873449608710786 ) ) ;
#8320=CARTESIAN_POINT ( 'NONE',  ( -4.243569643750005227, -28.98301395881438580, -12.83906343559744201 ) ) ;
#8324=CARTESIAN_POINT ( 'NONE',  ( -4.000000000000000888, -24.04545298585106394, -10.05898568553353378 ) ) ;
#8326=CARTESIAN_POINT ( 'NONE',  ( -5.000000000000001776, 0.000000000000000000, -4.999999999999999112 ) ) ;
#8327=CARTESIAN_POINT ( 'NONE',  ( 4.730628863548789710E-15, -18.40224968331953548, -10.54263636066531085 ) ) ;
#8328=VERTEX_POINT ( 'NONE', #16904 ) ;
#8330=EDGE_LOOP ( 'NONE', ( #16677, #45, #581, #12119 ) ) ;
#8331=CARTESIAN_POINT ( 'NONE',  ( -4.000000000000000888, -24.81978117492496949, -11.16484094532367699 ) ) ;
#8338=CARTESIAN_POINT ( 'NONE',  ( 4.000000000000000888, -25.46505466581989907, -12.08638699514879455 ) ) ;
#8341=CARTESIAN_POINT ( 'NONE',  ( 4.000000000000000888, -24.88430852330952447, -11.25699554929942003 ) ) ;
#8342=ORIENTED_EDGE ( 'NONE', *, *, #6882, .T. ) ;
#8344=CARTESIAN_POINT ( 'NONE',  ( -1.661723472263481630E-14, -21.54317299706404754, -13.45914668972107897 ) ) ;
#8347=ADVANCED_FACE ( 'NONE', ( #2622 ), #3204, .F. ) ;
#8350=CARTESIAN_POINT ( 'NONE',  ( 4.243569643749997233, -24.99307287344746342, -7.140837027512114688 ) ) ;
#8354=VERTEX_POINT ( 'NONE', #1409 ) ;
#8358=AXIS2_PLACEMENT_3D ( 'NONE', #1954, #16041, #457 ) ;
#8359=CARTESIAN_POINT ( 'NONE',  ( -5.577813053751546416E-15, -24.67643985033786791, -3.986341135846375838 ) ) ;
#8360=VERTEX_POINT ( 'NONE', #15322 ) ;
#8361=CIRCLE ( 'NONE', #6886, 0.4000000000000006883 ) ;
#8363=CARTESIAN_POINT ( 'NONE',  ( 4.243569643750003451, -21.45238569576768484, -10.62719191549412656 ) ) ;
#8367=DIRECTION ( 'NONE',  ( -1.214671430232282197E-14, -0.8191520442889843601, 0.5735764363510568176 ) ) ;
#8368=CARTESIAN_POINT ( 'NONE',  ( -2.121784821875005722, -26.60955462421497586, -7.313667161985088150 ) ) ;
#8371=DIRECTION ( 'NONE',  ( -0.000000000000000000, -0.000000000000000000, 1.000000000000000000 ) ) ;
#8374=CARTESIAN_POINT ( 'NONE',  ( 4.243569643750003451, -19.64561992126190049, -8.046862975983790633 ) ) ;
#8375=FACE_BOUND ( 'NONE', #14935, .T. ) ;
#8378=CARTESIAN_POINT ( 'NONE',  ( 1.533898589781675205E-14, -28.03186200299146336, -8.778380594936995962 ) ) ;
#8380=CARTESIAN_POINT ( 'NONE',  ( -9.570896052262728659, -9.974056209534193584, -0.5937313284778471534 ) ) ;
#8381=VERTEX_POINT ( 'NONE', #6952 ) ;
#8382=CARTESIAN_POINT ( 'NONE',  ( 2.121784821874994176, -24.50166122062490359, -4.303283399223027494 ) ) ;
#8385=CYLINDRICAL_SURFACE ( 'NONE', #11215, 4.000000000000000000 ) ;
#8387=AXIS2_PLACEMENT_3D ( 'NONE', #5961, #14228, #12827 ) ;
#8390=CARTESIAN_POINT ( 'NONE',  ( -2.121784821875005722, -29.15838491324991466, -10.95377405879430910 ) ) ;
#8392=EDGE_LOOP ( 'NONE', ( #8779, #2161, #7367 ) ) ;
#8393=CARTESIAN_POINT ( 'NONE',  ( -1.071796769724496334, -20.49920871091334362, -11.96821117534496892 ) ) ;
#8394=CARTESIAN_POINT ( 'NONE',  ( 4.000000000000003553, -20.45448218005117624, -8.956865794039782003 ) ) ;
#8396=EDGE_CURVE ( 'NONE', #5051, #14905, #662, .T. ) ;
#8399=CARTESIAN_POINT ( 'NONE',  ( -4.000000000000004441, -24.10892870809205135, -6.123320504649964136 ) ) ;
#8406=CARTESIAN_POINT ( 'NONE',  ( 2.121784821874994176, -27.85708337327849549, -9.095322858313648950 ) ) ;
#8413=CARTESIAN_POINT ( 'NONE',  ( -4.243569643750005227, -25.36948240980282421, -7.678405556576772817 ) ) ;
#8418=CARTESIAN_POINT ( 'NONE',  ( 4.000000000000003553, -23.03557614363086259, -12.64304999334026114 ) ) ;
#8420=LINE ( 'NONE', #10076, #11035 ) ;
#8424=CARTESIAN_POINT ( 'NONE',  ( -4.000000000000004441, -28.49678844617752205, -12.38983364346077565 ) ) ;
#8427=CARTESIAN_POINT ( 'NONE',  ( 4.000000000000000888, -23.85187093787765278, -9.782521869579230867 ) ) ;
#8429=CARTESIAN_POINT ( 'NONE',  ( 3.999999999999996447, -22.73234526084956286, -4.157355598356369697 ) ) ;
#8431=CARTESIAN_POINT ( 'NONE',  ( -5.330712181944246111E-15, -27.55925376772441382, -6.534233044972094895 ) ) ;
#8432=ADVANCED_FACE ( 'NONE', ( #11214 ), #1863, .F. ) ;
#8434=CARTESIAN_POINT ( 'NONE',  ( 2.343145750507615865, 4.000000000000006217, -3.999999999999999112 ) ) ;
#8436=ORIENTED_EDGE ( 'NONE', *, *, #16928, .T. ) ;
#8437=EDGE_LOOP ( 'NONE', ( #7685, #15667, #7578, #12011 ) ) ;
#8440=CARTESIAN_POINT ( 'NONE',  ( 2.000000000000004441, -18.19655077534320498, -7.745364512584909988 ) ) ;
#8443=CARTESIAN_POINT ( 'NONE',  ( -2.121784821875005722, -26.31918155331226217, -6.898971439563784003 ) ) ;
#8446=CARTESIAN_POINT ( 'NONE',  ( -2.000000000000005773, -24.00085731285198065, -3.955819603412733976 ) ) ;
#8448=CARTESIAN_POINT ( 'NONE',  ( -4.243569643750000786, -24.67459463912114259, -10.95749308360964136 ) ) ;
#8450=ADVANCED_FACE ( 'NONE', ( #15236 ), #1358, .F. ) ;
#8452=DIRECTION ( 'NONE',  ( -0.000000000000000000, 1.000000000000000000, -0.000000000000000000 ) ) ;
#8453=CARTESIAN_POINT ( 'NONE',  ( -5.330712181944245322E-15, -23.94572221871285578, -1.373575165951426369 ) ) ;
#8455=EDGE_CURVE ( 'NONE', #8864, #4535, #4771, .T. ) ;
#8457=ORIENTED_EDGE ( 'NONE', *, *, #14795, .F. ) ;
#8461=CARTESIAN_POINT ( 'NONE',  ( 2.121784821875004390, -23.78282679764076590, -16.09115178578480254 ) ) ;
#8465=CARTESIAN_POINT ( 'NONE',  ( 2.769796806539087886, -22.38185710306395393, -1.928164938508226456 ) ) ;
#8469=CARTESIAN_POINT ( 'NONE',  ( -4.243569643749998122, -24.20555259025267958, -14.55912172808130478 ) ) ;
#8471=DIRECTION ( 'NONE',  ( -0.000000000000000000, -0.000000000000000000, -1.000000000000000000 ) ) ;
#8472=DIRECTION ( 'NONE',  ( 0.000000000000000000, 1.000000000000000000, 0.000000000000000000 ) ) ;
#8473=CARTESIAN_POINT ( 'NONE',  ( -4.243569643749997233, -22.14067741938892908, -11.61017436864092112 ) ) ;
#8474=ORIENTED_EDGE ( 'NONE', *, *, #9762, .F. ) ;
#8475=CARTESIAN_POINT ( 'NONE',  ( -1.999999999999996225, -20.92820855276008629, -11.64657612250448437 ) ) ;
#8476=CARTESIAN_POINT ( 'NONE',  ( 3.999999999999996447, -21.95801707177565731, -3.051500338566227821 ) ) ;
#8479=( BOUNDED_CURVE ( )  B_SPLINE_CURVE ( 2, ( #3323, #10164, #11935, #358, #7481, #15840, #449, #17345, #7572 ),
 .UNSPECIFIED., .F., .F. ) 
 B_SPLINE_CURVE_WITH_KNOTS ( ( 3, 2, 2, 2, 3 ),
 ( 0.6120689655172414367, 0.6149425287356321546, 0.6206896551724138122, 0.6264367816091953589, 0.6293103448275861878 ),
 .UNSPECIFIED. ) 
 CURVE ( )  GEOMETRIC_REPRESENTATION_ITEM ( )  RATIONAL_B_SPLINE_CURVE ( ( 0.9330127018922194093, 0.9330127018922206306, 1.000000000000000000, 0.8660254037844387076, 1.000000000000000000, 0.8660254037844387076, 1.000000000000000000, 0.9330127018922194093, 0.9330127018922194093 ) ) 
 REPRESENTATION_ITEM ( '' )  );
#8480=DIRECTION ( 'NONE',  ( -0.000000000000000000, -0.5735764363510414965, -0.8191520442889950182 ) ) ;
#8485=VERTEX_POINT ( 'NONE', #14373 ) ;
#8486=CARTESIAN_POINT ( 'NONE',  ( 4.243569643749997233, -26.83210232249799532, -9.767243269513704362 ) ) ;
#8490=CARTESIAN_POINT ( 'NONE',  ( -5.577813053751546416E-15, -28.99977223862889275, -10.16069966866791141 ) ) ;
#8491=EDGE_CURVE ( 'NONE', #18179, #18256, #16534, .T. ) ;
#8497=CARTESIAN_POINT ( 'NONE',  ( -4.243569643750000786, -22.35161007189942595, -7.639927304239214401 ) ) ;
#8499=DIRECTION ( 'NONE',  ( 0.000000000000000000, 0.8191520442889952403, -0.5735764363510413855 ) ) ;
#8501=CARTESIAN_POINT ( 'NONE',  ( -1.999999999999996225, -22.28328288434436644, -13.58182282814399855 ) ) ;
#8502=CARTESIAN_POINT ( 'NONE',  ( 4.299564228933482956E-15, -17.21984060877302269, -7.284788156899542066 ) ) ;
#8506=CARTESIAN_POINT ( 'NONE',  ( 4.000000000000000888, -25.98127345853583847, -12.82362383500889003 ) ) ;
#8508=AXIS2_PLACEMENT_3D ( 'NONE', #1905, #502, #3096 ) ;
#8511=CARTESIAN_POINT ( 'NONE',  ( 4.713407268011036227E-15, -20.00384236256828885, -12.33960334402152270 ) ) ;
#8515=EDGE_CURVE ( 'NONE', #17896, #5987, #10827, .T. ) ;
#8517=CARTESIAN_POINT ( 'NONE',  ( -6.428571428571426161, -14.26578344203648463, -2.827263138854405611 ) ) ;
#8518=CARTESIAN_POINT ( 'NONE',  ( -5.330712181944246111E-15, -26.52681618229254212, -5.059759365251904839 ) ) ;
#8519=VECTOR ( 'NONE', #16291, 1000.000000000000000 ) ;
#8521=CARTESIAN_POINT ( 'NONE',  ( -3.706921591972381904E-14, -16.70362181605707619, -6.547551317039444818 ) ) ;
#8531=CARTESIAN_POINT ( 'NONE',  ( -4.000000000000004441, -28.75489784253548819, -12.75845206339082161 ) ) ;
#8534=CARTESIAN_POINT ( 'NONE',  ( 2.121784821875004390, -19.65307645591326846, -10.19325706690404054 ) ) ;
#8538=CARTESIAN_POINT ( 'NONE',  ( 4.000000000000000888, -27.20729309053124112, -14.57456132866984966 ) ) ;
#8539=AXIS2_PLACEMENT_3D ( 'NONE', #4224, #9781, #5249 ) ;
#8540=CARTESIAN_POINT ( 'NONE',  ( 2.121784821874994176, -25.01788001334084299, -5.040520239083123855 ) ) ;
#8541=CARTESIAN_POINT ( 'NONE',  ( 2.000000000000004441, -24.13306689157648321, -16.22358817097600436 ) ) ;
#8545=CARTESIAN_POINT ( 'NONE',  ( -4.243569643749997233, -19.04336466309330689, -7.186753329480350061 ) ) ;
#8548=ORIENTED_EDGE ( 'NONE', *, *, #7503, .T. ) ;
#8551=FACE_OUTER_BOUND ( 'NONE', #2673, .T. ) ;
#8555=EDGE_LOOP ( 'NONE', ( #2049, #5241, #11223, #16936 ) ) ;
#8556=CARTESIAN_POINT ( 'NONE',  ( -4.243569643749998122, -18.55940954492211503, -6.495593792111509224 ) ) ;
#8558=AXIS2_PLACEMENT_3D ( 'NONE', #12821, #5600, #4208 ) ;
#8563=CARTESIAN_POINT ( 'NONE',  ( 4.730628863548789710E-15, -21.20918936871244398, -14.55136167740457864 ) ) ;
#8568=CARTESIAN_POINT ( 'NONE',  ( -4.243569643750000786, -24.12611217186045565, -10.17417894125829037 ) ) ;
#8569=CARTESIAN_POINT ( 'NONE',  ( 2.000000000000004441, -18.97087896441710697, -8.851219772375051420 ) ) ;
#8570=CARTESIAN_POINT ( 'NONE',  ( 2.000000000000004441, -16.90600379355336003, -5.902272412934671308 ) ) ;
#8577=CARTESIAN_POINT ( 'NONE',  ( -1.071796769724496334, -26.23662292920451478, -6.214513490082579139 ) ) ;
#8580=CARTESIAN_POINT ( 'NONE',  ( 4.243569643749997233, -25.79966473706611652, -8.292769589793515195 ) ) ;
#8584=CARTESIAN_POINT ( 'NONE',  ( -2.000000000000005773, -25.29140429464182560, -5.798911703062972656 ) ) ;
#8585=CARTESIAN_POINT ( 'NONE',  ( 15.00000000000000355, -10.00000000000000000, 30.00000000000000000 ) ) ;
#8587=CARTESIAN_POINT ( 'NONE',  ( -6.158835246850665095E-15, -22.64013793229036864, -15.02577497543054186 ) ) ;
#8588=CARTESIAN_POINT ( 'NONE',  ( -5.577813053751546416E-15, -29.51599103134483570, -10.89793650852800511 ) ) ;
#8589=( BOUNDED_CURVE ( )  B_SPLINE_CURVE ( 2, ( #12063, #687, #773, #4933, #6236, #11789, #10587 ),
 .UNSPECIFIED., .F., .F. ) 
 B_SPLINE_CURVE_WITH_KNOTS ( ( 3, 2, 2, 3 ),
 ( 0.03070921116881014309, 0.03448275862068965469, 0.04022988505747126381, 0.04310344827586207184 ),
 .UNSPECIFIED. ) 
 CURVE ( )  GEOMETRIC_REPRESENTATION_ITEM ( )  RATIONAL_B_SPLINE_CURVE ( ( 0.9395835397632845698, 0.9120326476671477556, 1.000000000000000000, 0.8660254037844387076, 1.000000000000000000, 0.9330127018922192983, 0.9330127018922194093 ) ) 
 REPRESENTATION_ITEM ( '' )  );
#8590=CARTESIAN_POINT ( 'NONE',  ( 4.243569643750003451, -18.90355540673274248, -6.987085018684902948 ) ) ;
#8592=CARTESIAN_POINT ( 'NONE',  ( 1.071796769724485232, -26.40715157433038129, -6.458053634711515834 ) ) ;
#8599=ORIENTED_EDGE ( 'NONE', *, *, #4973, .T. ) ;
#8601=CARTESIAN_POINT ( 'NONE',  ( -3.999999999999997335, -21.59446534659391759, -10.58493048105740009 ) ) ;
#8605=CARTESIAN_POINT ( 'NONE',  ( -7.634097544908422073, -10.16870601894835069, 11.61220938195502583 ) ) ;
#8606=CARTESIAN_POINT ( 'NONE',  ( -5.330712181944246111E-15, -26.78492557865051893, -5.428377785181952575 ) ) ;
#8608=VECTOR ( 'NONE', #17384, 1000.000000000000000 ) ;
#8613=CARTESIAN_POINT ( 'NONE',  ( -6.903430137606132000, -10.00000000000000178, 15.77881270003272540 ) ) ;
#8614=EDGE_CURVE ( 'NONE', #8360, #6360, #11860, .T. ) ;
#8617=CARTESIAN_POINT ( 'NONE',  ( -1.661723472263481630E-14, -21.60770034685848984, -13.55130129571035447 ) ) ;
#8621=CARTESIAN_POINT ( 'NONE',  ( -5.330712181944245322E-15, -26.26870678593457242, -4.691140945321855327 ) ) ;
#8625=DIRECTION ( 'NONE',  ( -1.000000000000000000, 0.000000000000000000, 0.000000000000000000 ) ) ;
#8627=CARTESIAN_POINT ( 'NONE',  ( 4.243569643750000786, -22.99688356279435197, -8.561473354064329300 ) ) ;
#8628=ADVANCED_FACE ( 'NONE', ( #1966 ), #6397, .F. ) ;
#8629=CARTESIAN_POINT ( 'NONE',  ( 1.006530391514320222, -10.00000000000244782, -4.211315095031120670 ) ) ;
#8631=CARTESIAN_POINT ( 'NONE',  ( 0.000000000000000000, -27.20729309053124112, -14.57456132866985321 ) ) ;
#8632=AXIS2_PLACEMENT_3D ( 'NONE', #6029, #10192, #7790 ) ;
#8634=CARTESIAN_POINT ( 'NONE',  ( -2.121784821875005722, -23.99619698609053842, -3.581405660193354379 ) ) ;
#8639=VERTEX_POINT ( 'NONE', #10472 ) ;
#8641=CARTESIAN_POINT ( 'NONE',  ( -5.330712181944245322E-15, -30.91467592037801282, -11.32627250406271635 ) ) ;
#8644=CARTESIAN_POINT ( 'NONE',  ( 4.551717183842062475, -10.00000000000000178, -2.180355508048892776 ) ) ;
#8646=AXIS2_PLACEMENT_3D ( 'NONE', #10526, #625, #6363 ) ;
#8647=CARTESIAN_POINT ( 'NONE',  ( 4.243569643750000786, -20.41578959921466918, -4.875289154763852828 ) ) ;
#8650=CARTESIAN_POINT ( 'NONE',  ( 4.243569643750003451, -24.58196212660805458, -15.09669025714595314 ) ) ;
#8652=CARTESIAN_POINT ( 'NONE',  ( 4.243569643750000786, -25.28760445547132107, -11.83296183094350340 ) ) ;
#8655=CARTESIAN_POINT ( 'NONE',  ( -5.330712181944245322E-15, -29.10791014587222847, -8.745943564552380423 ) ) ;
#8656=CARTESIAN_POINT ( 'NONE',  ( 1.071796769724485232, -25.18113194233497154, -4.707116141050555314 ) ) ;
#8658=CARTESIAN_POINT ( 'NONE',  ( 2.000000000000004441, -17.93844137898523527, -7.376746092654861364 ) ) ;
#8661=ORIENTED_EDGE ( 'NONE', *, *, #14627, .F. ) ;
#8668=CARTESIAN_POINT ( 'NONE',  ( -4.243569643749998122, -22.68915988664960892, -12.39348851099227389 ) ) ;
#8670=VERTEX_POINT ( 'NONE', #7866 ) ;
#8672=DIRECTION ( 'NONE',  ( -0.000000000000000000, -0.5735764363510414965, -0.8191520442889950182 ) ) ;
#8676=CARTESIAN_POINT ( 'NONE',  ( -1.071796769724486786, -17.40189595461771432, -7.544790136184399643 ) ) ;
#8677=CARTESIAN_POINT ( 'NONE',  ( -4.243569643749997233, -18.81751894128008118, -6.864212212041558736 ) ) ;
#8679=EDGE_CURVE ( 'NONE', #8864, #10774, #14448, .T. ) ;
#8680=CARTESIAN_POINT ( 'NONE',  ( 0.000000000000000000, 5.977523610840987267, 32.81826849749789687 ) ) ;
#8682=VERTEX_POINT ( 'NONE', #12131 ) ;
#8685=FACE_OUTER_BOUND ( 'NONE', #4396, .T. ) ;
#8693=EDGE_CURVE ( 'NONE', #2518, #269, #15300, .T. ) ;
#8694=CARTESIAN_POINT ( 'NONE',  ( -4.000000000000000888, -23.46470684334068935, -9.229594239684162815 ) ) ;
#8696=CARTESIAN_POINT ( 'NONE',  ( 3.999999999999996447, 6.938893903907228378E-15, 24.28148006742132026 ) ) ;
#8698=( BOUNDED_CURVE ( )  B_SPLINE_CURVE ( 2, ( #14027, #1429, #1337, #17195, #9756, #4467, #8446, #5854, #5677 ),
 .UNSPECIFIED., .F., .T. ) 
 B_SPLINE_CURVE_WITH_KNOTS ( ( 3, 2, 2, 2, 3 ),
 ( 0.7672413793103448620, 0.7701149425287355799, 0.7758620689655172376, 0.7816091954022988952, 0.7844827586206897241 ),
 .UNSPECIFIED. ) 
 CURVE ( )  GEOMETRIC_REPRESENTATION_ITEM ( )  RATIONAL_B_SPLINE_CURVE ( ( 0.9330127018922194093, 0.9330127018922206306, 1.000000000000000000, 0.8660254037844387076, 1.000000000000000000, 0.8660254037844387076, 1.000000000000000000, 0.9330127018922180770, 0.9330127018922194093 ) ) 
 REPRESENTATION_ITEM ( '' )  );
#8700=CARTESIAN_POINT ( 'NONE',  ( 4.243569643750003451, -19.38751052490393789, -7.678244556053742897 ) ) ;
#8704=VERTEX_POINT ( 'NONE', #6929 ) ;
#8714=CARTESIAN_POINT ( 'NONE',  ( -4.243569643750000786, -23.09367458642858040, -8.699705261538101198 ) ) ;
#8720=CARTESIAN_POINT ( 'NONE',  ( 4.243569643750000786, -22.22255537372044998, -7.455618094274186092 ) ) ;
#8721=CARTESIAN_POINT ( 'NONE',  ( -1.661723472263481630E-14, -20.51073541163217584, -11.98467301000088803 ) ) ;
#8726=( BOUNDED_CURVE ( )  B_SPLINE_CURVE ( 2, ( #8197, #16472, #5144, #12366, #8015, #16569, #1262, #2744, #5235 ),
 .UNSPECIFIED., .F., .F. ) 
 B_SPLINE_CURVE_WITH_KNOTS ( ( 3, 2, 2, 2, 3 ),
 ( 0.8879310344827586743, 0.8908045977011493921, 0.8965517241379310498, 0.9022988505747125965, 0.9051724137931034253 ),
 .UNSPECIFIED. ) 
 CURVE ( )  GEOMETRIC_REPRESENTATION_ITEM ( )  RATIONAL_B_SPLINE_CURVE ( ( 0.9330127018922194093, 0.9330127018922206306, 1.000000000000000000, 0.8660254037844387076, 1.000000000000000000, 0.8660254037844387076, 1.000000000000000000, 0.9330127018922194093, 0.9330127018922194093 ) ) 
 REPRESENTATION_ITEM ( '' )  );
#8727=CARTESIAN_POINT ( 'NONE',  ( 2.121784821874994176, -23.17885056429031465, -2.414113997081532847 ) ) ;
#8728=DIRECTION ( 'NONE',  ( 0.000000000000000000, 0.000000000000000000, -1.000000000000000000 ) ) ;
#8732=CARTESIAN_POINT ( 'NONE',  ( 4.730628863548789710E-15, -22.75784574686025152, -16.76307219698486506 ) ) ;
#8733=CARTESIAN_POINT ( 'NONE',  ( -14.99999999999999645, 10.00000000000000000, -30.00000000000000000 ) ) ;
#8736=CARTESIAN_POINT ( 'NONE',  ( 8.767957691173201340, -10.00000000000000178, -4.386791830708262729 ) ) ;
#8738=CARTESIAN_POINT ( 'NONE',  ( -5.330712181944246111E-15, -24.23609528961556947, -1.788270888372731182 ) ) ;
#8740=CARTESIAN_POINT ( 'NONE',  ( -4.243569643750000786, -26.73946980998488954, -13.90644044305002502 ) ) ;
#8744=EDGE_CURVE ( 'NONE', #3556, #11075, #6526, .T. ) ;
#8745=CARTESIAN_POINT ( 'NONE',  ( 2.121784821874994176, -28.34103849144968379, -9.786482395682487123 ) ) ;
#8749=CARTESIAN_POINT ( 'NONE',  ( 4.000000000000000888, -25.98127345853583847, -12.82362383500889003 ) ) ;
#8751=CARTESIAN_POINT ( 'NONE',  ( -4.243569643750000786, -25.15854975729233090, -11.64865262097848309 ) ) ;
#8753=CARTESIAN_POINT ( 'NONE',  ( -4.000000000000004441, -22.30216293358627055, -3.542991565139629984 ) ) ;
#8757=CARTESIAN_POINT ( 'NONE',  ( 8.500000000000019540, 0.000000000000000000, -20.49999999999998934 ) ) ;
#8763=CARTESIAN_POINT ( 'NONE',  ( -5.330712181944246111E-15, -27.59151744226916492, -6.580310347463351306 ) ) ;
#8766=EDGE_LOOP ( 'NONE', ( #12252, #8159, #17455, #2499, #17236 ) ) ;
#8767=CARTESIAN_POINT ( 'NONE',  ( -3.706921591972381904E-14, -16.70362181605707619, -6.547551317039444818 ) ) ;
#8768=CARTESIAN_POINT ( 'NONE',  ( -4.243569643749997233, -23.20537867936554832, -13.13072535085237114 ) ) ;
#8771=CARTESIAN_POINT ( 'NONE',  ( 4.000000000000003553, -21.74502916184101409, -10.79995789369002246 ) ) ;
#8772=CARTESIAN_POINT ( 'NONE',  ( -2.121784821874996396, -18.35177491594184218, -8.334805866423387499 ) ) ;
#8773=VERTEX_POINT ( 'NONE', #11193 ) ;
#8775=CARTESIAN_POINT ( 'NONE',  ( 1.071796769724485232, -24.34227640346663080, -3.509106275271134834 ) ) ;
#8777=ORIENTED_EDGE ( 'NONE', *, *, #10734, .T. ) ;
#8778=AXIS2_PLACEMENT_3D ( 'NONE', #10698, #12267, #16374 ) ;
#8779=ORIENTED_EDGE ( 'NONE', *, *, #4223, .F. ) ;
#8787=EDGE_CURVE ( 'NONE', #9317, #4535, #18098, .T. ) ;
#8788=CARTESIAN_POINT ( 'NONE',  ( 4.000000000000000888, -21.52888637065593258, -6.464956090208799466 ) ) ;
#8789=ORIENTED_EDGE ( 'NONE', *, *, #7710, .T. ) ;
#8795=CARTESIAN_POINT ( 'NONE',  ( -9.930521455883233983, -9.929686425557429530, 8.932771133217334736 ) ) ;
#8796=CARTESIAN_POINT ( 'NONE',  ( -2.121784821874996396, -18.06140184503912494, -7.920110144002082464 ) ) ;
#8804=CARTESIAN_POINT ( 'NONE',  ( 1.071796769724485232, -25.43924133869294835, -5.075734560980603050 ) ) ;
#8809=CARTESIAN_POINT ( 'NONE',  ( 4.299564228933482956E-15, -23.15635672500629738, -15.76301181529063555 ) ) ;
#8810=CIRCLE ( 'NONE', #13550, 2.000000000000001776 ) ;
#8811=CARTESIAN_POINT ( 'NONE',  ( -4.243569643750000786, -21.80312760463873900, -6.856613161887861629 ) ) ;
#8814=CARTESIAN_POINT ( 'NONE',  ( 4.730628863548789710E-15, -22.79010942140499907, -16.80914949947612413 ) ) ;
#8815=CARTESIAN_POINT ( 'NONE',  ( 1.533898589781675205E-14, -28.28997139934942595, -9.146999014867043698 ) ) ;
#8816=( BOUNDED_CURVE ( )  B_SPLINE_CURVE ( 3, ( #5409, #14116, #16923, #6969 ),
 .UNSPECIFIED., .F., .T. ) 
 B_SPLINE_CURVE_WITH_KNOTS ( ( 4, 4 ),
 ( 5.253488506341834174, 6.283185307179586232 ),
 .UNSPECIFIED. ) 
 CURVE ( )  GEOMETRIC_REPRESENTATION_ITEM ( )  RATIONAL_B_SPLINE_CURVE ( ( 1.000000000000000000, 0.9135782535825734962, 0.9135782535825734962, 1.000000000000000000 ) ) 
 REPRESENTATION_ITEM ( '' )  );
#8817=CARTESIAN_POINT ( 'NONE',  ( 4.243569643749996345, -24.25100835891830542, -6.081059070213228779 ) ) ;
#8818=CARTESIAN_POINT ( 'NONE',  ( 0.000000000000000000, -3.999999999999991562, 11.59510085796834566 ) ) ;
#8819=AXIS2_PLACEMENT_3D ( 'NONE', #1345, #7067, #12736 ) ;
#8820=EDGE_CURVE ( 'NONE', #177, #9284, #3446, .T. ) ;
#8821=AXIS2_PLACEMENT_3D ( 'NONE', #11066, #11606, #8824 ) ;
#8823=DIRECTION ( 'NONE',  ( -0.000000000000000000, -0.5735764363510414965, -0.8191520442889950182 ) ) ;
#8824=DIRECTION ( 'NONE',  ( 0.000000000000000000, 0.8191520442889949072, -0.5735764363510414965 ) ) ;
#8825=VERTEX_POINT ( 'NONE', #13617 ) ;
#8827=CARTESIAN_POINT ( 'NONE',  ( -4.243569643750000786, -21.28690881192279960, -6.119376322027766157 ) ) ;
#8832=CARTESIAN_POINT ( 'NONE',  ( 4.730628863548789710E-15, -22.49973635050228538, -16.39445377705482088 ) ) ;
#8835=LINE ( 'NONE', #4860, #12541 ) ;
#8837=CYLINDRICAL_SURFACE ( 'NONE', #1665, 4.000000000000000000 ) ;
#8838=VERTEX_POINT ( 'NONE', #1299 ) ;
#8840=CARTESIAN_POINT ( 'NONE',  ( 1.999999999999994449, -22.86087414489934488, -2.327754914381585660 ) ) ;
#8842=CARTESIAN_POINT ( 'NONE',  ( -5.330712181944246111E-15, -29.62412893858816432, -9.483180404412477671 ) ) ;
#8843=DIRECTION ( 'NONE',  ( -0.000000000000000000, -0.5735764363510414965, -0.8191520442889950182 ) ) ;
#8845=CARTESIAN_POINT ( 'NONE',  ( 1.533898589781675205E-14, -27.77375260663349366, -8.409762175006950002 ) ) ;
#8847=CARTESIAN_POINT ( 'NONE',  ( 2.121784821875004390, -21.45984223041904926, -12.77358600641437469 ) ) ;
#8848=CARTESIAN_POINT ( 'NONE',  ( -2.000000000000005773, -22.71031033106213570, -2.112727503762495296 ) ) ;
#8852=CARTESIAN_POINT ( 'NONE',  ( 1.071796769724485454, -21.10300825486137200, -12.83052629050617277 ) ) ;
#8853=EDGE_CURVE ( 'NONE', #451, #7377, #931, .T. ) ;
#8854=CARTESIAN_POINT ( 'NONE',  ( -4.000000000000004441, -27.98056965346157909, -11.65259680360067662 ) ) ;
#8855=AXIS2_PLACEMENT_3D ( 'NONE', #3398, #14625, #14812 ) ;
#8856=CARTESIAN_POINT ( 'NONE',  ( 4.000000000000000888, -23.33565214516171338, -9.045285029719133618 ) ) ;
#8860=CARTESIAN_POINT ( 'NONE',  ( -5.330712181944246111E-15, -28.10773623498509721, -7.317547187323447666 ) ) ;
#8861=EDGE_CURVE ( 'NONE', #13482, #9317, #13712, .T. ) ;
#8864=VERTEX_POINT ( 'NONE', #12313 ) ;
#8866=CARTESIAN_POINT ( 'NONE',  ( -4.000000000000007105, 6.938893903907228378E-15, 30.00000000000000000 ) ) ;
#8867=CARTESIAN_POINT ( 'NONE',  ( -4.243569643750000786, -25.96514162091098399, -12.80058518325988182 ) ) ;
#8869=DIRECTION ( 'NONE',  ( -0.000000000000000000, -0.5735764363510414965, -0.8191520442889950182 ) ) ;
#8870=DIRECTION ( 'NONE',  ( -0.000000000000000000, -0.5735764363510414965, -0.8191520442889950182 ) ) ;
#8871=CARTESIAN_POINT ( 'NONE',  ( 2.121784821874994176, -25.01788001334084299, -5.040520239083123855 ) ) ;
#8872=ADVANCED_FACE ( 'NONE', ( #9624 ), #2600, .F. ) ;
#8873=ORIENTED_EDGE ( 'NONE', *, *, #4053, .T. ) ;
#8874=CARTESIAN_POINT ( 'NONE',  ( -1.661723472263481630E-14, -21.60770034685848984, -13.55130129571035447 ) ) ;
#8877=CARTESIAN_POINT ( 'NONE',  ( 4.000000000000003553, -21.16428301933063949, -9.970566447840647939 ) ) ;
#8878=ORIENTED_EDGE ( 'NONE', *, *, #1348, .F. ) ;
#8879=VERTEX_POINT ( 'NONE', #12947 ) ;
#8880=CARTESIAN_POINT ( 'NONE',  ( 1.071796769724494780, -27.50411650955668463, -8.024681920420986714 ) ) ;
#8885=ORIENTED_EDGE ( 'NONE', *, *, #3365, .F. ) ;
#8887=CARTESIAN_POINT ( 'NONE',  ( -2.000000000000005773, -24.71065815213145100, -4.969520257213599024 ) ) ;
#8888=VERTEX_POINT ( 'NONE', #5637 ) ;
#8889=AXIS2_PLACEMENT_3D ( 'NONE', #14648, #16132, #15507 ) ;
#8892=CARTESIAN_POINT ( 'NONE',  ( -9.974300771894275996, -9.920519257017851089, 4.129833639286026425 ) ) ;
#8894=CARTESIAN_POINT ( 'NONE',  ( 2.121784821874994176, -24.72750694243812219, -4.625824516661818819 ) ) ;
#8899=DIRECTION ( 'NONE',  ( 0.000000000000000000, 0.8191520442889952403, -0.5735764363510413855 ) ) ;
#8900=CARTESIAN_POINT ( 'NONE',  ( 9.000000000000005329, -10.00000000000000000, 15.14468620625654616 ) ) ;
#8906=CARTESIAN_POINT ( 'NONE',  ( 2.121784821875004390, -18.87874826683935936, -9.087401807113897334 ) ) ;
#8911=CARTESIAN_POINT ( 'NONE',  ( 4.243569643750000786, -26.61041511180591357, -13.72213123308499760 ) ) ;
#8912=CARTESIAN_POINT ( 'NONE',  ( -3.999999999999997335, -24.94988749924751303, -15.37696994014802065 ) ) ;
#8913=CARTESIAN_POINT ( 'NONE',  ( -2.121784821875005722, -25.83522643514106676, -6.207811902194944054 ) ) ;
#8914=CARTESIAN_POINT ( 'NONE',  ( -7.037433860066684588, -13.81827297165700408, -0.01215148577350405948 ) ) ;
#8915=CARTESIAN_POINT ( 'NONE',  ( -6.262826437386821432, -14.35615764868811617, -3.437201991565423054 ) ) ;
#8916=CARTESIAN_POINT ( 'NONE',  ( -5.577813053751546416E-15, -23.57947491511155036, -2.419712850136908511 ) ) ;
#8918=ORIENTED_EDGE ( 'NONE', *, *, #8679, .T. ) ;
#8921=CARTESIAN_POINT ( 'NONE',  ( -6.938893903907228378E-15, 6.938893903907228378E-15, -30.00000000000000000 ) ) ;
#8924=( LENGTH_UNIT ( ) NAMED_UNIT ( * ) SI_UNIT ( .MILLI., .METRE. ) );
#8925=CARTESIAN_POINT ( 'NONE',  ( 4.243569643750003451, -23.77537026298940148, -13.94475769486455619 ) ) ;
#8926=CARTESIAN_POINT ( 'NONE',  ( -4.000000000000007105, 0.000000000000000000, 30.00000000000000000 ) ) ;
#8927=( BOUNDED_CURVE ( )  B_SPLINE_CURVE ( 3, ( #6620, #13656, #12265, #2734 ),
 .UNSPECIFIED., .F., .T. ) 
 B_SPLINE_CURVE_WITH_KNOTS ( ( 4, 4 ),
 ( -8.881784197001252323E-16, 1.570796326794896558 ),
 .UNSPECIFIED. ) 
 CURVE ( )  GEOMETRIC_REPRESENTATION_ITEM ( )  RATIONAL_B_SPLINE_CURVE ( ( 1.000000000000000000, 0.8047378541243648264, 0.8047378541243648264, 1.000000000000000000 ) ) 
 REPRESENTATION_ITEM ( '' )  );
#8931=CARTESIAN_POINT ( 'NONE',  ( -0.9156706748235758919, -10.00000000000091660, -4.445527249945649295 ) ) ;
#8934=CARTESIAN_POINT ( 'NONE',  ( -5.279047395330986450E-15, -23.57014917145950506, -1.327545676256177254 ) ) ;
#8936=CARTESIAN_POINT ( 'NONE',  ( -3.999999999999997335, -22.36879353566782314, -11.69078574084754152 ) ) ;
#8938=CARTESIAN_POINT ( 'NONE',  ( -4.243569643750004339, -26.11154692433198576, -8.738183513875661390 ) ) ;
#8939=CARTESIAN_POINT ( 'NONE',  ( 4.898587196589413815E-16, 2.700915433685006750, 35.11257424290206330 ) ) ;
#8941=CARTESIAN_POINT ( 'NONE',  ( 8.500000000000019540, 0.000000000000000000, -22.49999999999999289 ) ) ;
#8942=FACE_OUTER_BOUND ( 'NONE', #14157, .T. ) ;
#8943=CARTESIAN_POINT ( 'NONE',  ( 2.121784821875004390, -19.91118585227123816, -10.56187548683408828 ) ) ;
#8944=CARTESIAN_POINT ( 'NONE',  ( 5.040478647146458435, -15.02265568887750469, -7.935421837999466099 ) ) ;
#8949=CARTESIAN_POINT ( 'NONE',  ( 4.000000000000003553, -22.51935735091492674, -11.90581315348016567 ) ) ;
#8952=CARTESIAN_POINT ( 'NONE',  ( 3.999999999999996447, -28.15264258436690525, -11.89834241688737393 ) ) ;
#8953=VECTOR ( 'NONE', #4616, 1000.000000000000000 ) ;
#8954=CARTESIAN_POINT ( 'NONE',  ( 8.500000000000019540, 10.00000000000000000, -22.49999999999999289 ) ) ;
#8957=CARTESIAN_POINT ( 'NONE',  ( -2.121784821874996396, -20.15854069044762298, -10.91513480593371987 ) ) ;
#8964=CARTESIAN_POINT ( 'NONE',  ( -4.243569643750000786, -25.70703222455301784, -12.43196676332983408 ) ) ;
#8968=CARTESIAN_POINT ( 'NONE',  ( -1.071796769724491671, -22.62861123157153287, -15.00931314077462631 ) ) ;
#8971=CARTESIAN_POINT ( 'NONE',  ( -1.661723472263481630E-14, -21.80128239342201724, -13.82776510965112671 ) ) ;
#8972=CARTESIAN_POINT ( 'NONE',  ( -4.243569643749997233, -18.04319075220617563, -5.758356952251413752 ) ) ;
#8974=CARTESIAN_POINT ( 'NONE',  ( -3.999999999999997335, -22.94953967817819773, -12.52017718669691604 ) ) ;
#8975=CARTESIAN_POINT ( 'NONE',  ( 4.000000000000000888, -23.40017949495614857, -9.137439635708412666 ) ) ;
#8979=DIRECTION ( 'NONE',  ( 0.000000000000000000, 0.8191520442889952403, -0.5735764363510413855 ) ) ;
#8989=CARTESIAN_POINT ( 'NONE',  ( -3.999999999999997335, -20.56202776116204234, -9.110456801337207366 ) ) ;
#8995=CARTESIAN_POINT ( 'NONE',  ( -4.243569643750000786, -22.06123700099670870, -7.225231581817909365 ) ) ;
#8996=EDGE_CURVE ( 'NONE', #11449, #5080, #18325, .T. ) ;
#8998=CARTESIAN_POINT ( 'NONE',  ( 3.250762944584260072, -21.87258937905581746, -2.200190645090608133 ) ) ;
#9001=CARTESIAN_POINT ( 'NONE',  ( -3.678256433394857527, -9.999999999999056755, 21.51556408012798371 ) ) ;
#9005=VERTEX_POINT ( 'NONE', #4518 ) ;
#9008=CARTESIAN_POINT ( 'NONE',  ( 4.730628863548789710E-15, -17.59565781970087883, -9.390703798383910339 ) ) ;
#9011=DIRECTION ( 'NONE',  ( 0.000000000000000000, -0.5735764363510413855, -0.8191520442889951292 ) ) ;
#9012=CARTESIAN_POINT ( 'NONE',  ( -5.279047395330986450E-15, -30.53910287312466210, -11.28024301436746768 ) ) ;
#9013=CARTESIAN_POINT ( 'NONE',  ( -5.330712181944245322E-15, -25.52664227140541797, -3.631362988022969862 ) ) ;
#9014=CARTESIAN_POINT ( 'NONE',  ( -6.428571428571425272, -14.26578344203648285, -2.827263138854410496 ) ) ;
#9016=CARTESIAN_POINT ( 'NONE',  ( -1.071796769724496334, -21.53164629634521887, -13.44268485506515809 ) ) ;
#9018=EDGE_LOOP ( 'NONE', ( #15938, #6781 ) ) ;
#9019=CARTESIAN_POINT ( 'NONE',  ( -1.071796769724486786, -16.43398571898028138, -6.162471062453482418 ) ) ;
#9021=CARTESIAN_POINT ( 'NONE',  ( -14.99999999999999645, -10.00000000000000000, 30.00000000000000000 ) ) ;
#9024=CARTESIAN_POINT ( 'NONE',  ( 0.000000000000000000, 0.000000000000000000, 0.000000000000000000 ) ) ;
#9025=CARTESIAN_POINT ( 'NONE',  ( 2.121784821874994176, -28.08292909509171764, -9.417863975752439387 ) ) ;
#9029=CARTESIAN_POINT ( 'NONE',  ( -4.243569643750005227, -27.95057637338251411, -11.36458975587725106 ) ) ;
#9030=ADVANCED_FACE ( 'NONE', ( #4603 ), #11368, .F. ) ;
#9031=CARTESIAN_POINT ( 'NONE',  ( 1.475796370471763337E-14, -21.86580974321645598, -13.91991971564040220 ) ) ;
#9032=CARTESIAN_POINT ( 'NONE',  ( 4.243569643750003451, -21.71049509212565454, -10.99581033542417252 ) ) ;
#9033=CARTESIAN_POINT ( 'NONE',  ( 1.071796769724504328, -23.05172942167677519, -1.666014175620901705 ) ) ;
#9036=EDGE_CURVE ( 'NONE', #13551, #1052, #4434, .T. ) ;
#9038=CARTESIAN_POINT ( 'NONE',  ( 4.243569643750000786, -22.96461988824960443, -8.515396051573073777 ) ) ;
#9040=ADVANCED_FACE ( 'NONE', ( #10065 ), #15562, .F. ) ;
#9047=CARTESIAN_POINT ( 'NONE',  ( 4.000000000000000888, -25.20694526946192937, -11.71776857521874504 ) ) ;
#9048=DIRECTION ( 'NONE',  ( 1.000000000000000000, 0.000000000000000000, -8.673617379884034239E-17 ) ) ;
#9051=CARTESIAN_POINT ( 'NONE',  ( 2.121784821875004390, -19.68534013045801956, -10.23933436939529606 ) ) ;
#9053=ORIENTED_EDGE ( 'NONE', *, *, #13852, .F. ) ;
#9055=VECTOR ( 'NONE', #16510, 1000.000000000000000 ) ;
#9057=CARTESIAN_POINT ( 'NONE',  ( -4.243569643750005227, -27.69246697702454441, -10.99597133594720333 ) ) ;
#9060=CARTESIAN_POINT ( 'NONE',  ( 0.000000000000000000, -10.00099999999999767, 4.000000000000000000 ) ) ;
#9061=CARTESIAN_POINT ( 'NONE',  ( 4.243569643750000786, -26.83626083361913217, -14.04467235052378804 ) ) ;
#9063=CARTESIAN_POINT ( 'NONE',  ( -2.000000000000005773, -27.61438886186354225, -9.116477482433401391 ) ) ;
#9064=CARTESIAN_POINT ( 'NONE',  ( -1.999999999999996225, -19.96029831712264979, -10.26425704877356715 ) ) ;
#9068=FACE_OUTER_BOUND ( 'NONE', #17516, .T. ) ;
#9069=DIRECTION ( 'NONE',  ( -0.3258630558627247376, -2.016891894289822030E-15, 0.9454169814551708351 ) ) ;
#9073=ORIENTED_EDGE ( 'NONE', *, *, #718, .T. ) ;
#9075=CARTESIAN_POINT ( 'NONE',  ( -4.000000000000004441, -23.78629196193964646, -5.662547478730636463 ) ) ;
#9076=VERTEX_POINT ( 'NONE', #2859 ) ;
#9080=CARTESIAN_POINT ( 'NONE',  ( 3.999999999999996447, -27.31378704549856451, -10.70033255110795167 ) ) ;
#9081=CARTESIAN_POINT ( 'NONE',  ( 4.730628863548789710E-15, -16.82132963062697684, -8.284848538593767131 ) ) ;
#9083=CARTESIAN_POINT ( 'NONE',  ( 2.121784821874994176, -26.56653639148865409, -7.252230758663410271 ) ) ;
#9084=CARTESIAN_POINT ( 'NONE',  ( 3.604268994871578258, -25.13996932480225155, -16.02211701335336258 ) ) ;
#9086=CARTESIAN_POINT ( 'NONE',  ( 5.526342620815748674, -10.00000000000108713, 19.09106094340506132 ) ) ;
#9088=CARTESIAN_POINT ( 'NONE',  ( 2.343145750507616754, -3.999999999999992450, 25.54267522293724113 ) ) ;
#9089=CARTESIAN_POINT ( 'NONE',  ( 4.243569643750000786, -27.12663390452184942, -14.45936807294509308 ) ) ;
#9093=CARTESIAN_POINT ( 'NONE',  ( 4.243569643750000786, -21.15785411374382363, -5.935067112062737849 ) ) ;
#9095=ADVANCED_FACE ( 'NONE', ( #1474 ), #5793, .F. ) ;
#9097=CARTESIAN_POINT ( 'NONE',  ( 4.000000000000003553, -17.87338821647148990, -5.270681594739305531 ) ) ;
#9100=CARTESIAN_POINT ( 'NONE',  ( 4.713407268011036227E-15, -22.58493632614797164, -16.02578754332199651 ) ) ;
#9101=EDGE_CURVE ( 'NONE', #17559, #14256, #6345, .T. ) ;
#9102=CARTESIAN_POINT ( 'NONE',  ( -2.121784821875005722, -24.54467945335122536, -4.364719802544705374 ) ) ;
#9103=CARTESIAN_POINT ( 'NONE',  ( -7.471284260961007284, -13.12030862272409237, 4.270667233515101024 ) ) ;
#9104=CARTESIAN_POINT ( 'NONE',  ( -1.999999999999996225, -22.73497432726586709, -14.22690506201481853 ) ) ;
#9105=CARTESIAN_POINT ( 'NONE',  ( 1.071796769724476128, -16.90873056333943936, -6.840476965636138829 ) ) ;
#9107=CARTESIAN_POINT ( 'NONE',  ( 1.071796769724495224, -19.29624248035560896, -10.25019735099583862 ) ) ;
#9112=CARTESIAN_POINT ( 'NONE',  ( -3.999999999999997335, -17.78735175101882859, -5.147808788095962207 ) ) ;
#9113=CARTESIAN_POINT ( 'NONE',  ( 1.071796769724495224, -17.42494935605538942, -7.577713805496229860 ) ) ;
#9115=ORIENTED_EDGE ( 'NONE', *, *, #14732, .F. ) ;
#9117=CARTESIAN_POINT ( 'NONE',  ( 2.121784821875004390, -22.23417041949295481, -13.87944126620451790 ) ) ;
#9119=FACE_BOUND ( 'NONE', #13379, .T. ) ;
#9121=AXIS2_PLACEMENT_3D ( 'NONE', #15249, #2544, #6339 ) ;
#9122=CARTESIAN_POINT ( 'NONE',  ( -4.243569643750005227, -27.69246697702454441, -10.99597133594720333 ) ) ;
#9125=CARTESIAN_POINT ( 'NONE',  ( -2.121784821874996396, -21.41682399769271328, -12.71214960309270303 ) ) ;
#9126=CARTESIAN_POINT ( 'NONE',  ( 4.146003165456281003, -26.80775609498953926, -14.74331408136821864 ) ) ;
#9129=CARTESIAN_POINT ( 'NONE',  ( -4.243569643750005227, -25.85343752797401606, -8.369565093945613654 ) ) ;
#9131=CARTESIAN_POINT ( 'NONE',  ( 0.000000000000000000, 5.977523610840987267, 32.81826849749789687 ) ) ;
#9137=CARTESIAN_POINT ( 'NONE',  ( -1.661723472263481630E-14, -20.57526276142661459, -12.07682761599016175 ) ) ;
#9140=ADVANCED_FACE ( 'NONE', ( #13326 ), #16031, .F. ) ;
#9143=CARTESIAN_POINT ( 'NONE',  ( -4.243569643750004339, -24.85326361708688836, -6.941168716716676457 ) ) ;
#9152=CARTESIAN_POINT ( 'NONE',  ( 6.616872821575479513, -14.16311011709497691, -2.134317094043340024 ) ) ;
#9155=CARTESIAN_POINT ( 'NONE',  ( -2.121784821875005722, -29.93271310232382021, -12.05962931858445231 ) ) ;
#9158=CARTESIAN_POINT ( 'NONE',  ( -4.000000000000000888, -23.01301540041918869, -8.584512005813342839 ) ) ;
#9159=ORIENTED_EDGE ( 'NONE', *, *, #150, .T. ) ;
#9161=CARTESIAN_POINT ( 'NONE',  ( -4.000000000000004441, -23.27007316922370705, -4.925310638870541879 ) ) ;
#9162=CARTESIAN_POINT ( 'NONE',  ( 1.533898589781675205E-14, -28.28997139934942950, -9.146999014867043698 ) ) ;
#9168=ORIENTED_EDGE ( 'NONE', *, *, #3663, .F. ) ;
#9171=CARTESIAN_POINT ( 'NONE',  ( 4.000000000000000888, -22.30321455972984168, -7.570811349998943562 ) ) ;
#9175=CARTESIAN_POINT ( 'NONE',  ( 4.000000000000000888, -25.40052731602546032, -11.99423238915951551 ) ) ;
#9176=VECTOR ( 'NONE', #4772, 999.9999999999998863 ) ;
#9177=CARTESIAN_POINT ( 'NONE',  ( 4.243569643750003451, -17.83885414675612324, -5.466534036473456482 ) ) ;
#9178=CARTESIAN_POINT ( 'NONE',  ( 2.121784821875004390, -20.45966831953192511, -11.34518962918543927 ) ) ;
#9181=CARTESIAN_POINT ( 'NONE',  ( 4.950315044627312311, -10.00000000000193090, 20.01801554165957953 ) ) ;
#9184=CARTESIAN_POINT ( 'NONE',  ( -3.999999999999997335, -20.88466450731445079, -9.571229827256534151 ) ) ;
#9188=CARTESIAN_POINT ( 'NONE',  ( -2.121784821875005722, -24.77052517516444752, -4.687260919983497587 ) ) ;
#9192=CARTESIAN_POINT ( 'NONE',  ( -4.243569643750000786, -26.22325101726895369, -13.16920360318992955 ) ) ;
#9193=CARTESIAN_POINT ( 'NONE',  ( 4.713407268011036227E-15, -22.06871753343203579, -15.28855070346190459 ) ) ;
#9194=CARTESIAN_POINT ( 'NONE',  ( 2.121784821874994176, -23.98544242790896774, -3.566046559362932467 ) ) ;
#9196=CARTESIAN_POINT ( 'NONE',  ( 0.000000000000000000, 9.254131787996968228, 30.52396275209373044 ) ) ;
#9201=FACE_OUTER_BOUND ( 'NONE', #2426, .T. ) ;
#9204=( BOUNDED_CURVE ( )  B_SPLINE_CURVE ( 2, ( #10593, #9019, #7810, #9112, #6240, #10308, #4658, #16085, #7620 ),
 .UNSPECIFIED., .F., .F. ) 
 B_SPLINE_CURVE_WITH_KNOTS ( ( 3, 2, 2, 2, 3 ),
 ( 0.9741379310344827624, 0.9770114942528735913, 0.9827586206896551380, 0.9885057471264367956, 0.9913793103448276245 ),
 .UNSPECIFIED. ) 
 CURVE ( )  GEOMETRIC_REPRESENTATION_ITEM ( )  RATIONAL_B_SPLINE_CURVE ( ( 0.9330127018922194093, 0.9330127018922194093, 1.000000000000000000, 0.8660254037844387076, 1.000000000000000000, 0.8660254037844387076, 1.000000000000000000, 0.9330127018922180770, 0.9330127018922194093 ) ) 
 REPRESENTATION_ITEM ( '' )  );
#9206=CARTESIAN_POINT ( 'NONE',  ( 1.999999999999994449, -23.63520233397325399, -3.433610174171729312 ) ) ;
#9209=ORIENTED_EDGE ( 'NONE', *, *, #9036, .T. ) ;
#9212=CARTESIAN_POINT ( 'NONE',  ( -4.243569643749997233, -23.94744319389470633, -14.19050330815125704 ) ) ;
#9217=AXIS2_PLACEMENT_3D ( 'NONE', #13180, #15793, #403 ) ;
#9218=CARTESIAN_POINT ( 'NONE',  ( -2.121784821874996396, -22.99774405038527547, -14.96993742516424497 ) ) ;
#9219=EDGE_CURVE ( 'NONE', #10898, #17470, #1968, .T. ) ;
#9220=CARTESIAN_POINT ( 'NONE',  ( 3.064183985264992582, -21.85725672082847382, -2.451266466499125052 ) ) ;
#9221=CIRCLE ( 'NONE', #1247, 4.000000000000000888 ) ;
#9223=CARTESIAN_POINT ( 'NONE',  ( -2.121784821875005722, -25.80296276059631921, -6.161734599703687643 ) ) ;
#9225=DIRECTION ( 'NONE',  ( -0.000000000000000000, 1.000000000000000000, -0.000000000000000000 ) ) ;
#9226=DIRECTION ( 'NONE',  ( 0.000000000000000000, 0.000000000000000000, 1.000000000000000000 ) ) ;
#9228=DIRECTION ( 'NONE',  ( 0.000000000000000000, 0.8191520442889952403, -0.5735764363510413855 ) ) ;
#9231=PRODUCT_CONTEXT ( 'NONE', #16747, 'mechanical' ) ;
#9235=CARTESIAN_POINT ( 'NONE',  ( -2.121784821875005722, -25.31900764242513091, -5.470575062334849470 ) ) ;
#9237=CIRCLE ( 'NONE', #10716, 6.000000000000000000 ) ;
#9241=CARTESIAN_POINT ( 'NONE',  ( 3.579096709490575479E-14, -22.86967407583208711, -1.406012196336041020 ) ) ;
#9242=CARTESIAN_POINT ( 'NONE',  ( -3.083685924183309446, -24.92688910118828716, -15.92291992907465747 ) ) ;
#9243=CARTESIAN_POINT ( 'NONE',  ( 1.999999999999994449, -27.50684327934278528, -8.962886473122447129 ) ) ;
#9244=CARTESIAN_POINT ( 'NONE',  ( -4.243569643750005227, -22.27216965350720201, -3.254984517416200873 ) ) ;
#9246=CARTESIAN_POINT ( 'NONE',  ( 3.579096709490575479E-14, -26.48320562484364871, -6.566670075356708658 ) ) ;
#9248=CARTESIAN_POINT ( 'NONE',  ( -1.999999999999996225, -19.70218892076468364, -9.895638628843521190 ) ) ;
#9252=CARTESIAN_POINT ( 'NONE',  ( -5.577813053751546416E-15, -24.35380310418546657, -3.525568109927051275 ) ) ;
#9256=ORIENTED_EDGE ( 'NONE', *, *, #3538, .T. ) ;
#9258=CARTESIAN_POINT ( 'NONE',  ( -2.000000000000005773, -24.19443935941551160, -4.232283417353504440 ) ) ;
#9259=ORIENTED_EDGE ( 'NONE', *, *, #2542, .T. ) ;
#9261=DIRECTION ( 'NONE',  ( -0.000000000000000000, -0.5735764363510414965, -0.8191520442889950182 ) ) ;
#9262=VECTOR ( 'NONE', #7972, 1000.000000000000000 ) ;
#9266=CARTESIAN_POINT ( 'NONE',  ( 2.121784821874994176, -22.66263177157437525, -1.676877157221437376 ) ) ;
#9267=CARTESIAN_POINT ( 'NONE',  ( 4.243569643750003451, -22.25897755938633793, -11.77912447777552352 ) ) ;
#9268=CARTESIAN_POINT ( 'NONE',  ( -4.000000000000000888, -22.94848805062475350, -8.492357399824065567 ) ) ;
#9271=CARTESIAN_POINT ( 'NONE',  ( -6.503403972913312181, -10.00000000000000178, 16.98026834952698039 ) ) ;
#9275=CARTESIAN_POINT ( 'NONE',  ( 4.243569643750003451, -25.09818091932399398, -15.83392709700605039 ) ) ;
#9280=CARTESIAN_POINT ( 'NONE',  ( 4.730628863548789710E-15, -16.56322023426900714, -7.916230118663721171 ) ) ;
#9283=CARTESIAN_POINT ( 'NONE',  ( 4.000000000000003553, -24.51970517198423849, -14.76260590693127028 ) ) ;
#9284=VERTEX_POINT ( 'NONE', #7075 ) ;
#9285=CARTESIAN_POINT ( 'NONE',  ( 2.121784821874994176, -23.72733303155099804, -3.197428139432884286 ) ) ;
#9287=AXIS2_PLACEMENT_3D ( 'NONE', #11989, #14799, #6056 ) ;
#9289=CARTESIAN_POINT ( 'NONE',  ( 3.276967058447619152, -25.10900663730464188, -15.57833582608148326 ) ) ;
#9294=CARTESIAN_POINT ( 'NONE',  ( 4.000000000000000888, -21.59341372045036778, -6.557110696198077626 ) ) ;
#9296=VERTEX_POINT ( 'NONE', #4577 ) ;
#9298=CARTESIAN_POINT ( 'NONE',  ( -5.330712181944245322E-15, -30.14034773130410372, -10.22041724427257137 ) ) ;
#9302=CARTESIAN_POINT ( 'NONE',  ( 3.108848142585227681, -10.00000000000000178, -11.78746955954679976 ) ) ;
#9304=CARTESIAN_POINT ( 'NONE',  ( 2.121784821874994176, -28.88952095871037429, -10.56979653803383989 ) ) ;
#9305=ADVANCED_FACE ( 'NONE', ( #4301 ), #10234, .T. ) ;
#9306=( BOUNDED_CURVE ( )  B_SPLINE_CURVE ( 2, ( #5733, #8592, #4335, #15750, #11463, #8877, #14357, #6095, #13050 ),
 .UNSPECIFIED., .F., .T. ) 
 B_SPLINE_CURVE_WITH_KNOTS ( ( 3, 2, 2, 2, 3 ),
 ( 0.5431034482758620996, 0.5459770114942529284, 0.5517241379310344751, 0.5574712643678161328, 0.5603448275862069616 ),
 .UNSPECIFIED. ) 
 CURVE ( )  GEOMETRIC_REPRESENTATION_ITEM ( )  RATIONAL_B_SPLINE_CURVE ( ( 0.9330127018922194093, 0.9330127018922194093, 1.000000000000000000, 0.8660254037844387076, 1.000000000000000000, 0.8660254037844387076, 1.000000000000000000, 0.9330127018922180770, 0.9330127018922194093 ) ) 
 REPRESENTATION_ITEM ( '' )  );
#9307=DIRECTION ( 'NONE',  ( -0.000000000000000000, -0.5735764363510414965, -0.8191520442889950182 ) ) ;
#9309=CARTESIAN_POINT ( 'NONE',  ( 4.299564228933482956E-15, -23.09182937521185863, -15.67085720930136006 ) ) ;
#9311=CARTESIAN_POINT ( 'NONE',  ( 4.243569643749996345, -25.76740106252136542, -8.246692287302257895 ) ) ;
#9312=B_SPLINE_CURVE_WITH_KNOTS ( 'NONE', 3,
 ( #11873, #5012, #673, #6499, #5100, #14868 ),
 .UNSPECIFIED., .F., .F.,
 ( 4, 2, 4 ),
 ( 0.000000000000000000, 0.001225725630168212092, 0.002451451260336424184 ),
 .UNSPECIFIED. ) ;
#9313=ORIENTED_EDGE ( 'NONE', *, *, #548, .T. ) ;
#9315=LINE ( 'NONE', #12000, #17477 ) ;
#9317=VERTEX_POINT ( 'NONE', #15620 ) ;
#9322=EDGE_CURVE ( 'NONE', #6383, #8354, #9936, .T. ) ;
#9324=CARTESIAN_POINT ( 'NONE',  ( -4.243569643750000786, -22.09350067554145625, -7.271308884309165776 ) ) ;
#9329=CARTESIAN_POINT ( 'NONE',  ( -0.3167908498167790188, -23.77648345714862543, -16.77767476633956534 ) ) ;
#9331=CARTESIAN_POINT ( 'NONE',  ( -1.071796769724505882, -17.66000535097569113, -7.913408556114437609 ) ) ;
#9332=CARTESIAN_POINT ( 'NONE',  ( -4.243569643750000786, -19.77051610831973605, -3.953743104938735708 ) ) ;
#9335=CARTESIAN_POINT ( 'NONE',  ( -5.279047395330986450E-15, -27.50631746662347155, -6.948976581196172120 ) ) ;
#9337=ORIENTED_EDGE ( 'NONE', *, *, #2769, .F. ) ;
#9338=ORIENTED_EDGE ( 'NONE', *, *, #16261, .T. ) ;
#9339=CARTESIAN_POINT ( 'NONE',  ( -4.000000000000003553, 6.938893903907228378E-15, 0.000000000000000000 ) ) ;
#9343=ORIENTED_EDGE ( 'NONE', *, *, #1627, .T. ) ;
#9346=CARTESIAN_POINT ( 'NONE',  ( 4.713407268011036227E-15, -16.90652960627266310, -7.916182304860950758 ) ) ;
#9348=CARTESIAN_POINT ( 'NONE',  ( -1.071796769724496334, -24.88154859762023463, -4.279266784443063187 ) ) ;
#9351=ADVANCED_FACE ( 'NONE', ( #14323 ), #8837, .F. ) ;
#9352=CARTESIAN_POINT ( 'NONE',  ( 3.250762944584260072, -21.87258937905581746, -2.200190645090608133 ) ) ;
#9354=CARTESIAN_POINT ( 'NONE',  ( -2.121784821874996396, -21.19097827587949467, -12.38960848565391260 ) ) ;
#9355=CARTESIAN_POINT ( 'NONE',  ( 4.898587196589413815E-16, 2.700915433685006750, 35.11257424290206330 ) ) ;
#9356=ORIENTED_EDGE ( 'NONE', *, *, #4113, .T. ) ;
#9358=CARTESIAN_POINT ( 'NONE',  ( -6.681132651088828034, -10.00000000000000178, 19.92483346546715950 ) ) ;
#9360=CARTESIAN_POINT ( 'NONE',  ( -3.999999999999997335, -20.82013715752001559, -9.479075221267256879 ) ) ;
#9361=CARTESIAN_POINT ( 'NONE',  ( -5.330712181944245322E-15, -30.68883019856478711, -11.00373138662392236 ) ) ;
#9365=CARTESIAN_POINT ( 'NONE',  ( 4.243569643750003451, -17.83885414675612324, -5.466534036473456482 ) ) ;
#9368=CARTESIAN_POINT ( 'NONE',  ( 4.000000000000000888, -25.40052731602546032, -11.99423238915951551 ) ) ;
#9371=CARTESIAN_POINT ( 'NONE',  ( -2.121784821874996396, -17.06122793415199723, -6.491713766773147931 ) ) ;
#9382=CARTESIAN_POINT ( 'NONE',  ( -5.577813053751546416E-15, -26.41867827504920996, -6.474515469367432274 ) ) ;
#9385=VECTOR ( 'NONE', #7889, 1000.000000000000000 ) ;
#9386=CARTESIAN_POINT ( 'NONE',  ( 4.243569643750003451, -21.71049509212565454, -10.99581033542417252 ) ) ;
#9388=FACE_OUTER_BOUND ( 'NONE', #15084, .T. ) ;
#9389=CARTESIAN_POINT ( 'NONE',  ( 4.730628863548789710E-15, -21.75767183597312737, -15.33467581975593141 ) ) ;
#9390=ADVANCED_FACE ( 'NONE', ( #10035 ), #3196, .F. ) ;
#9392=VECTOR ( 'NONE', #53, 1000.000000000000000 ) ;
#9393=CARTESIAN_POINT ( 'NONE',  ( 3.878940541574451562, -25.96705729343073443, -15.31857466066475304 ) ) ;
#9395=CARTESIAN_POINT ( 'NONE',  ( -4.000000000000004441, -28.17415170002511360, -11.92906061754144886 ) ) ;
#9397=CARTESIAN_POINT ( 'NONE',  ( 2.121784821874994176, -24.72750694243812219, -4.625824516661818819 ) ) ;
#9399=CYLINDRICAL_SURFACE ( 'NONE', #14866, 4.000000000000000000 ) ;
#9402=DIRECTION ( 'NONE',  ( 0.000000000000000000, 0.8191520442889952403, -0.5735764363510413855 ) ) ;
#9409=EDGE_LOOP ( 'NONE', ( #6958, #11642, #17188, #11419 ) ) ;
#9410=CARTESIAN_POINT ( 'NONE',  ( 4.243569643750003451, -18.90355540673274248, -6.987085018684902948 ) ) ;
#9412=( BOUNDED_CURVE ( )  B_SPLINE_CURVE ( 2, ( #16221, #10545, #3515, #5076, #740, #9161, #2136, #6197, #11847 ),
 .UNSPECIFIED., .F., .T. ) 
 B_SPLINE_CURVE_WITH_KNOTS ( ( 3, 2, 2, 2, 3 ),
 ( 0.7672413793103448620, 0.7701149425287355799, 0.7758620689655172376, 0.7816091954022988952, 0.7844827586206897241 ),
 .UNSPECIFIED. ) 
 CURVE ( )  GEOMETRIC_REPRESENTATION_ITEM ( )  RATIONAL_B_SPLINE_CURVE ( ( 0.9330127018922194093, 0.9330127018922206306, 1.000000000000000000, 0.8660254037844387076, 1.000000000000000000, 0.8660254037844387076, 1.000000000000000000, 0.9330127018922180770, 0.9330127018922194093 ) ) 
 REPRESENTATION_ITEM ( '' )  );
#9414=CARTESIAN_POINT ( 'NONE',  ( 3.579096709490575479E-14, -25.12813129325936501, -4.631423369717193594 ) ) ;
#9418=CARTESIAN_POINT ( 'NONE',  ( 9.566593547379630635, -9.974457738288718289, -0.6241947029430978677 ) ) ;
#9420=CARTESIAN_POINT ( 'NONE',  ( -4.000000000000000888, -20.88361287976100300, -5.543410040383684567 ) ) ;
#9421=CARTESIAN_POINT ( 'NONE',  ( -4.243569643749997233, -24.46366198661064573, -14.92774014801135074 ) ) ;
#9422=ADVANCED_FACE ( 'NONE', ( #3011 ), #12010, .F. ) ;
#9424=CARTESIAN_POINT ( 'NONE',  ( -5.279047395330986450E-15, -25.95766108847566400, -4.737266061615885704 ) ) ;
#9426=EDGE_CURVE ( 'NONE', #17255, #18179, #1257, .T. ) ;
#9429=CARTESIAN_POINT ( 'NONE',  ( -4.000000000000002665, 2.343145750507625191, 2.343145750507618086 ) ) ;
#9430=EDGE_CURVE ( 'NONE', #8069, #2307, #14610, .T. ) ;
#9434=ORIENTED_EDGE ( 'NONE', *, *, #11755, .F. ) ;
#9438=CARTESIAN_POINT ( 'NONE',  ( 3.999999999999996447, -22.40970851469715441, -3.696582572437044245 ) ) ;
#9444=CARTESIAN_POINT ( 'NONE',  ( 2.121784821875004390, -17.58820128504952152, -7.244309707463659542 ) ) ;
#9446=( BOUNDED_CURVE ( )  B_SPLINE_CURVE ( 2, ( #8175, #18133, #10867, #5309, #12164, #7897, #17854, #16644, #1146 ),
 .UNSPECIFIED., .F., .F. ) 
 B_SPLINE_CURVE_WITH_KNOTS ( ( 3, 2, 2, 2, 3 ),
 ( 0.02586206896551724796, 0.02873563218390804558, 0.03448275862068965469, 0.04022988505747126381, 0.04310344827586207184 ),
 .UNSPECIFIED. ) 
 CURVE ( )  GEOMETRIC_REPRESENTATION_ITEM ( )  RATIONAL_B_SPLINE_CURVE ( ( 0.9330127018922194093, 0.9330127018922195203, 1.000000000000000000, 0.8660254037844387076, 1.000000000000000000, 0.8660254037844387076, 1.000000000000000000, 0.9330127018922192983, 0.9330127018922194093 ) ) 
 REPRESENTATION_ITEM ( '' )  );
#9447=CARTESIAN_POINT ( 'NONE',  ( -4.243569643750005227, -26.14381059887672976, -8.784260816366916913 ) ) ;
#9449=AXIS2_PLACEMENT_3D ( 'NONE', #12587, #16792, #16972 ) ;
#9452=CARTESIAN_POINT ( 'NONE',  ( -3.706921591972381904E-14, -18.44586024076842534, -9.035725650560502586 ) ) ;
#9454=CARTESIAN_POINT ( 'NONE',  ( 2.000000000000004441, -19.22898836077508022, -9.219838192305099156 ) ) ;
#9458=CARTESIAN_POINT ( 'NONE',  ( -5.330712181944245322E-15, -23.68761282235488963, -1.004956746021377967 ) ) ;
#9462=CARTESIAN_POINT ( 'NONE',  ( 1.999999999999994449, -27.24873388298481558, -8.594268053192397616 ) ) ;
#9467=CARTESIAN_POINT ( 'NONE',  ( -4.243569643749998122, -21.88256802303095938, -11.24155594871087338 ) ) ;
#9468=CARTESIAN_POINT ( 'NONE',  ( -4.000000000000003553, 6.938893903907228378E-15, 0.000000000000000000 ) ) ;
#9470=VERTEX_POINT ( 'NONE', #5040 ) ;
#9471=ORIENTED_EDGE ( 'NONE', *, *, #4450, .F. ) ;
#9474=LINE ( 'NONE', #6517, #13263 ) ;
#9478=CARTESIAN_POINT ( 'NONE',  ( -2.121784821875005722, -26.57729094967022831, -7.267589859493831739 ) ) ;
#9482=CARTESIAN_POINT ( 'NONE',  ( 1.533898589781675205E-14, -28.48355344591296401, -9.423462828807814162 ) ) ;
#9483=CARTESIAN_POINT ( 'NONE',  ( -5.330712181944245322E-15, -28.10773623498509721, -7.317547187323446778 ) ) ;
#9485=CARTESIAN_POINT ( 'NONE',  ( 4.150834101209824212, -27.15734369766470380, -14.50322620280942587 ) ) ;
#9489=CARTESIAN_POINT ( 'NONE',  ( -4.243569643750000786, -22.31934639735467840, -7.593850001747957990 ) ) ;
#9491=CARTESIAN_POINT ( 'NONE',  ( -2.000000000000005773, -29.61473668293285399, -11.97327023588450601 ) ) ;
#9495=CARTESIAN_POINT ( 'NONE',  ( 1.071796769724485454, -20.07057066942950385, -11.35605261078598360 ) ) ;
#9499=AXIS2_PLACEMENT_3D ( 'NONE', #14335, #7270, #12926 ) ;
#9502=CARTESIAN_POINT ( 'NONE',  ( -5.330712181944246111E-15, -25.78475166776338057, -3.999981407953017598 ) ) ;
#9504=ORIENTED_EDGE ( 'NONE', *, *, #684, .F. ) ;
#9505=DIRECTION ( 'NONE',  ( 0.000000000000000000, 0.8191520442889952403, -0.5735764363510413855 ) ) ;
#9506=CARTESIAN_POINT ( 'NONE',  ( -4.243569643750000786, -26.70720613544014199, -13.86036314055876772 ) ) ;
#9509=CARTESIAN_POINT ( 'NONE',  ( -4.000000000000000888, -22.43226925790881765, -7.755120559963970983 ) ) ;
#9511=CARTESIAN_POINT ( 'NONE',  ( -4.243569643750000786, -26.70720613544014199, -13.86036314055876772 ) ) ;
#9513=LINE ( 'NONE', #3688, #8311 ) ;
#9514=CARTESIAN_POINT ( 'NONE',  ( 4.000000000000003553, -19.42204459461930099, -7.482392114319591947 ) ) ;
#9518=CARTESIAN_POINT ( 'NONE',  ( 1.999999999999994449, -25.24838606191550028, -5.737475299741293888 ) ) ;
#9522=CARTESIAN_POINT ( 'NONE',  ( -1.661723472263481630E-14, -20.25262601527420969, -11.61605459007084029 ) ) ;
#9524=( BOUNDED_CURVE ( )  B_SPLINE_CURVE ( 2, ( #7744, #14816, #2114, #12004, #17699, #2293, #6717, #8200, #6538 ),
 .UNSPECIFIED., .F., .T. ) 
 B_SPLINE_CURVE_WITH_KNOTS ( ( 3, 2, 2, 2, 3 ),
 ( 0.04310344827586207184, 0.04597701149425287293, 0.05172413793103448204, 0.05747126436781609116, 0.06034482758620690612 ),
 .UNSPECIFIED. ) 
 CURVE ( )  GEOMETRIC_REPRESENTATION_ITEM ( )  RATIONAL_B_SPLINE_CURVE ( ( 0.9330127018922194093, 0.9330127018922194093, 1.000000000000000000, 0.8660254037844387076, 1.000000000000000000, 0.8660254037844387076, 1.000000000000000000, 0.9330127018922191873, 0.9330127018922194093 ) ) 
 REPRESENTATION_ITEM ( '' )  );
#9526=CARTESIAN_POINT ( 'NONE',  ( -2.121784821875005722, -28.93253919143669251, -10.63123294135551689 ) ) ;
#9529=CARTESIAN_POINT ( 'NONE',  ( -2.000000000000005773, -23.93632996305754190, -3.863664997423455816 ) ) ;
#9535=CARTESIAN_POINT ( 'NONE',  ( -4.243569643749998122, -18.01092707766142809, -5.712279649760158229 ) ) ;
#9537=CARTESIAN_POINT ( 'NONE',  ( -4.243569643750000786, -23.12593826097332794, -8.745782564029356720 ) ) ;
#9541=CARTESIAN_POINT ( 'NONE',  ( -4.000000000000000888, -24.56167177856700334, -10.79622252539362925 ) ) ;
#9542=CARTESIAN_POINT ( 'NONE',  ( 1.071796769724494780, -28.47202674519411758, -9.407000994151900386 ) ) ;
#9544=ORIENTED_EDGE ( 'NONE', *, *, #755, .T. ) ;
#9547=CARTESIAN_POINT ( 'NONE',  ( 2.121784821874994176, -23.69506935700625050, -3.151350836941627875 ) ) ;
#9551=UNCERTAINTY_MEASURE_WITH_UNIT (LENGTH_MEASURE( 1.000000000000000082E-05 ), #12168, 'distance_accuracy_value', 'NONE');
#9552=CARTESIAN_POINT ( 'NONE',  ( 4.000000000000003553, -22.71293939747845769, -12.18227696742093791 ) ) ;
#9553=ORIENTED_EDGE ( 'NONE', *, *, #15, .T. ) ;
#9555=CARTESIAN_POINT ( 'NONE',  ( 4.243569643750003451, -18.12922721765884049, -5.881229758894760629 ) ) ;
#9559=CARTESIAN_POINT ( 'NONE',  ( -2.000000000000005773, -27.09817006914760640, -8.379240642573305919 ) ) ;
#9560=CARTESIAN_POINT ( 'NONE',  ( -2.121784821875005722, -26.83540034602819802, -7.636208279423879475 ) ) ;
#9561=CARTESIAN_POINT ( 'NONE',  ( 4.000000000000003553, -24.26159577562626524, -14.39398748700122077 ) ) ;
#9563=CARTESIAN_POINT ( 'NONE',  ( -5.577813053751546416E-15, -26.22509622848567545, -6.198051655426662698 ) ) ;
#9565=CARTESIAN_POINT ( 'NONE',  ( 9.000000000000005329, -10.00000000000000000, 30.00000000000000000 ) ) ;
#9571=ORIENTED_EDGE ( 'NONE', *, *, #6035, .F. ) ;
#9573=CARTESIAN_POINT ( 'NONE',  ( -5.330712181944245322E-15, -28.84980074951425877, -8.377325144622332687 ) ) ;
#9578=AXIS2_PLACEMENT_3D ( 'NONE', #2388, #16758, #13953 ) ;
#9579=CARTESIAN_POINT ( 'NONE',  ( 2.121784821875004390, -20.71777771588989125, -11.71380804911548701 ) ) ;
#9582=CARTESIAN_POINT ( 'NONE',  ( -4.648177544792955347E-16, -29.58051838113927090, -10.99009111451728415 ) ) ;
#9584=CARTESIAN_POINT ( 'NONE',  ( -5.330712181944245322E-15, -25.75248799321863657, -3.953904105461760743 ) ) ;
#9594=ADVANCED_FACE ( 'NONE', ( #1090 ), #5250, .F. ) ;
#9597=CARTESIAN_POINT ( 'NONE',  ( 2.121784821874994176, -25.01788001334084299, -5.040520239083123855 ) ) ;
#9602=CARTESIAN_POINT ( 'NONE',  ( 2.000000000000004441, -18.90635161462267178, -8.759065166385774148 ) ) ;
#9603=EDGE_CURVE ( 'NONE', #9076, #4809, #7888, .T. ) ;
#9608=CARTESIAN_POINT ( 'NONE',  ( 2.121784821875004390, -23.52471740128279620, -15.72253336585475658 ) ) ;
#9610=CARTESIAN_POINT ( 'NONE',  ( -14.99999999999999645, -10.00000000000000000, 30.00000000000000000 ) ) ;
#9611=CARTESIAN_POINT ( 'NONE',  ( -1.999999999999996225, -19.18597012804874069, -9.158401788983423941 ) ) ;
#9613=ORIENTED_EDGE ( 'NONE', *, *, #3658, .F. ) ;
#9614=CARTESIAN_POINT ( 'NONE',  ( -5.577813053751546416E-15, -24.35380310418546657, -3.525568109927051275 ) ) ;
#9619=CARTESIAN_POINT ( 'NONE',  ( -4.243569643750004339, -27.95057637338251411, -11.36458975587725106 ) ) ;
#9621=CARTESIAN_POINT ( 'NONE',  ( 4.713407268011036227E-15, -16.39031081355672725, -7.178945465000852622 ) ) ;
#9624=FACE_OUTER_BOUND ( 'NONE', #12758, .T. ) ;
#9625=DIRECTION ( 'NONE',  ( -0.000000000000000000, 1.000000000000000000, -0.000000000000000000 ) ) ;
#9626=CARTESIAN_POINT ( 'NONE',  ( 4.730628863548789710E-15, -18.91846847603547133, -11.27987320052540809 ) ) ;
#9628=CARTESIAN_POINT ( 'NONE',  ( -2.908121172428787649, -29.32336267363790938, -12.73959420715949875 ) ) ;
#9630=CARTESIAN_POINT ( 'NONE',  ( -5.279047395330986450E-15, -28.28064565569737709, -8.054831840986315328 ) ) ;
#9633=ORIENTED_EDGE ( 'NONE', *, *, #9909, .T. ) ;
#9636=CARTESIAN_POINT ( 'NONE',  ( -4.243569643749997233, -18.01092707766142809, -5.712279649760157341 ) ) ;
#9640=CARTESIAN_POINT ( 'NONE',  ( 4.713407268011036227E-15, -20.77817055164219084, -13.44545860381166413 ) ) ;
#9642=CARTESIAN_POINT ( 'NONE',  ( -4.243569643750000786, -19.77051610831973605, -3.953743104938735708 ) ) ;
#9644=CARTESIAN_POINT ( 'NONE',  ( 4.730628863548789710E-15, -18.88620480149072023, -11.23379589803414902 ) ) ;
#9646=CARTESIAN_POINT ( 'NONE',  ( 4.299564228933482956E-15, -23.15635672500629738, -15.76301181529063733 ) ) ;
#9650=ORIENTED_EDGE ( 'NONE', *, *, #14664, .F. ) ;
#9654=CYLINDRICAL_SURFACE ( 'NONE', #2343, 4.000000000000000000 ) ;
#9658=CARTESIAN_POINT ( 'NONE',  ( 4.243569643749996345, -26.54172925159527452, -9.352547547092401103 ) ) ;
#9662=LINE ( 'NONE', #13939, #1307 ) ;
#9664=DIRECTION ( 'NONE',  ( -0.000000000000000000, 1.000000000000000000, -0.000000000000000000 ) ) ;
#9666=CARTESIAN_POINT ( 'NONE',  ( -2.121784821875005722, -27.12577341693091171, -8.050904001845182734 ) ) ;
#9667=CARTESIAN_POINT ( 'NONE',  ( -1.794514420735399352, -10.00000000000000178, -12.33839425357257902 ) ) ;
#9668=CARTESIAN_POINT ( 'NONE',  ( -4.000000000000004441, -22.56027232994424025, -3.911609985069677276 ) ) ;
#9671=CARTESIAN_POINT ( 'NONE',  ( -4.243569643750005227, -23.53045296075229942, -5.051999314575184030 ) ) ;
#9672=CARTESIAN_POINT ( 'NONE',  ( -4.000000000000004441, -23.85081931173408165, -5.754702084719914623 ) ) ;
#9677=CARTESIAN_POINT ( 'NONE',  ( -4.000000000000000888, -25.27147261784647014, -11.80992317919449519 ) ) ;
#9680=CARTESIAN_POINT ( 'NONE',  ( -4.243569643750000786, -21.83539127918348299, -6.902690464379118040 ) ) ;
#9685=CARTESIAN_POINT ( 'NONE',  ( 4.730628863548789710E-15, -22.49973635050228538, -16.39445377705482088 ) ) ;
#9689=CARTESIAN_POINT ( 'NONE',  ( -2.121784821874996396, -22.70737097948255823, -14.55524170274294171 ) ) ;
#9692=CARTESIAN_POINT ( 'NONE',  ( 1.999999999999994449, -24.99027666555753413, -5.368856879811245264 ) ) ;
#9699=CARTESIAN_POINT ( 'NONE',  ( -5.577813053751546416E-15, -23.57947491511155036, -2.419712850136908511 ) ) ;
#9703=CARTESIAN_POINT ( 'NONE',  ( -4.243569643749998122, -23.20537867936554832, -13.13072535085236936 ) ) ;
#9705=CARTESIAN_POINT ( 'NONE',  ( 4.000000000000003553, -18.06697026303502085, -5.547145408680076883 ) ) ;
#9708=CARTESIAN_POINT ( 'NONE',  ( -5.577813053751546416E-15, -24.87002189690140241, -4.262804949787145858 ) ) ;
#9713=CARTESIAN_POINT ( 'NONE',  ( -2.121784821875005722, -25.57711703878310061, -5.839193482264897206 ) ) ;
#9717=CARTESIAN_POINT ( 'NONE',  ( 3.999999999999996447, -26.86209560257706030, -10.05525031723713347 ) ) ;
#9718=CARTESIAN_POINT ( 'NONE',  ( 1.999999999999994449, -28.02306207205872113, -9.700123312982540824 ) ) ;
#9721=ORIENTED_EDGE ( 'NONE', *, *, #5518, .F. ) ;
#9728=CARTESIAN_POINT ( 'NONE',  ( 1.999999999999994449, -28.34569881821112602, -10.16089633890186761 ) ) ;
#9732=CARTESIAN_POINT ( 'NONE',  ( 2.000000000000004441, -22.26177376727626367, -13.55110462547639472 ) ) ;
#9734=CARTESIAN_POINT ( 'NONE',  ( -2.121784821875005722, -22.99602307520341427, -2.153009282964420290 ) ) ;
#9738=CARTESIAN_POINT ( 'NONE',  ( -4.243569643750004339, -24.82099994254214081, -6.895091414225420934 ) ) ;
#9740=CARTESIAN_POINT ( 'NONE',  ( 3.999999999999996447, -26.28134946006668926, -9.225858871387760729 ) ) ;
#9742=CARTESIAN_POINT ( 'NONE',  ( -1.661723472263481630E-14, -20.05904396871067874, -11.33959077613006450 ) ) ;
#9744=ORIENTED_EDGE ( 'NONE', *, *, #13683, .T. ) ;
#9747=CARTESIAN_POINT ( 'NONE',  ( -4.000000000000000888, -24.49714442877256459, -10.70406791940435198 ) ) ;
#9748=DIRECTION ( 'NONE',  ( 0.000000000000000000, 0.8191520442889952403, -0.5735764363510413855 ) ) ;
#9749=ORIENTED_EDGE ( 'NONE', *, *, #2592, .F. ) ;
#9752=CARTESIAN_POINT ( 'NONE',  ( 2.121784821875004390, -19.91118585227123816, -10.56187548683408828 ) ) ;
#9754=AXIS2_PLACEMENT_3D ( 'NONE', #4227, #2578, #13779 ) ;
#9756=CARTESIAN_POINT ( 'NONE',  ( -4.000000000000000888, -21.20624962591340790, -6.004183066303009575 ) ) ;
#9758=CARTESIAN_POINT ( 'NONE',  ( -4.243569643749997233, -21.39861290485977463, -10.55039641134203521 ) ) ;
#9760=ADVANCED_FACE ( 'NONE', ( #11433 ), #15586, .F. ) ;
#9761=CARTESIAN_POINT ( 'NONE',  ( 1.071796769724493670, -23.68410221844107610, -16.51671048980665191 ) ) ;
#9762=EDGE_CURVE ( 'NONE', #13448, #11075, #2840, .T. ) ;
#9763=VECTOR ( 'NONE', #5134, 1000.000000000000000 ) ;
#9765=CARTESIAN_POINT ( 'NONE',  ( 4.299564228933482956E-15, -19.28471577963676964, -10.23373551633992129 ) ) ;
#9766=CARTESIAN_POINT ( 'NONE',  ( 4.243569643749996345, -23.70252589165761492, -5.297744927861876896 ) ) ;
#9768=FACE_OUTER_BOUND ( 'NONE', #4553, .T. ) ;
#9773=LINE ( 'NONE', #10389, #2175 ) ;
#9775=CARTESIAN_POINT ( 'NONE',  ( 3.064181913176682759, -21.66367673124435100, -2.174801284911689336 ) ) ;
#9777=CARTESIAN_POINT ( 'NONE',  ( 4.243569643750003451, -19.93599299216462128, -8.461558698405095669 ) ) ;
#9781=DIRECTION ( 'NONE',  ( -0.000000000000000000, 1.000000000000000000, -0.000000000000000000 ) ) ;
#9783=CARTESIAN_POINT ( 'NONE',  ( 3.082316921986471225, -29.06618978543598786, -12.78463801463987437 ) ) ;
#9784=CARTESIAN_POINT ( 'NONE',  ( 4.243569643749996345, -28.60660442245902146, -12.30149490653278121 ) ) ;
#9787=CARTESIAN_POINT ( 'NONE',  ( 4.713407268011036227E-15, -18.00349454149897355, -9.482810590570412757 ) ) ;
#9788=VECTOR ( 'NONE', #17632, 1000.000000000000000 ) ;
#9791=( BOUNDED_CURVE ( )  B_SPLINE_CURVE ( 2, ( #8521, #6093, #4272, #14194, #2039, #7662, #7040, #1497, #12704 ),
 .UNSPECIFIED., .F., .T. ) 
 B_SPLINE_CURVE_WITH_KNOTS ( ( 3, 2, 2, 2, 3 ),
 ( 0.9396551724137931494, 0.9425287356321838672, 0.9482758620689655249, 0.9540229885057470716, 0.9568965517241379004 ),
 .UNSPECIFIED. ) 
 CURVE ( )  GEOMETRIC_REPRESENTATION_ITEM ( )  RATIONAL_B_SPLINE_CURVE ( ( 0.9330127018922194093, 0.9330127018922206306, 1.000000000000000000, 0.8660254037844387076, 1.000000000000000000, 0.8660254037844387076, 1.000000000000000000, 0.9330127018922194093, 0.9330127018922194093 ) ) 
 REPRESENTATION_ITEM ( '' )  );
#9792=CARTESIAN_POINT ( 'NONE',  ( -1.999999999999996225, -19.44407952440671039, -9.527020208913473454 ) ) ;
#9797=EDGE_LOOP ( 'NONE', ( #7403, #18348, #7015, #1479 ) ) ;
#9798=CARTESIAN_POINT ( 'NONE',  ( -4.243569643750004339, -26.91813878795063530, -9.890116076157061897 ) ) ;
#9801=VERTEX_POINT ( 'NONE', #15369 ) ;
#9802=CARTESIAN_POINT ( 'NONE',  ( 0.000000000000000000, 5.977523610840987267, 32.81826849749789687 ) ) ;
#9804=CARTESIAN_POINT ( 'NONE',  ( 9.000000000000005329, -10.00000000000000000, 30.00000000000000000 ) ) ;
#9806=CARTESIAN_POINT ( 'NONE',  ( 2.121784821875004390, -19.16912133774208016, -9.502097529535200593 ) ) ;
#9810=CARTESIAN_POINT ( 'NONE',  ( 4.713407268011036227E-15, -20.58458850507865989, -13.16899478987089189 ) ) ;
#9812=DIRECTION ( 'NONE',  ( 0.000000000000000000, 1.000000000000000000, 0.000000000000000000 ) ) ;
#9815=CARTESIAN_POINT ( 'NONE',  ( -2.000000000000005773, -28.38871705093744779, -10.22233274222354460 ) ) ;
#9818=CARTESIAN_POINT ( 'NONE',  ( 4.713407268011036227E-15, -19.74573296621031915, -11.97098492409147319 ) ) ;
#9821=LINE ( 'NONE', #12788, #18031 ) ;
#9826=CARTESIAN_POINT ( 'NONE',  ( 4.243569643750003451, -20.93616690305174544, -9.889955075634029313 ) ) ;
#9829=EDGE_CURVE ( 'NONE', #14557, #5353, #5707, .T. ) ;
#9830=DIRECTION ( 'NONE',  ( -0.000000000000000000, -0.5735764363510414965, -0.8191520442889950182 ) ) ;
#9831=DIRECTION ( 'NONE',  ( -0.000000000000000000, 1.000000000000000000, -0.000000000000000000 ) ) ;
#9832=EDGE_LOOP ( 'NONE', ( #17262, #14145, #13954, #4339 ) ) ;
#9835=DIRECTION ( 'NONE',  ( 0.000000000000000000, 0.000000000000000000, -1.000000000000000000 ) ) ;
#9838=CARTESIAN_POINT ( 'NONE',  ( -1.999999999999996225, -24.09004865885014723, -16.16215176765433270 ) ) ;
#9842=CARTESIAN_POINT ( 'NONE',  ( -5.330712181944245322E-15, -26.52681618229254212, -5.059759365251903951 ) ) ;
#9848=CARTESIAN_POINT ( 'NONE',  ( -5.330712181944245322E-15, -28.62395502770104017, -8.054784027183542250 ) ) ;
#9851=CARTESIAN_POINT ( 'NONE',  ( 0.9964672492349638810, -9.999999999997456257, -3.740800554891051899 ) ) ;
#9852=CARTESIAN_POINT ( 'NONE',  ( -3.706921591972381904E-14, -17.47795000513098884, -7.653406576829588026 ) ) ;
#9854=CARTESIAN_POINT ( 'NONE',  ( -4.243569643750005227, -21.98179658260448832, -2.840288794994898058 ) ) ;
#9858=CARTESIAN_POINT ( 'NONE',  ( 4.243569643749996345, -28.34849502610105176, -11.93287648660273703 ) ) ;
#9861=CARTESIAN_POINT ( 'NONE',  ( -9.670852723135475060, -9.962926482346835755, 0.1910560633138593534 ) ) ;
#9862=ADVANCED_FACE ( 'NONE', ( #4402 ), #15817, .F. ) ;
#9864=CARTESIAN_POINT ( 'NONE',  ( 3.250767888004682415, -21.90484815091188509, -2.246271217071878379 ) ) ;
#9867=CARTESIAN_POINT ( 'NONE',  ( 4.243569643750000786, -25.80382324818726048, -12.57019867080359710 ) ) ;
#9870=CARTESIAN_POINT ( 'NONE',  ( 4.299564228933482956E-15, -19.22018842984233089, -10.14158091035064579 ) ) ;
#9872=CARTESIAN_POINT ( 'NONE',  ( 2.121784821874994176, -27.56671030237578179, -8.680627135892345692 ) ) ;
#9873=VERTEX_POINT ( 'NONE', #15720 ) ;
#9875=CARTESIAN_POINT ( 'NONE',  ( -1.999999999999996225, -17.63731374990092959, -6.946691269403138413 ) ) ;
#9878=CARTESIAN_POINT ( 'NONE',  ( 4.299564228933482956E-15, -19.02660638327880349, -9.865117096409875330 ) ) ;
#9880=EDGE_CURVE ( 'NONE', #17896, #8888, #333, .T. ) ;
#9885=ORIENTED_EDGE ( 'NONE', *, *, #1672, .T. ) ;
#9886=CARTESIAN_POINT ( 'NONE',  ( -2.121784821874996396, -21.19097827587949467, -12.38960848565391260 ) ) ;
#9889=CYLINDRICAL_SURFACE ( 'NONE', #14603, 4.000000000000000000 ) ;
#9891=CARTESIAN_POINT ( 'NONE',  ( 4.000000000000000888, -22.04510516337187198, -7.202192930068894938 ) ) ;
#9893=( BOUNDED_CURVE ( )  B_SPLINE_CURVE ( 2, ( #3229, #72, #5727, #14542, #11736, #11367, #17146, #12945, #8767 ),
 .UNSPECIFIED., .F., .T. ) 
 B_SPLINE_CURVE_WITH_KNOTS ( ( 3, 2, 2, 2, 3 ),
 ( 0.9224137931034482873, 0.9252873563218391162, 0.9310344827586206629, 0.9367816091954023205, 0.9396551724137931494 ),
 .UNSPECIFIED. ) 
 CURVE ( )  GEOMETRIC_REPRESENTATION_ITEM ( )  RATIONAL_B_SPLINE_CURVE ( ( 0.9330127018922194093, 0.9330127018922194093, 1.000000000000000000, 0.8660254037844387076, 1.000000000000000000, 0.8660254037844387076, 1.000000000000000000, 0.9330127018922180770, 0.9330127018922194093 ) ) 
 REPRESENTATION_ITEM ( '' )  );
#9894=CARTESIAN_POINT ( 'NONE',  ( 4.730628863548789710E-15, -18.66035907967750163, -10.91125478059535681 ) ) ;
#9897=ORIENTED_EDGE ( 'NONE', *, *, #12881, .F. ) ;
#9898=CARTESIAN_POINT ( 'NONE',  ( 1.999999999999994449, -26.79704244006331493, -7.949185819321580304 ) ) ;
#9899=DIRECTION ( 'NONE',  ( -0.000000000000000000, -0.5735764363510414965, -0.8191520442889950182 ) ) ;
#9904=CARTESIAN_POINT ( 'NONE',  ( 1.999999999999994449, -28.86191761092706187, -10.89813317876196308 ) ) ;
#9907=CARTESIAN_POINT ( 'NONE',  ( 2.000000000000004441, -21.22933618184438842, -12.07663094575620377 ) ) ;
#9909=EDGE_CURVE ( 'NONE', #17255, #4281, #14522, .T. ) ;
#9912=CARTESIAN_POINT ( 'NONE',  ( 9.670609637961767646, -9.962952946793892650, 0.1891778739417505906 ) ) ;
#9913=CARTESIAN_POINT ( 'NONE',  ( 4.730628863548789710E-15, -18.62809540513275053, -10.86517747810410128 ) ) ;
#9915=CARTESIAN_POINT ( 'NONE',  ( -2.000000000000005773, -26.32384188007369730, -7.273385382783162711 ) ) ;
#9917=ORIENTED_EDGE ( 'NONE', *, *, #10393, .F. ) ;
#9923=CARTESIAN_POINT ( 'NONE',  ( 4.000000000000000888, -22.88396070224021273, -8.400202795848317194 ) ) ;
#9926=CARTESIAN_POINT ( 'NONE',  ( 4.243569643750000786, -22.96461988824960443, -8.515396051573073777 ) ) ;
#9927=( BOUNDED_CURVE ( )  B_SPLINE_CURVE ( 1, ( #988, #12188 ),
 .UNSPECIFIED., .F., .T. ) 
 B_SPLINE_CURVE_WITH_KNOTS ( ( 2, 2 ),
 ( 0.000000000000000000, 1.000000000000000000 ),
 .UNSPECIFIED. ) 
 CURVE ( )  GEOMETRIC_REPRESENTATION_ITEM ( )  RATIONAL_B_SPLINE_CURVE ( ( 0.9401540970596700131, 0.9401540970596700131 ) ) 
 REPRESENTATION_ITEM ( '' )  );
#9934=ADVANCED_FACE ( 'NONE', ( #6254 ), #7637, .F. ) ;
#9935=CARTESIAN_POINT ( 'NONE',  ( -2.121784821875005722, -25.57711703878310061, -5.839193482264897206 ) ) ;
#9936=CIRCLE ( 'NONE', #12308, 4.000000000000000000 ) ;
#9939=CARTESIAN_POINT ( 'NONE',  ( -4.000000000000004441, -22.81838172630220640, -4.280228404999725456 ) ) ;
#9940=CARTESIAN_POINT ( 'NONE',  ( 4.243569643749996345, -22.41197890986777352, -3.454652828211636884 ) ) ;
#9945=CARTESIAN_POINT ( 'NONE',  ( 4.243569643750003451, -24.80780784842128028, -15.41923137458474535 ) ) ;
#9950=CARTESIAN_POINT ( 'NONE',  ( 4.243569643750003451, -18.38733661401680308, -6.249848178824808365 ) ) ;
#9954=CARTESIAN_POINT ( 'NONE',  ( -2.121784821874996396, -22.44926158312459208, -14.18662328281289398 ) ) ;
#9958=CARTESIAN_POINT ( 'NONE',  ( -4.243569643750005227, -26.36965632068995191, -9.106801933805707350 ) ) ;
#9959=B_SPLINE_CURVE_WITH_KNOTS ( 'NONE', 3,
 ( #14952, #2245, #934, #665, #6489, #13529, #4914, #10566, #6577, #12135, #17828, #5093, #10751, #16426, #13990, #9628, #12412, #2517 ),
 .UNSPECIFIED., .F., .F.,
 ( 4, 2, 2, 2, 2, 2, 2, 2, 4 ),
 ( 0.000000000000000000, 0.0009265903667615439090, 0.001853180733523087818, 0.002779771100284632052, 0.003706361467046175636, 0.004632951833807719653, 0.005559542200569264105, 0.006486132567330806821, 0.007412722934092349537 ),
 .UNSPECIFIED. ) ;
#9961=CARTESIAN_POINT ( 'NONE',  ( -1.999999999999996225, -17.12109495718499375, -6.209454429543042941 ) ) ;
#9964=CYLINDRICAL_SURFACE ( 'NONE', #14293, 4.000000000000000000 ) ;
#9969=CARTESIAN_POINT ( 'NONE',  ( 4.243569643750003451, -21.74275876667040208, -11.04188763791542982 ) ) ;
#9971=ORIENTED_EDGE ( 'NONE', *, *, #3663, .T. ) ;
#9973=CARTESIAN_POINT ( 'NONE',  ( 1.071796769724485232, -26.14904217797241515, -6.089435214781468986 ) ) ;
#9974=ADVANCED_FACE ( 'NONE', ( #6063 ), #11716, .F. ) ;
#9980=CARTESIAN_POINT ( 'NONE',  ( -2.121784821875005722, -24.02846066063528596, -3.627482962684610346 ) ) ;
#9982=ADVANCED_FACE ( 'NONE', ( #7264 ), #5881, .F. ) ;
#9984=VERTEX_POINT ( 'NONE', #14421 ) ;
#9987=CARTESIAN_POINT ( 'NONE',  ( -1.071796769724496334, -29.01129893934772852, -10.17716150332382696 ) ) ;
#9996=CARTESIAN_POINT ( 'NONE',  ( 4.000000000000000888, -24.10998033423561893, -10.15114028950927683 ) ) ;
#9998=EDGE_CURVE ( 'NONE', #6301, #14557, #1855, .T. ) ;
#9999=CARTESIAN_POINT ( 'NONE',  ( -3.706921591972381904E-14, -17.47795000513098884, -7.653406576829588026 ) ) ;
#10001=( BOUNDED_SURFACE ( )  B_SPLINE_SURFACE ( 1, 2, ( 
 ( #8538, #12896, #11597, #3085, #14391, #1697, #305, #5947, #17294, #7427, #4561, #3178, #13085, #16343, #10491, #17381, #16164, #8912, #3275, #14589, #10581, #9012, #10396, #11690, #7800, #14779, #4842, #4647, #4928, #6414, #2076, #10299, #15979, #1893, #588, #7524, #13178, #9283, #3457, #9100, #2170, #6230, #7706, #489, #6132, #11783, #13457, #17666, #2258, #11974, #17478, #16257, #11878, #13271, #16074, #4747, #3548, #17573, #3636, #769, #10673, #14963, #13366, #9193, #3368, #14874, #14688, #5018, #680, #12059, #17756, #6326, #7883, #13542, #6040, #1985, #7611, #13729, #16718, #10945, #12150, #12240, #18209, #13635, #9368, #17841, #6503, #18020, #15414, #1225, #4079, #15045, #6594, #2618, #17929, #13822, #16630, #1039, #9732, #11036, #6679, #8158, #16529, #5106, #3993, #5474, #5292, #2710, #8341, #13915, #857, #16440, #3903, #10765, #6767, #3718, #8258, #11120, #2350, #5201, #12332, #9552, #15230, #9640, #7981, #16808, #948, #10852, #2529, #3807, #9462, #15135, #1132, #2438, #8068, #12424, #18117, #5385, #15318, #6860, #12517, #5563, #6948, #14090, #9996, #2969, #9907, #15579, #10180, #12785, #15857, #14185, #1401, #2796, #14369, #4265, #8427, #5745, #2879, #8511, #1489, #11569, #1315, #3062, #4176, #5923, #93, #12600, #11385, #16899, #11210, #9818, #12966, #8601, #8694, #11477, #7033, #1670, #7217, #15501, #18291, #12695, #2, #5653, #11295, #16989, #14003, #7124, #7304, #17074, #4538, #4347, #15761, #15670, #14277, #1582, #12872, #179, #5829, #280, #17168, #3154, #4442, #10083, #17264, #14662, #13154, #566, #6206, #11854, #10554, #6015, #4819, #465, #6300, #10371, #10468, #14472, #17454, #6393, #16145, #8989, #16229, #6108, #16323, #3524, #13062, #14851, #9171, #17728, #11667, #373, #13345, #1866, #17551, #4721, #1772, #748, #3434, #1961, #17360, #17646, #13246, #12036, #4904, #14566, #16051, #9075, #8887, #7587, #7683, #7496, #14754, #4996, #15955, #2144, #10651, #3342, #11759, #2054, #656, #11953, #7774, #13435, #8788, #7402, #4625, #10272, #3249, #17907, #5451, #3610, #9258, #6839, #13799, #15024, #1107, #13611, #2596, #2414, #8138, #6747, #3880, #11098, #9529, #14944, #6660, #2236, #16506, #12403, #13706, #7862, #2324, #8229, #16416, #12127, #13520, #834, #8045, #18182, #3970, #12490, #17821, #9346, #5365, #7955, #16606, #1020, #3785, #6476, #18094, #9438, #10925, #925, #5083, #11012, #13892, #12309, #10742, #3699, #16691, #6568, #12219, #17999, #5175, #15208, #10831, #9621, #1203, #15111, #5270, #2510, #15297, #10133, #8840, #7544, #3295, #9705, #4054, #15813, #7173, #15389, #135, #11526, #11429, #8934, #14234, #14615, #230 ),
 ( #3200, #1624, #3016, #2689, #423, #7356, #3110, #8320, #15903, #17406, #13016, #1537, #12832, #5787, #17218, #17120, #4399, #1916, #8740, #1721, #13110, #4490, #329, #10039, #15716, #8650, #6060, #10225, #13199, #4580, #14327, #14517, #14415, #5879, #7258, #12918, #1816, #5965, #514, #11712, #6158, #16785, #11621, #7451, #17314, #4669, #10322, #16002, #977, #17686, #16180, #3569, #9218, #14896, #13564, #9029, #7820, #3477, #9304, #13387, #13476, #17503, #2098, #9389, #788, #11992, #881, #9122, #11806, #6524, #16099, #17865, #12176, #2374, #14708, #3390, #16371, #4863, #2194, #7726, #4767, #3741, #6435, #4948, #2005, #2279, #16280, #15069, #7908, #17599, #702, #12081, #11900, #10604, #10697, #10512, #17781, #8002, #607, #5131, #13658, #6350, #14801, #5041, #3657, #14980, #10785, #16459, #10418, #7633, #13297, #6251, #5412, #2554, #8448, #6622, #12266, #9848, #16837, #18048, #2821, #11062, #14119, #6798, #12354, #13756, #6971, #15258, #1066, #16744, #8185, #1155, #13844, #4201, #17951, #14031, #15159, #16925, #4019, #5224, #9666, #9483, #3836, #2466, #5593, #1251, #1339, #4107, #6700, #12630, #18231, #8094, #10876, #16557, #5321, #10974, #16653, #3927, #9579, #12449, #18319, #18145, #15524, #15342, #8368, #2642, #8283, #13941, #6884, #12542, #5499, #11237, #11146, #9758, #15439, #2735, #14304, #7149, #10022, #4371, #12994, #15697, #15882, #11503, #10111, #1605, #1796, #206, #2996, #3277, #17382, #11599, #8627, #17295, #11409, #402, #5857, #5948, #4563, #1698, #8913, #7332, #1431, #4469, #7059, #7240, #10202, #17197, #12727, #12812, #6041, #14213, #9935, #27, #5680, #15792, #15981, #7428, #4648, #15604, #118, #3179, #5770, #14393, #3086, #12898, #10300, #8817, #8720, #306, #17102, #11323, #14498, #11692, #13087, #17018, #4288, #2905, #8540, #1517, #682, #1894, #2171, #7526, #3639, #859, #492, #13273, #2078, #4930, #7708, #6415, #5109, #6506, #13179, #6133, #13367, #4748, #11784, #16076, #9102, #9013, #12153, #17480, #17843, #16165, #13544, #6328, #10398, #3369, #14689, #1987, #10583, #3550, #10492, #3458, #770, #17576, #590, #7612, #16345, #16259, #11975, #6232, #13459, #14965, #9194, #11879, #4843, #14780, #17667, #14875, #7801, #10767, #12060, #17758, #10675, #5022, #9285, #2261, #7885, #16442, #3721, #14591, #15137, #11212, #6770, #5204, #16902, #15233, #13731, #1134, #12428, #18120, #11123, #6596, #5388, #1042, #6863, #10948, #11039, #15047, #18022, #6950, #16721, #9555, #16811, #6681, #9371, #4081, #13637, #15417, #9734, #18294, #12242, #951, #13918, #2440, #3996, #5295, #2353, #1317, #9642, #2531, #17931, #18211, #13824, #12604, #5478 ) ),
 .UNSPECIFIED., .F., .F., .T. ) 
 B_SPLINE_SURFACE_WITH_KNOTS ( ( 2, 2 ),
 ( 3, 2, 2, 2, 2, 2, 2, 2, 2, 2, 2, 2, 2, 2, 2, 2, 2, 2, 2, 2, 2, 2, 2, 2, 2, 2, 2, 2, 2, 2, 2, 2, 2, 2, 2, 2, 2, 2, 2, 2, 2, 2, 2, 2, 2, 2, 2, 2, 2, 2, 2, 2, 2, 2, 2, 2, 2, 2, 2, 2, 2, 2, 2, 2, 2, 2, 2, 2, 2, 2, 2, 2, 2, 2, 2, 2, 2, 2, 2, 2, 2, 2, 2, 2, 2, 2, 2, 2, 2, 2, 2, 2, 2, 2, 2, 2, 2, 2, 2, 2, 2, 2, 2, 2, 2, 2, 2, 2, 2, 2, 2, 2, 2, 2, 2, 2, 2, 2, 2, 2, 2, 2, 2, 2, 2, 2, 2, 2, 2, 2, 2, 2, 2, 2, 2, 2, 2, 2, 2, 2, 2, 2, 2, 2, 2, 2, 2, 2, 2, 2, 2, 2, 2, 2, 2, 2, 2, 2, 2, 2, 2, 2, 2, 2, 2, 2, 2, 2, 2, 2, 2, 2, 2, 2, 3 ),
 ( 0.000000000000000000, 1.000000000000000000 ),
 ( 0.000000000000000000, 0.005747126436781609116, 0.01149425287356321823, 0.01724137931034482735, 0.02298850574712643646, 0.02873563218390804558, 0.03448275862068965469, 0.04022988505747126381, 0.04597701149425287293, 0.05172413793103448204, 0.05747126436781609116, 0.06321839080459770721, 0.06896551724137930939, 0.07471264367816092544, 0.08045977011494252762, 0.08620689655172414367, 0.09195402298850574585, 0.09770114942528736190, 0.1034482758620689641, 0.1091954022988505801, 0.1149425287356321823, 0.1206896551724137984, 0.1264367816091954144, 0.1321839080459770166, 0.1379310344827586188, 0.1436781609195402210, 0.1494252873563218509, 0.1551724137931034531, 0.1609195402298850552, 0.1666666666666666574, 0.1724137931034482873, 0.1781609195402298895, 0.1839080459770114917, 0.1896551724137930939, 0.1954022988505747238, 0.2011494252873563260, 0.2068965517241379282, 0.2126436781609195303, 0.2183908045977011603, 0.2241379310344827624, 0.2298850574712643646, 0.2356321839080459668, 0.2413793103448275967, 0.2471264367816091989, 0.2528735632183908288, 0.2586206896551724310, 0.2643678160919540332, 0.2701149425287356354, 0.2758620689655172376, 0.2816091954022988397, 0.2873563218390804419, 0.2931034482758620441, 0.2988505747126437018, 0.3045977011494253039, 0.3103448275862069061, 0.3160919540229885083, 0.3218390804597701105, 0.3275862068965517127, 0.3333333333333333148, 0.3390804597701149170, 0.3448275862068965747, 0.3505747126436781769, 0.3563218390804597790, 0.3620689655172413812, 0.3678160919540229834, 0.3735632183908045856, 0.3793103448275861878, 0.3850574712643677899, 0.3908045977011494476, 0.3965517241379310498, 0.4022988505747126520, 0.4080459770114942541, 0.4137931034482758563, 0.4195402298850574585, 0.4252873563218390607, 0.4310344827586206629, 0.4367816091954023205, 0.4425287356321839227, 0.4482758620689655249, 0.4540229885057471271, 0.4597701149425287293, 0.4655172413793103314, 0.4712643678160919336, 0.4770114942528735358, 0.4827586206896551935, 0.4885057471264367956, 0.4942528735632183978, 0.5000000000000000000, 0.5057471264367816577, 0.5114942528735632044, 0.5172413793103448620, 0.5229885057471264087, 0.5287356321839080664, 0.5344827586206896131, 0.5402298850574712707, 0.5459770114942529284, 0.5517241379310344751, 0.5574712643678161328, 0.5632183908045976795, 0.5689655172413793371, 0.5747126436781608838, 0.5804597701149425415, 0.5862068965517240882, 0.5919540229885057459, 0.5977011494252874035, 0.6034482758620689502, 0.6091954022988506079, 0.6149425287356321546, 0.6206896551724138122, 0.6264367816091953589, 0.6321839080459770166, 0.6379310344827586743, 0.6436781609195402210, 0.6494252873563218786, 0.6551724137931034253, 0.6609195402298850830, 0.6666666666666666297, 0.6724137931034482873, 0.6781609195402298340, 0.6839080459770114917, 0.6896551724137931494, 0.6954022988505746961, 0.7011494252873563537, 0.7068965517241379004, 0.7126436781609195581, 0.7183908045977011048, 0.7241379310344827624, 0.7298850574712644201, 0.7356321839080459668, 0.7413793103448276245, 0.7471264367816091712, 0.7528735632183908288, 0.7586206896551723755, 0.7643678160919540332, 0.7701149425287355799, 0.7758620689655172376, 0.7816091954022988952, 0.7873563218390804419, 0.7931034482758620996, 0.7988505747126436463, 0.8045977011494253039, 0.8103448275862068506, 0.8160919540229885083, 0.8218390804597701660, 0.8275862068965517127, 0.8333333333333333703, 0.8390804597701149170, 0.8448275862068965747, 0.8505747126436781214, 0.8563218390804597790, 0.8620689655172413257, 0.8678160919540229834, 0.8735632183908046411, 0.8793103448275861878, 0.8850574712643678454, 0.8908045977011493921, 0.8965517241379310498, 0.9022988505747125965, 0.9080459770114942541, 0.9137931034482759118, 0.9195402298850574585, 0.9252873563218391162, 0.9310344827586206629, 0.9367816091954023205, 0.9425287356321838672, 0.9482758620689655249, 0.9540229885057470716, 0.9597701149425287293, 0.9655172413793103869, 0.9712643678160919336, 0.9770114942528735913, 0.9827586206896551380, 0.9885057471264367956, 0.9942528735632183423, 0.9961881933054925753 ),
 .UNSPECIFIED. ) 
 GEOMETRIC_REPRESENTATION_ITEM ( )  RATIONAL_B_SPLINE_SURFACE ( (
 ( 1.000000000000000000, 0.8660254037844387076, 1.000000000000000000, 0.8660254037844387076, 1.000000000000000000, 0.8660254037844387076, 1.000000000000000000, 0.8660254037844387076, 1.000000000000000000, 0.8660254037844387076, 1.000000000000000000, 0.8660254037844387076, 1.000000000000000000, 0.8660254037844387076, 1.000000000000000000, 0.8660254037844387076, 1.000000000000000000, 0.8660254037844387076, 1.000000000000000000, 0.8660254037844387076, 1.000000000000000000, 0.8660254037844387076, 1.000000000000000000, 0.8660254037844387076, 1.000000000000000000, 0.8660254037844387076, 1.000000000000000000, 0.8660254037844387076, 1.000000000000000000, 0.8660254037844387076, 1.000000000000000000, 0.8660254037844387076, 1.000000000000000000, 0.8660254037844387076, 1.000000000000000000, 0.8660254037844387076, 1.000000000000000000, 0.8660254037844387076, 1.000000000000000000, 0.8660254037844387076, 1.000000000000000000, 0.8660254037844387076, 1.000000000000000000, 0.8660254037844387076, 1.000000000000000000, 0.8660254037844387076, 1.000000000000000000, 0.8660254037844387076, 1.000000000000000000, 0.8660254037844387076, 1.000000000000000000, 0.8660254037844387076, 1.000000000000000000, 0.8660254037844387076, 1.000000000000000000, 0.8660254037844387076, 1.000000000000000000, 0.8660254037844387076, 1.000000000000000000, 0.8660254037844387076, 1.000000000000000000, 0.8660254037844387076, 1.000000000000000000, 0.8660254037844387076, 1.000000000000000000, 0.8660254037844387076, 1.000000000000000000, 0.8660254037844387076, 1.000000000000000000, 0.8660254037844387076, 1.000000000000000000, 0.8660254037844387076, 1.000000000000000000, 0.8660254037844387076, 1.000000000000000000, 0.8660254037844387076, 1.000000000000000000, 0.8660254037844387076, 1.000000000000000000, 0.8660254037844387076, 1.000000000000000000, 0.8660254037844387076, 1.000000000000000000, 0.8660254037844387076, 1.000000000000000000, 0.8660254037844387076, 1.000000000000000000, 0.8660254037844387076, 1.000000000000000000, 0.8660254037844387076, 1.000000000000000000, 0.8660254037844387076, 1.000000000000000000, 0.8660254037844387076, 1.000000000000000000, 0.8660254037844387076, 1.000000000000000000, 0.8660254037844387076, 1.000000000000000000, 0.8660254037844387076, 1.000000000000000000, 0.8660254037844387076, 1.000000000000000000, 0.8660254037844387076, 1.000000000000000000, 0.8660254037844387076, 1.000000000000000000, 0.8660254037844387076, 1.000000000000000000, 0.8660254037844387076, 1.000000000000000000, 0.8660254037844387076, 1.000000000000000000, 0.8660254037844387076, 1.000000000000000000, 0.8660254037844387076, 1.000000000000000000, 0.8660254037844387076, 1.000000000000000000, 0.8660254037844387076, 1.000000000000000000, 0.8660254037844387076, 1.000000000000000000, 0.8660254037844387076, 1.000000000000000000, 0.8660254037844387076, 1.000000000000000000, 0.8660254037844387076, 1.000000000000000000, 0.8660254037844387076, 1.000000000000000000, 0.8660254037844387076, 1.000000000000000000, 0.8660254037844387076, 1.000000000000000000, 0.8660254037844387076, 1.000000000000000000, 0.8660254037844387076, 1.000000000000000000, 0.8660254037844387076, 1.000000000000000000, 0.8660254037844387076, 1.000000000000000000, 0.8660254037844387076, 1.000000000000000000, 0.8660254037844387076, 1.000000000000000000, 0.8660254037844387076, 1.000000000000000000, 0.8660254037844387076, 1.000000000000000000, 0.8660254037844387076, 1.000000000000000000, 0.8660254037844387076, 1.000000000000000000, 0.8660254037844387076, 1.000000000000000000, 0.8660254037844387076, 1.000000000000000000, 0.8660254037844387076, 1.000000000000000000, 0.8660254037844387076, 1.000000000000000000, 0.8660254037844387076, 1.000000000000000000, 0.8660254037844387076, 1.000000000000000000, 0.8660254037844387076, 1.000000000000000000, 0.8660254037844387076, 1.000000000000000000, 0.8660254037844387076, 1.000000000000000000, 0.8660254037844387076, 1.000000000000000000, 0.8660254037844387076, 1.000000000000000000, 0.8660254037844387076, 1.000000000000000000, 0.8660254037844387076, 1.000000000000000000, 0.8660254037844387076, 1.000000000000000000, 0.8660254037844387076, 1.000000000000000000, 0.8660254037844387076, 1.000000000000000000, 0.8660254037844387076, 1.000000000000000000, 0.8660254037844387076, 1.000000000000000000, 0.8660254037844387076, 1.000000000000000000, 0.8660254037844387076, 1.000000000000000000, 0.8660254037844387076, 1.000000000000000000, 0.8660254037844387076, 1.000000000000000000, 0.8660254037844387076, 1.000000000000000000, 0.8660254037844387076, 1.000000000000000000, 0.8660254037844387076, 1.000000000000000000, 0.8660254037844387076, 1.000000000000000000, 0.8660254037844387076, 1.000000000000000000, 0.8660254037844387076, 1.000000000000000000, 0.8660254037844387076, 1.000000000000000000, 0.8660254037844387076, 1.000000000000000000, 0.8660254037844387076, 1.000000000000000000, 0.8660254037844387076, 1.000000000000000000, 0.8660254037844387076, 1.000000000000000000, 0.8660254037844387076, 1.000000000000000000, 0.8660254037844387076, 1.000000000000000000, 0.8660254037844387076, 1.000000000000000000, 0.8660254037844387076, 1.000000000000000000, 0.8660254037844387076, 1.000000000000000000, 0.8660254037844387076, 1.000000000000000000, 0.8660254037844387076, 1.000000000000000000, 0.8660254037844387076, 1.000000000000000000, 0.8660254037844387076, 1.000000000000000000, 0.8660254037844387076, 1.000000000000000000, 0.8660254037844387076, 1.000000000000000000, 0.8660254037844387076, 1.000000000000000000, 0.8660254037844387076, 1.000000000000000000, 0.8660254037844387076, 1.000000000000000000, 0.8660254037844387076, 1.000000000000000000, 0.8660254037844387076, 1.000000000000000000, 0.8660254037844387076, 1.000000000000000000, 0.8660254037844387076, 1.000000000000000000, 0.8660254037844387076, 1.000000000000000000, 0.8660254037844387076, 1.000000000000000000, 0.8660254037844387076, 1.000000000000000000, 0.8660254037844387076, 1.000000000000000000, 0.8660254037844387076, 1.000000000000000000, 0.8660254037844387076, 1.000000000000000000, 0.8660254037844387076, 1.000000000000000000, 0.8660254037844387076, 1.000000000000000000, 0.8660254037844387076, 1.000000000000000000, 0.8660254037844387076, 1.000000000000000000, 0.8660254037844387076, 1.000000000000000000, 0.8660254037844387076, 1.000000000000000000, 0.8660254037844387076, 1.000000000000000000, 0.8660254037844387076, 1.000000000000000000, 0.8660254037844387076, 1.000000000000000000, 0.8660254037844387076, 1.000000000000000000, 0.8660254037844387076, 1.000000000000000000, 0.8660254037844387076, 1.000000000000000000, 0.8660254037844387076, 1.000000000000000000, 0.8660254037844387076, 1.000000000000000000, 0.8660254037844387076, 1.000000000000000000, 0.8660254037844387076, 1.000000000000000000, 0.8660254037844387076, 1.000000000000000000, 0.8660254037844387076, 1.000000000000000000, 0.8660254037844387076, 1.000000000000000000, 0.8660254037844387076, 1.000000000000000000, 0.8660254037844387076, 1.000000000000000000, 0.8660254037844387076, 1.000000000000000000, 0.8660254037844387076, 1.000000000000000000, 0.8660254037844387076, 1.000000000000000000, 0.8660254037844387076, 1.000000000000000000, 0.8660254037844387076, 1.000000000000000000, 0.8660254037844387076, 1.000000000000000000, 0.8660254037844387076, 1.000000000000000000, 0.8660254037844387076, 1.000000000000000000, 0.8660254037844387076, 1.000000000000000000, 0.8660254037844387076, 1.000000000000000000, 0.8660254037844387076, 1.000000000000000000, 0.8660254037844387076, 1.000000000000000000, 0.8660254037844387076, 1.000000000000000000, 0.8660254037844387076, 1.000000000000000000, 0.8660254037844387076, 1.000000000000000000, 0.8660254037844387076, 1.000000000000000000, 0.8660254037844387076, 1.000000000000000000, 0.8660254037844387076, 1.000000000000000000, 0.9548846395026606704, 0.9401540804572323662),
 ( 1.000000000000000000, 0.8660254037844387076, 1.000000000000000000, 0.8660254037844387076, 1.000000000000000000, 0.8660254037844387076, 1.000000000000000000, 0.8660254037844387076, 1.000000000000000000, 0.8660254037844387076, 1.000000000000000000, 0.8660254037844387076, 1.000000000000000000, 0.8660254037844387076, 1.000000000000000000, 0.8660254037844387076, 1.000000000000000000, 0.8660254037844387076, 1.000000000000000000, 0.8660254037844387076, 1.000000000000000000, 0.8660254037844387076, 1.000000000000000000, 0.8660254037844387076, 1.000000000000000000, 0.8660254037844387076, 1.000000000000000000, 0.8660254037844387076, 1.000000000000000000, 0.8660254037844387076, 1.000000000000000000, 0.8660254037844387076, 1.000000000000000000, 0.8660254037844387076, 1.000000000000000000, 0.8660254037844387076, 1.000000000000000000, 0.8660254037844387076, 1.000000000000000000, 0.8660254037844387076, 1.000000000000000000, 0.8660254037844387076, 1.000000000000000000, 0.8660254037844387076, 1.000000000000000000, 0.8660254037844387076, 1.000000000000000000, 0.8660254037844387076, 1.000000000000000000, 0.8660254037844387076, 1.000000000000000000, 0.8660254037844387076, 1.000000000000000000, 0.8660254037844387076, 1.000000000000000000, 0.8660254037844387076, 1.000000000000000000, 0.8660254037844387076, 1.000000000000000000, 0.8660254037844387076, 1.000000000000000000, 0.8660254037844387076, 1.000000000000000000, 0.8660254037844387076, 1.000000000000000000, 0.8660254037844387076, 1.000000000000000000, 0.8660254037844387076, 1.000000000000000000, 0.8660254037844387076, 1.000000000000000000, 0.8660254037844387076, 1.000000000000000000, 0.8660254037844387076, 1.000000000000000000, 0.8660254037844387076, 1.000000000000000000, 0.8660254037844387076, 1.000000000000000000, 0.8660254037844387076, 1.000000000000000000, 0.8660254037844387076, 1.000000000000000000, 0.8660254037844387076, 1.000000000000000000, 0.8660254037844387076, 1.000000000000000000, 0.8660254037844387076, 1.000000000000000000, 0.8660254037844387076, 1.000000000000000000, 0.8660254037844387076, 1.000000000000000000, 0.8660254037844387076, 1.000000000000000000, 0.8660254037844387076, 1.000000000000000000, 0.8660254037844387076, 1.000000000000000000, 0.8660254037844387076, 1.000000000000000000, 0.8660254037844387076, 1.000000000000000000, 0.8660254037844387076, 1.000000000000000000, 0.8660254037844387076, 1.000000000000000000, 0.8660254037844387076, 1.000000000000000000, 0.8660254037844387076, 1.000000000000000000, 0.8660254037844387076, 1.000000000000000000, 0.8660254037844387076, 1.000000000000000000, 0.8660254037844387076, 1.000000000000000000, 0.8660254037844387076, 1.000000000000000000, 0.8660254037844387076, 1.000000000000000000, 0.8660254037844387076, 1.000000000000000000, 0.8660254037844387076, 1.000000000000000000, 0.8660254037844387076, 1.000000000000000000, 0.8660254037844387076, 1.000000000000000000, 0.8660254037844387076, 1.000000000000000000, 0.8660254037844387076, 1.000000000000000000, 0.8660254037844387076, 1.000000000000000000, 0.8660254037844387076, 1.000000000000000000, 0.8660254037844387076, 1.000000000000000000, 0.8660254037844387076, 1.000000000000000000, 0.8660254037844387076, 1.000000000000000000, 0.8660254037844387076, 1.000000000000000000, 0.8660254037844387076, 1.000000000000000000, 0.8660254037844387076, 1.000000000000000000, 0.8660254037844387076, 1.000000000000000000, 0.8660254037844387076, 1.000000000000000000, 0.8660254037844387076, 1.000000000000000000, 0.8660254037844387076, 1.000000000000000000, 0.8660254037844387076, 1.000000000000000000, 0.8660254037844387076, 1.000000000000000000, 0.8660254037844387076, 1.000000000000000000, 0.8660254037844387076, 1.000000000000000000, 0.8660254037844387076, 1.000000000000000000, 0.8660254037844387076, 1.000000000000000000, 0.8660254037844387076, 1.000000000000000000, 0.8660254037844387076, 1.000000000000000000, 0.8660254037844387076, 1.000000000000000000, 0.8660254037844387076, 1.000000000000000000, 0.8660254037844387076, 1.000000000000000000, 0.8660254037844387076, 1.000000000000000000, 0.8660254037844387076, 1.000000000000000000, 0.8660254037844387076, 1.000000000000000000, 0.8660254037844387076, 1.000000000000000000, 0.8660254037844387076, 1.000000000000000000, 0.8660254037844387076, 1.000000000000000000, 0.8660254037844387076, 1.000000000000000000, 0.8660254037844387076, 1.000000000000000000, 0.8660254037844387076, 1.000000000000000000, 0.8660254037844387076, 1.000000000000000000, 0.8660254037844387076, 1.000000000000000000, 0.8660254037844387076, 1.000000000000000000, 0.8660254037844387076, 1.000000000000000000, 0.8660254037844387076, 1.000000000000000000, 0.8660254037844387076, 1.000000000000000000, 0.8660254037844387076, 1.000000000000000000, 0.8660254037844387076, 1.000000000000000000, 0.8660254037844387076, 1.000000000000000000, 0.8660254037844387076, 1.000000000000000000, 0.8660254037844387076, 1.000000000000000000, 0.8660254037844387076, 1.000000000000000000, 0.8660254037844387076, 1.000000000000000000, 0.8660254037844387076, 1.000000000000000000, 0.8660254037844387076, 1.000000000000000000, 0.8660254037844387076, 1.000000000000000000, 0.8660254037844387076, 1.000000000000000000, 0.8660254037844387076, 1.000000000000000000, 0.8660254037844387076, 1.000000000000000000, 0.8660254037844387076, 1.000000000000000000, 0.8660254037844387076, 1.000000000000000000, 0.8660254037844387076, 1.000000000000000000, 0.8660254037844387076, 1.000000000000000000, 0.8660254037844387076, 1.000000000000000000, 0.8660254037844387076, 1.000000000000000000, 0.8660254037844387076, 1.000000000000000000, 0.8660254037844387076, 1.000000000000000000, 0.8660254037844387076, 1.000000000000000000, 0.8660254037844387076, 1.000000000000000000, 0.8660254037844387076, 1.000000000000000000, 0.8660254037844387076, 1.000000000000000000, 0.8660254037844387076, 1.000000000000000000, 0.8660254037844387076, 1.000000000000000000, 0.8660254037844387076, 1.000000000000000000, 0.8660254037844387076, 1.000000000000000000, 0.8660254037844387076, 1.000000000000000000, 0.8660254037844387076, 1.000000000000000000, 0.8660254037844387076, 1.000000000000000000, 0.8660254037844387076, 1.000000000000000000, 0.8660254037844387076, 1.000000000000000000, 0.8660254037844387076, 1.000000000000000000, 0.8660254037844387076, 1.000000000000000000, 0.8660254037844387076, 1.000000000000000000, 0.8660254037844387076, 1.000000000000000000, 0.8660254037844387076, 1.000000000000000000, 0.8660254037844387076, 1.000000000000000000, 0.8660254037844387076, 1.000000000000000000, 0.8660254037844387076, 1.000000000000000000, 0.8660254037844387076, 1.000000000000000000, 0.8660254037844387076, 1.000000000000000000, 0.8660254037844387076, 1.000000000000000000, 0.8660254037844387076, 1.000000000000000000, 0.8660254037844387076, 1.000000000000000000, 0.8660254037844387076, 1.000000000000000000, 0.8660254037844387076, 1.000000000000000000, 0.8660254037844387076, 1.000000000000000000, 0.8660254037844387076, 1.000000000000000000, 0.8660254037844387076, 1.000000000000000000, 0.8660254037844387076, 1.000000000000000000, 0.8660254037844387076, 1.000000000000000000, 0.8660254037844387076, 1.000000000000000000, 0.8660254037844387076, 1.000000000000000000, 0.8660254037844387076, 1.000000000000000000, 0.8660254037844387076, 1.000000000000000000, 0.8660254037844387076, 1.000000000000000000, 0.8660254037844387076, 1.000000000000000000, 0.8660254037844387076, 1.000000000000000000, 0.8660254037844387076, 1.000000000000000000, 0.8660254037844387076, 1.000000000000000000, 0.8660254037844387076, 1.000000000000000000, 0.8660254037844387076, 1.000000000000000000, 0.8660254037844387076, 1.000000000000000000, 0.8660254037844387076, 1.000000000000000000, 0.8660254037844387076, 1.000000000000000000, 0.8660254037844387076, 1.000000000000000000, 0.9548846395026606704, 0.9401540804572323662) ) ) 
 REPRESENTATION_ITEM ( '' )  SURFACE ( )  );
#10002=CARTESIAN_POINT ( 'NONE',  ( -7.385235650263080487, -10.35677961432909377, 5.003020502729047969 ) ) ;
#10003=CARTESIAN_POINT ( 'NONE',  ( -4.243569643750000786, -23.09367458642858040, -8.699705261538101198 ) ) ;
#10006=CARTESIAN_POINT ( 'NONE',  ( 1.071796769724485232, -23.30983881803475555, -2.034632595550943002 ) ) ;
#10007=ORIENTED_EDGE ( 'NONE', *, *, #7265, .F. ) ;
#10011=CARTESIAN_POINT ( 'NONE',  ( 4.898587196589417759E-16, -3.999999999999993339, 25.54267522293723758 ) ) ;
#10012=CARTESIAN_POINT ( 'NONE',  ( -3.706921591972381904E-14, -18.25227819420489439, -8.759261836619732122 ) ) ;
#10016=CARTESIAN_POINT ( 'NONE',  ( -2.121784821875005722, -25.28674396788038337, -5.424497759843593059 ) ) ;
#10022=CARTESIAN_POINT ( 'NONE',  ( 2.121784821874994176, -26.30842699513068439, -6.883612338733362535 ) ) ;
#10024=CYLINDRICAL_SURFACE ( 'NONE', #12745, 4.000000000000000000 ) ;
#10026=CARTESIAN_POINT ( 'NONE',  ( 4.243569643750000786, -20.89974471738585748, -5.566448692132691001 ) ) ;
#10027=CARTESIAN_POINT ( 'NONE',  ( -8.999999999999996447, -10.00000000000000000, 30.00000000000000000 ) ) ;
#10035=FACE_OUTER_BOUND ( 'NONE', #6182, .T. ) ;
#10036=VERTEX_POINT ( 'NONE', #9485 ) ;
#10037=CARTESIAN_POINT ( 'NONE',  ( -5.330712181944246111E-15, -23.97798589325759977, -1.419652468442682558 ) ) ;
#10039=CARTESIAN_POINT ( 'NONE',  ( 4.243569643749996345, -28.63886809700377611, -12.34757220902403851 ) ) ;
#10042=CARTESIAN_POINT ( 'NONE',  ( 4.243569643749997233, -27.05794804431121037, -10.08978438695249480 ) ) ;
#10047=CARTESIAN_POINT ( 'NONE',  ( 4.243569643749996345, -27.31605744066918007, -10.45840280688254431 ) ) ;
#10048=CYLINDRICAL_SURFACE ( 'NONE', #9499, 4.000000000000000000 ) ;
#10049=CARTESIAN_POINT ( 'NONE',  ( -4.000000000000000888, -20.69003083319747205, -5.266946226442914991 ) ) ;
#10050=EDGE_CURVE ( 'NONE', #17559, #3748, #16282, .T. ) ;
#10054=CARTESIAN_POINT ( 'NONE',  ( -1.999999999999996225, -20.99273590255452149, -11.73873072849375987 ) ) ;
#10059=VERTEX_POINT ( 'NONE', #10880 ) ;
#10060=CARTESIAN_POINT ( 'NONE',  ( -2.121784821875005722, -27.64199220964684756, -8.788140841705278206 ) ) ;
#10063=ORIENTED_EDGE ( 'NONE', *, *, #13044, .F. ) ;
#10065=FACE_OUTER_BOUND ( 'NONE', #7952, .T. ) ;
#10067=CARTESIAN_POINT ( 'NONE',  ( 3.157473464924626771, -21.86492304994214564, -2.325728555794866814 ) ) ;
#10068=CARTESIAN_POINT ( 'NONE',  ( 3.579096709490575479E-14, -23.83758431146952361, -2.788331270066955359 ) ) ;
#10069=CARTESIAN_POINT ( 'NONE',  ( 2.121784821874994176, -24.24355182426693389, -3.934664979292979314 ) ) ;
#10076=CARTESIAN_POINT ( 'NONE',  ( 3.999999999999993339, 0.000000000000000000, 30.00000000000000000 ) ) ;
#10081=ORIENTED_EDGE ( 'NONE', *, *, #15287, .T. ) ;
#10083=CARTESIAN_POINT ( 'NONE',  ( 3.999999999999996447, -24.73269308191887461, -7.014148351807475201 ) ) ;
#10084=EDGE_LOOP ( 'NONE', ( #3786, #7719, #17961, #1133 ) ) ;
#10085=DIRECTION ( 'NONE',  ( -0.000000000000000000, -0.5735764363510414965, -0.8191520442889950182 ) ) ;
#10087=CARTESIAN_POINT ( 'NONE',  ( 10.00265829479232060, -9.915630618149643638, 6.507612919863985823 ) ) ;
#10088=CARTESIAN_POINT ( 'NONE',  ( -4.243569643750004339, -24.04667175346823527, -5.789236154435278614 ) ) ;
#10090=CARTESIAN_POINT ( 'NONE',  ( 2.000000000000004441, -17.09958584011689098, -6.178736226875440884 ) ) ;
#10096=CARTESIAN_POINT ( 'NONE',  ( 1.071796769724504328, -24.40680375326105533, -3.601260881260418767 ) ) ;
#10097=CARTESIAN_POINT ( 'NONE',  ( -1.999999999999996225, -23.76741191269774234, -15.70137874173500947 ) ) ;
#10098=ORIENTED_EDGE ( 'NONE', *, *, #18188, .T. ) ;
#10100=CARTESIAN_POINT ( 'NONE',  ( 4.000000000000003553, -23.80990433270476458, -13.74890525313040612 ) ) ;
#10101=CARTESIAN_POINT ( 'NONE',  ( 4.243569643749996345, -25.50929166616339572, -7.878073867372210159 ) ) ;
#10103=ADVANCED_FACE ( 'NONE', ( #5226 ), #2281, .F. ) ;
#10110=( BOUNDED_CURVE ( )  B_SPLINE_CURVE ( 3, ( #1180, #5432, #11078, #6726 ),
 .UNSPECIFIED., .F., .F. ) 
 B_SPLINE_CURVE_WITH_KNOTS ( ( 4, 4 ),
 ( 3.141592653589793116, 4.171289454427542509 ),
 .UNSPECIFIED. ) 
 CURVE ( )  GEOMETRIC_REPRESENTATION_ITEM ( )  RATIONAL_B_SPLINE_CURVE ( ( 1.000000000000000000, 0.9135782535825738293, 0.9135782535825738293, 1.000000000000000000 ) ) 
 REPRESENTATION_ITEM ( '' )  );
#10111=CARTESIAN_POINT ( 'NONE',  ( -2.121784821874996396, -20.15854069044762298, -10.91513480593371987 ) ) ;
#10112=CARTESIAN_POINT ( 'NONE',  ( -6.428571428571423496, -11.73421655796351892, 14.25837509840161310 ) ) ;
#10117=CYLINDRICAL_SURFACE ( 'NONE', #6461, 4.000000000000000000 ) ;
#10118=CARTESIAN_POINT ( 'NONE',  ( 4.730628863548789710E-15, -16.04700144155306774, -7.178993278803624811 ) ) ;
#10120=CARTESIAN_POINT ( 'NONE',  ( -5.577813053751546416E-15, -23.90211166126395881, -2.880485876056233518 ) ) ;
#10124=CARTESIAN_POINT ( 'NONE',  ( -3.999999999999997335, -20.30391836480407619, -8.741838381407161407 ) ) ;
#10125=LINE ( 'NONE', #8926, #7452 ) ;
#10128=ORIENTED_EDGE ( 'NONE', *, *, #62, .T. ) ;
#10130=CARTESIAN_POINT ( 'NONE',  ( -2.121784821875005722, -22.73791367884544812, -1.784390863034371666 ) ) ;
#10133=CARTESIAN_POINT ( 'NONE',  ( -5.279047395330986450E-15, -23.82825856781747831, -1.696164096186225656 ) ) ;
#10135=CARTESIAN_POINT ( 'NONE',  ( -4.243569643750004339, -27.14398450976385746, -10.21265719359585056 ) ) ;
#10136=CARTESIAN_POINT ( 'NONE',  ( 0.000000000000000000, 9.254131787996968228, 30.52396275209373044 ) ) ;
#10139=CARTESIAN_POINT ( 'NONE',  ( -2.121784821874996396, -21.41682399769271328, -12.71214960309270303 ) ) ;
#10141=VECTOR ( 'NONE', #4966, 1000.000000000000000 ) ;
#10142=CARTESIAN_POINT ( 'NONE',  ( -3.999999999999997335, -18.56167994009273059, -6.253664047886104527 ) ) ;
#10143=AXIS2_PLACEMENT_3D ( 'NONE', #6758, #2521, #3709 ) ;
#10144=EDGE_CURVE ( 'NONE', #4809, #10036, #15438, .T. ) ;
#10148=FACE_OUTER_BOUND ( 'NONE', #6070, .T. ) ;
#10150=CARTESIAN_POINT ( 'NONE',  ( -2.000000000000005773, -25.80762308735776145, -6.536148542923068128 ) ) ;
#10153=ORIENTED_EDGE ( 'NONE', *, *, #5808, .T. ) ;
#10154=CARTESIAN_POINT ( 'NONE',  ( 4.243569643750003451, -22.00086816302836823, -11.41050605784547578 ) ) ;
#10158=AXIS2_PLACEMENT_3D ( 'NONE', #15452, #12741, #1715 ) ;
#10161=CARTESIAN_POINT ( 'NONE',  ( 4.243569643750000786, -25.57797752637403832, -12.24765755336480666 ) ) ;
#10162=CARTESIAN_POINT ( 'NONE',  ( 3.999999999999996447, -23.95836489284496906, -5.908293092017329329 ) ) ;
#10163=DIRECTION ( 'NONE',  ( -0.000000000000000000, 1.000000000000000000, -0.000000000000000000 ) ) ;
#10164=CARTESIAN_POINT ( 'NONE',  ( 1.071796769724504328, -25.89093278161442768, -5.720816794851426579 ) ) ;
#10165=CARTESIAN_POINT ( 'NONE',  ( -2.121784821874996396, -18.60988431229980833, -8.703424286353433459 ) ) ;
#10166=ORIENTED_EDGE ( 'NONE', *, *, #11440, .F. ) ;
#10180=CARTESIAN_POINT ( 'NONE',  ( -1.999999999999996225, -21.18631794911805599, -12.01519454243453211 ) ) ;
#10181=ORIENTED_EDGE ( 'NONE', *, *, #17408, .T. ) ;
#10184=CARTESIAN_POINT ( 'NONE',  ( -9.997135785739454050, -9.916563802935840499, 4.936593098934934254 ) ) ;
#10185=CARTESIAN_POINT ( 'NONE',  ( 2.121784821875004390, -18.10442007776545736, -7.981546547323755014 ) ) ;
#10187=CARTESIAN_POINT ( 'NONE',  ( 3.250767888004682415, -21.90484815091188509, -2.246271217071878823 ) ) ;
#10188=ORIENTED_EDGE ( 'NONE', *, *, #15907, .F. ) ;
#10189=ORIENTED_EDGE ( 'NONE', *, *, #11841, .T. ) ;
#10192=DIRECTION ( 'NONE',  ( -0.000000000000000000, -0.5735764363510414965, -0.8191520442889950182 ) ) ;
#10193=CARTESIAN_POINT ( 'NONE',  ( 1.999999999999994449, -27.76495267570075143, -9.331504893052493088 ) ) ;
#10197=CARTESIAN_POINT ( 'NONE',  ( -2.121784821874996396, -18.57762063775506078, -8.657346983862177936 ) ) ;
#10200=CARTESIAN_POINT ( 'NONE',  ( -2.121784821875005722, -29.96497677686856775, -12.10570662107570961 ) ) ;
#10202=CARTESIAN_POINT ( 'NONE',  ( 2.121784821875004390, -19.68534013045801956, -10.23933436939529606 ) ) ;
#10204=CARTESIAN_POINT ( 'NONE',  ( -5.002737418184070251, -14.83391033323086994, -6.661572473864194599 ) ) ;
#10205=EDGE_CURVE ( 'NONE', #3333, #6382, #13220, .T. ) ;
#10209=ORIENTED_EDGE ( 'NONE', *, *, #6272, .F. ) ;
#10211=CARTESIAN_POINT ( 'NONE',  ( 2.121784821875004390, -17.84631068140748766, -7.612928127393706390 ) ) ;
#10217=CARTESIAN_POINT ( 'NONE',  ( -4.243569643749997233, -24.97988077932658513, -15.66497698787144977 ) ) ;
#10225=CARTESIAN_POINT ( 'NONE',  ( 4.730628863548789710E-15, -22.53200002504703647, -16.44053107954607640 ) ) ;
#10227=CARTESIAN_POINT ( 'NONE',  ( 1.533898589781675205E-14, -28.28997139934942595, -9.146999014867043698 ) ) ;
#10228=CARTESIAN_POINT ( 'NONE',  ( 2.121784821875004390, -22.75038921220889065, -14.61667810606461337 ) ) ;
#10234=TOROIDAL_SURFACE ( 'NONE', #10830, 4.400000000000002132, 0.4000000000000000222 ) ;
#10235=CARTESIAN_POINT ( 'NONE',  ( -5.330712181944245322E-15, -28.84980074951425877, -8.377325144622332687 ) ) ;
#10236=CARTESIAN_POINT ( 'NONE',  ( 15.00000000000000355, -4.000000000000000000, -30.00000000000000000 ) ) ;
#10237=CARTESIAN_POINT ( 'NONE',  ( 4.713407268011036227E-15, -16.71294755970913215, -7.639718490920175853 ) ) ;
#10243=CARTESIAN_POINT ( 'NONE',  ( 2.000000000000004441, -22.84251990978664182, -14.38049607132576746 ) ) ;
#10247=CARTESIAN_POINT ( 'NONE',  ( 4.243569643750000786, -24.28743054458419692, -10.40456545371456620 ) ) ;
#10250=ORIENTED_EDGE ( 'NONE', *, *, #5297, .T. ) ;
#10253=CARTESIAN_POINT ( 'NONE',  ( 4.243569643750000786, -25.06175873365810247, -11.51042071350471119 ) ) ;
#10255=DIRECTION ( 'NONE',  ( 0.6985514936319299206, -0.7155597883787208069, 0.000000000000000000 ) ) ;
#10257=CARTESIAN_POINT ( 'NONE',  ( -4.243569643750000786, -21.83539127918348299, -6.902690464379118040 ) ) ;
#10272=CARTESIAN_POINT ( 'NONE',  ( 4.713407268011036227E-15, -17.68085779534656510, -9.022037564651093078 ) ) ;
#10274=VECTOR ( 'NONE', #2866, 1000.000000000000000 ) ;
#10276=CIRCLE ( 'NONE', #16829, 2.000000000000001776 ) ;
#10278=CARTESIAN_POINT ( 'NONE',  ( -7.256038713980983879, -10.36824963302216318, 4.264491367891564799 ) ) ;
#10279=CARTESIAN_POINT ( 'NONE',  ( 4.243569643750000786, -21.93218230281772918, -7.040922371852881945 ) ) ;
#10289=CARTESIAN_POINT ( 'NONE',  ( -1.071796769724494114, -29.78562712842163762, -11.28301676311397017 ) ) ;
#10293=CARTESIAN_POINT ( 'NONE',  ( 8.500000000000019540, 0.000000000000000000, -18.49999999999998934 ) ) ;
#10295=CARTESIAN_POINT ( 'NONE',  ( -5.330712181944245322E-15, -26.01059738957660272, -4.322522525391808479 ) ) ;
#10298=CARTESIAN_POINT ( 'NONE',  ( 2.121784821874994176, -29.66384914778427628, -11.67565179782398310 ) ) ;
#10299=CARTESIAN_POINT ( 'NONE',  ( -4.000000000000004441, -28.43226109638308330, -12.29767903747149660 ) ) ;
#10300=CARTESIAN_POINT ( 'NONE',  ( 2.121784821874994176, -25.27598940969881269, -5.409138659013170702 ) ) ;
#10302=AXIS2_PLACEMENT_3D ( 'NONE', #11414, #15262, #2558 ) ;
#10303=CARTESIAN_POINT ( 'NONE',  ( 1.743066579297358403E-15, -23.41446612136426708, -16.13163023522068684 ) ) ;
#10304=CARTESIAN_POINT ( 'NONE',  ( -2.000000000000005773, -23.48463852013604480, -3.218582763552638948 ) ) ;
#10307=VERTEX_POINT ( 'NONE', #17019 ) ;
#10308=CARTESIAN_POINT ( 'NONE',  ( -4.000000000000004441, -21.52783474451236145, -2.437136305349486332 ) ) ;
#10313=CARTESIAN_POINT ( 'NONE',  ( -4.243569643750000786, -25.93287794636623644, -12.75450788076862452 ) ) ;
#10322=CARTESIAN_POINT ( 'NONE',  ( 2.121784821874994176, -29.14763035506834044, -10.93841495796388763 ) ) ;
#10323=EDGE_CURVE ( 'NONE', #12341, #6360, #18003, .T. ) ;
#10324=CARTESIAN_POINT ( 'NONE',  ( -4.243569643750000786, -24.64233096457639505, -10.91141578111838584 ) ) ;
#10329=CARTESIAN_POINT ( 'NONE',  ( -6.158835246850665095E-15, -22.64013793229036864, -15.02577497543054186 ) ) ;
#10330=CARTESIAN_POINT ( 'NONE',  ( 4.243569643750000786, -23.48083868096554028, -9.252632891433169249 ) ) ;
#10336=CARTESIAN_POINT ( 'NONE',  ( 1.533898589781675205E-14, -27.25753381391755426, -7.672525335146852754 ) ) ;
#10338=CARTESIAN_POINT ( 'NONE',  ( -5.279047395330986450E-15, -29.57119263748722204, -9.897923940636554008 ) ) ;
#10343=CARTESIAN_POINT ( 'NONE',  ( -2.121784821875005722, -26.35144522785700616, -6.945048742055040414 ) ) ;
#10346=EDGE_CURVE ( 'NONE', #4066, #1806, #12632, .T. ) ;
#10348=LINE ( 'NONE', #8866, #4794 ) ;
#10349=CARTESIAN_POINT ( 'NONE',  ( -4.000000000000004441, -24.36703810445001750, -6.491938924580010983 ) ) ;
#10350=CARTESIAN_POINT ( 'NONE',  ( -2.121784821874996396, -22.22341586131136992, -13.86408216537410354 ) ) ;
#10351=CARTESIAN_POINT ( 'NONE',  ( -2.000000000000005773, -28.13060765457947809, -9.853714322293496863 ) ) ;
#10352=DIRECTION ( 'NONE',  ( 0.000000000000000000, 0.8191520442889952403, -0.5735764363510413855 ) ) ;
#10354=CARTESIAN_POINT ( 'NONE',  ( 4.730628863548789710E-15, -17.88603089060359963, -9.805399520805213598 ) ) ;
#10356=DIRECTION ( 'NONE',  ( -0.000000000000000000, 1.000000000000000000, -0.000000000000000000 ) ) ;
#10359=CARTESIAN_POINT ( 'NONE',  ( 0.000000000000000000, 9.254131787996968228, 30.52396275209373044 ) ) ;
#10362=CARTESIAN_POINT ( 'NONE',  ( 0.000000000000000000, 5.977523610840987267, 32.81826849749789687 ) ) ;
#10366=EDGE_CURVE ( 'NONE', #9005, #12967, #507, .T. ) ;
#10369=ORIENTED_EDGE ( 'NONE', *, *, #13088, .T. ) ;
#10371=CARTESIAN_POINT ( 'NONE',  ( 3.999999999999996447, -24.47458368556090491, -6.645529931877427465 ) ) ;
#10376=DIRECTION ( 'NONE',  ( -0.000000000000000000, -0.5735764363510414965, -0.8191520442889950182 ) ) ;
#10377=CARTESIAN_POINT ( 'NONE',  ( -4.243569643749998122, -20.07580224852517858, -8.661227009200541005 ) ) ;
#10379=CARTESIAN_POINT ( 'NONE',  ( 4.299564228933482956E-15, -16.63909446626264454, -6.455396711050170211 ) ) ;
#10382=CARTESIAN_POINT ( 'NONE',  ( 2.978814741686848677, -10.00000000000000178, 22.09987478887119394 ) ) ;
#10389=CARTESIAN_POINT ( 'NONE',  ( 8.500000000000019540, 0.000000000000000000, 22.49999999999999289 ) ) ;
#10390=CARTESIAN_POINT ( 'NONE',  ( 4.243569643749996345, -23.44441649529964877, -4.929126507931827383 ) ) ;
#10392=( BOUNDED_CURVE ( )  B_SPLINE_CURVE ( 2, ( #8874, #12795, #5569, #8974, #13142, #5662, #9063, #4608, #11219 ),
 .UNSPECIFIED., .F., .T. ) 
 B_SPLINE_CURVE_WITH_KNOTS ( ( 3, 2, 2, 2, 3 ),
 ( 0.2844827586206896686, 0.2873563218390804419, 0.2931034482758620441, 0.2988505747126437018, 0.3017241379310345306 ),
 .UNSPECIFIED. ) 
 CURVE ( )  GEOMETRIC_REPRESENTATION_ITEM ( )  RATIONAL_B_SPLINE_CURVE ( ( 0.9330127018922194093, 0.9330127018922200755, 1.000000000000000000, 0.8660254037844387076, 1.000000000000000000, 0.8660254037844387076, 1.000000000000000000, 0.9330127018922187432, 0.9330127018922194093 ) ) 
 REPRESENTATION_ITEM ( '' )  );
#10393=EDGE_CURVE ( 'NONE', #12581, #10307, #5500, .T. ) ;
#10395=CARTESIAN_POINT ( 'NONE',  ( 4.730628863548789710E-15, -23.04821881776297232, -17.17776791940616832 ) ) ;
#10396=CARTESIAN_POINT ( 'NONE',  ( 1.999999999999994449, -29.57171845020653222, -11.91183383256282724 ) ) ;
#10398=CARTESIAN_POINT ( 'NONE',  ( -2.121784821874996396, -18.35177491594184218, -8.334805866423387499 ) ) ;
#10399=ADVANCED_FACE ( 'NONE', ( #16654 ), #12282, .F. ) ;
#10403=CARTESIAN_POINT ( 'NONE',  ( -1.448116719718852696, -10.00000000000000355, -4.839896329767194416 ) ) ;
#10413=CARTESIAN_POINT ( 'NONE',  ( -4.243569643750000786, -25.15854975729233090, -11.64865262097848309 ) ) ;
#10416=CARTESIAN_POINT ( 'NONE',  ( 6.660876705454565894, -10.00000000000000178, -8.457461752749473760 ) ) ;
#10418=CARTESIAN_POINT ( 'NONE',  ( 4.243569643750000786, -24.80364933730013277, -11.14180229357466345 ) ) ;
#10420=DIRECTION ( 'NONE',  ( 0.000000000000000000, 0.000000000000000000, 1.000000000000000000 ) ) ;
#10422=CARTESIAN_POINT ( 'NONE',  ( -4.243569643750004339, -26.88587511340589131, -9.844038773665804598 ) ) ;
#10425=DIRECTION ( 'NONE',  ( 0.8191520442889951292, 0.4698463103929522156, -0.3289899283371602867 ) ) ;
#10427=CARTESIAN_POINT ( 'NONE',  ( 2.121784821874994176, -26.01805392422797070, -6.468916616312057499 ) ) ;
#10436=CARTESIAN_POINT ( 'NONE',  ( -4.000000000000000888, -25.33599996764090534, -11.90207778518377246 ) ) ;
#10437=CIRCLE ( 'NONE', #11316, 3.000000000000000444 ) ;
#10441=CARTESIAN_POINT ( 'NONE',  ( -4.243569643749998122, -20.88239411214383523, -9.813159571481939736 ) ) ;
#10446=CARTESIAN_POINT ( 'NONE',  ( -4.243569643750000786, -25.19081343183707844, -11.69472992346973861 ) ) ;
#10447=CARTESIAN_POINT ( 'NONE',  ( -6.938893903907228378E-15, 6.938893903907228378E-15, 30.00000000000000000 ) ) ;
#10450=CARTESIAN_POINT ( 'NONE',  ( -1.661723472263481630E-14, -20.31715336506863423, -11.70820919606011579 ) ) ;
#10451=CARTESIAN_POINT ( 'NONE',  ( -5.330712181944245322E-15, -30.91467592037801282, -11.32627250406271635 ) ) ;
#10454=CARTESIAN_POINT ( 'NONE',  ( -8.500000000000005329, 10.00000000000000000, -20.49999999999999645 ) ) ;
#10455=CARTESIAN_POINT ( 'NONE',  ( -4.000000000000004441, -24.88325689716596045, -7.229175764440105567 ) ) ;
#10456=CARTESIAN_POINT ( 'NONE',  ( -5.577813053751546416E-15, -25.38624068961733826, -5.000041789647243107 ) ) ;
#10458=VERTEX_POINT ( 'NONE', #14502 ) ;
#10460=CARTESIAN_POINT ( 'NONE',  ( 0.000000000000000000, 5.977523610840987267, 32.81826849749789687 ) ) ;
#10465=AXIS2_PLACEMENT_3D ( 'NONE', #717, #13490, #12099 ) ;
#10468=CARTESIAN_POINT ( 'NONE',  ( 4.000000000000000888, -22.56132395608780783, -7.939429769928989522 ) ) ;
#10472=CARTESIAN_POINT ( 'NONE',  ( 9.184850993605147944E-16, -10.54254386713301628, 22.30101802474215589 ) ) ;
#10473=CARTESIAN_POINT ( 'NONE',  ( 4.243569643750003451, -18.87129173218799849, -6.941007716193646537 ) ) ;
#10474=CARTESIAN_POINT ( 'NONE',  ( 4.730628863548789710E-15, -19.95090606146734658, -12.75434688024559726 ) ) ;
#10477=CARTESIAN_POINT ( 'NONE',  ( 1.071796769724487675, -29.82710107677840483, -11.34224769979141456 ) ) ;
#10479=CARTESIAN_POINT ( 'NONE',  ( 1.533898589781675205E-14, -28.48355344591296401, -9.423462828807814162 ) ) ;
#10482=CARTESIAN_POINT ( 'NONE',  ( 1.071796769724494780, -28.21391734883615143, -9.038382574221850874 ) ) ;
#10486=CARTESIAN_POINT ( 'NONE',  ( -4.243569643749997233, -19.55958345580923918, -7.923990169340445533 ) ) ;
#10490=CARTESIAN_POINT ( 'NONE',  ( 2.121784821875004390, -23.29887167946958115, -15.39999224841596437 ) ) ;
#10491=CARTESIAN_POINT ( 'NONE',  ( 2.000000000000004441, -24.06853954178204447, -16.13143356498672887 ) ) ;
#10492=CARTESIAN_POINT ( 'NONE',  ( 2.121784821874994176, -24.24355182426693389, -3.934664979292979314 ) ) ;
#10497=VERTEX_POINT ( 'NONE', #10303 ) ;
#10499=( BOUNDED_CURVE ( )  B_SPLINE_CURVE ( 3, ( #3047, #1844, #3133, #6089 ),
 .UNSPECIFIED., .F., .F. ) 
 B_SPLINE_CURVE_WITH_KNOTS ( ( 4, 4 ),
 ( 2.111895852752041502, 3.141592653589793116 ),
 .UNSPECIFIED. ) 
 CURVE ( )  GEOMETRIC_REPRESENTATION_ITEM ( )  RATIONAL_B_SPLINE_CURVE ( ( 1.000000000000000000, 0.9135782535825734962, 0.9135782535825734962, 1.000000000000000000 ) ) 
 REPRESENTATION_ITEM ( '' )  );
#10500=CARTESIAN_POINT ( 'NONE',  ( 4.243569643749996345, -21.89576011715183768, -2.717415988351541856 ) ) ;
#10502=CYLINDRICAL_SURFACE ( 'NONE', #5622, 4.000000000000000000 ) ;
#10503=CARTESIAN_POINT ( 'NONE',  ( 1.071796769724495224, -17.23136730949185491, -7.301249991555458507 ) ) ;
#10506=SHAPE_REPRESENTATION_RELATIONSHIP ( 'NONE' , 'NONE' ,  #17791, #6498 ) ;
#10507=CARTESIAN_POINT ( 'NONE',  ( -2.121784821874996396, -22.70737097948255823, -14.55524170274294171 ) ) ;
#10509=EDGE_CURVE ( 'NONE', #10807, #10740, #10586, .T. ) ;
#10511=CARTESIAN_POINT ( 'NONE',  ( -4.000000000000000888, -23.98092563605662875, -9.966831079544254735 ) ) ;
#10512=CARTESIAN_POINT ( 'NONE',  ( 4.243569643749996345, -27.09021171885596146, -10.13586168944375210 ) ) ;
#10514=CARTESIAN_POINT ( 'NONE',  ( 4.730628863548789710E-15, -20.69297057599650458, -13.81412483754448495 ) ) ;
#10517=CARTESIAN_POINT ( 'NONE',  ( 2.000000000000004441, -23.10062930614460797, -14.74911449125581520 ) ) ;
#10518=CARTESIAN_POINT ( 'NONE',  ( 4.730628863548789710E-15, -19.91864238692259903, -12.70826957775434352 ) ) ;
#10523=EDGE_CURVE ( 'NONE', #16355, #17896, #3419, .T. ) ;
#10526=CARTESIAN_POINT ( 'NONE',  ( 0.000000000000000000, 5.977523610840987267, 32.81826849749789687 ) ) ;
#10529=ORIENTED_EDGE ( 'NONE', *, *, #14377, .F. ) ;
#10530=CARTESIAN_POINT ( 'NONE',  ( 4.730628863548789710E-15, -18.40224968331953548, -10.54263636066531085 ) ) ;
#10532=ORIENTED_EDGE ( 'NONE', *, *, #2769, .T. ) ;
#10536=CARTESIAN_POINT ( 'NONE',  ( 4.243569643750003451, -24.06574333389212228, -14.35945341728585767 ) ) ;
#10537=CARTESIAN_POINT ( 'NONE',  ( 5.348585110054253633, -10.20669165899109743, -1.142694657456339691 ) ) ;
#10539=CARTESIAN_POINT ( 'NONE',  ( 4.243569643750003451, -18.12922721765884049, -5.881229758894760629 ) ) ;
#10541=CARTESIAN_POINT ( 'NONE',  ( 1.071796769724504328, -26.47167892412480583, -6.550208240700799323 ) ) ;
#10542=CARTESIAN_POINT ( 'NONE',  ( -4.000000000000004441, -24.62514750080799075, -6.860557344510057831 ) ) ;
#10543=ORIENTED_EDGE ( 'NONE', *, *, #17831, .T. ) ;
#10545=CARTESIAN_POINT ( 'NONE',  ( -1.071796769724505882, -18.17622414369163053, -8.650645395974535745 ) ) ;
#10554=CARTESIAN_POINT ( 'NONE',  ( -4.000000000000000888, -22.69037865426678380, -8.123738979894017831 ) ) ;
#10555=ORIENTED_EDGE ( 'NONE', *, *, #8455, .T. ) ;
#10558=EDGE_CURVE ( 'NONE', #6382, #10757, #13277, .T. ) ;
#10562=CARTESIAN_POINT ( 'NONE',  ( 4.243569643750000786, -20.38352592466991808, -4.829211852272596417 ) ) ;
#10563=VECTOR ( 'NONE', #14784, 1000.000000000000000 ) ;
#10564=CARTESIAN_POINT ( 'NONE',  ( -2.121784821875005722, -27.38388281328888141, -8.419522421775232246 ) ) ;
#10565=EDGE_CURVE ( 'NONE', #16355, #16719, #6234, .T. ) ;
#10566=CARTESIAN_POINT ( 'NONE',  ( 0.4488142760818575883, -30.27607861724349902, -12.00111911307740087 ) ) ;
#10568=CARTESIAN_POINT ( 'NONE',  ( 5.694236848974395748, -11.38679575279332212, 16.60313092159397641 ) ) ;
#10571=CARTESIAN_POINT ( 'NONE',  ( -2.121784821875005722, -29.96497677686856775, -12.10570662107570961 ) ) ;
#10575=CARTESIAN_POINT ( 'NONE',  ( -4.243569643750005227, -23.53045296075229942, -5.051999314575184030 ) ) ;
#10579=CARTESIAN_POINT ( 'NONE',  ( -2.121784821875005722, -29.44875798415262835, -11.36846978121561236 ) ) ;
#10581=CARTESIAN_POINT ( 'NONE',  ( -2.000000000000005773, -29.61473668293285399, -11.97327023588450601 ) ) ;
#10583=CARTESIAN_POINT ( 'NONE',  ( -2.121784821875005722, -24.28657005699325921, -3.996101382614658970 ) ) ;
#10586=LINE ( 'NONE', #9196, #13526 ) ;
#10587=CARTESIAN_POINT ( 'NONE',  ( 1.743066579297358403E-15, -23.60804816792780159, -16.40809404916146264 ) ) ;
#10590=ORIENTED_EDGE ( 'NONE', *, *, #3887, .T. ) ;
#10593=CARTESIAN_POINT ( 'NONE',  ( 4.299564228933482956E-15, -16.44551241969911359, -6.178932897109397970 ) ) ;
#10599=CARTESIAN_POINT ( 'NONE',  ( 4.730628863548789710E-15, -20.95107997235447073, -14.18274325747453268 ) ) ;
#10602=CARTESIAN_POINT ( 'NONE',  ( 1.533898589781675205E-14, -27.19300646412311551, -7.580370729157575482 ) ) ;
#10604=CARTESIAN_POINT ( 'NONE',  ( -5.330712181944245322E-15, -29.14017382041697601, -8.792020867043637722 ) ) ;
#10606=( BOUNDED_CURVE ( )  B_SPLINE_CURVE ( 2, ( #9414, #10811, #2394, #8025, #13776, #13682, #9602, #12287, #5248 ),
 .UNSPECIFIED., .F., .T. ) 
 B_SPLINE_CURVE_WITH_KNOTS ( ( 3, 2, 2, 2, 3 ),
 ( 0.7155172413793103869, 0.7183908045977011048, 0.7241379310344827624, 0.7298850574712644201, 0.7327586206896552490 ),
 .UNSPECIFIED. ) 
 CURVE ( )  GEOMETRIC_REPRESENTATION_ITEM ( )  RATIONAL_B_SPLINE_CURVE ( ( 0.9330127018922194093, 0.9330127018922206306, 1.000000000000000000, 0.8660254037844387076, 1.000000000000000000, 0.8660254037844387076, 1.000000000000000000, 0.9330127018922180770, 0.9330127018922194093 ) ) 
 REPRESENTATION_ITEM ( '' )  );
#10610=CARTESIAN_POINT ( 'NONE',  ( 2.121784821874994176, -26.79238211330187625, -7.574771876102201595 ) ) ;
#10611=ORIENTED_EDGE ( 'NONE', *, *, #1576, .F. ) ;
#10613=LINE ( 'NONE', #17788, #2649 ) ;
#10623=CARTESIAN_POINT ( 'NONE',  ( -2.121784821875005722, -25.83522643514106676, -6.207811902194944054 ) ) ;
#10628=EDGE_CURVE ( 'NONE', #11984, #2690, #6600, .T. ) ;
#10630=CARTESIAN_POINT ( 'NONE',  ( -3.852824484123190008, -26.05880171954380842, -15.10261301480446683 ) ) ;
#10632=CARTESIAN_POINT ( 'NONE',  ( 7.634387662550983222, -10.16876176238401186, 11.61152380675876650 ) ) ;
#10634=CARTESIAN_POINT ( 'NONE',  ( -2.121784821875005722, -22.73791367884544812, -1.784390863034371666 ) ) ;
#10635=ORIENTED_EDGE ( 'NONE', *, *, #10346, .F. ) ;
#10638=CARTESIAN_POINT ( 'NONE',  ( -4.000000000000000888, -22.75490600406122255, -8.215893585883295103 ) ) ;
#10644=VECTOR ( 'NONE', #2953, 1000.000000000000000 ) ;
#10651=CARTESIAN_POINT ( 'NONE',  ( -1.999999999999996225, -18.86333338189633579, -8.697628763064102486 ) ) ;
#10657=AXIS2_PLACEMENT_3D ( 'NONE', #16376, #7823, #10425 ) ;
#10658=CARTESIAN_POINT ( 'NONE',  ( -2.121784821875005722, -22.70565000430070057, -1.738313560543115477 ) ) ;
#10659=CARTESIAN_POINT ( 'NONE',  ( 2.121784821874994176, -27.59897397692052934, -8.726704438383601214 ) ) ;
#10660=DIRECTION ( 'NONE',  ( -0.000000000000000000, -0.5735764363510414965, -0.8191520442889950182 ) ) ;
#10662=CARTESIAN_POINT ( 'NONE',  ( 0.7594769011888096166, -10.00000000000000178, 23.07585096715833473 ) ) ;
#10665=CARTESIAN_POINT ( 'NONE',  ( -2.121784821874996396, -24.03018163581715072, -16.44441110488443769 ) ) ;
#10668=CARTESIAN_POINT ( 'NONE',  ( -8.999999999999996447, -13.00000000000000178, 15.14468620625656925 ) ) ;
#10669=CARTESIAN_POINT ( 'NONE',  ( -2.121784821875005722, -22.70565000430070057, -1.738313560543115477 ) ) ;
#10673=CARTESIAN_POINT ( 'NONE',  ( 4.000000000000000888, -25.91674610874139972, -12.73146922901961098 ) ) ;
#10675=CARTESIAN_POINT ( 'NONE',  ( -2.121784821875005722, -23.77035126427731981, -3.258864542754563942 ) ) ;
#10679=CARTESIAN_POINT ( 'NONE',  ( -3.706921591972381904E-14, -16.89720386262061425, -6.824015130980216171 ) ) ;
#10680=DIRECTION ( 'NONE',  ( 0.000000000000000000, 0.8191520442889952403, -0.5735764363510413855 ) ) ;
#10688=ORIENTED_EDGE ( 'NONE', *, *, #8787, .F. ) ;
#10690=PRESENTATION_STYLE_ASSIGNMENT (( #7901 ) ) ;
#10691=EDGE_CURVE ( 'NONE', #17988, #7315, #3528, .T. ) ;
#10692=CARTESIAN_POINT ( 'NONE',  ( -2.121784821875005722, -29.15838491324991466, -10.95377405879430910 ) ) ;
#10695=CARTESIAN_POINT ( 'NONE',  ( 2.121784821874994176, -27.85708337327849549, -9.095322858313648950 ) ) ;
#10697=CARTESIAN_POINT ( 'NONE',  ( 2.121784821874994176, -28.11519276963646519, -9.463941278243694910 ) ) ;
#10698=CARTESIAN_POINT ( 'NONE',  ( 0.000000000000000000, 5.977523610840987267, 32.81826849749789687 ) ) ;
#10701=CARTESIAN_POINT ( 'NONE',  ( -4.243569643749997233, -21.10823983395705383, -10.13570068892072840 ) ) ;
#10702=ORIENTED_EDGE ( 'NONE', *, *, #11122, .F. ) ;
#10713=CARTESIAN_POINT ( 'NONE',  ( 4.243569643750003451, -20.19410238852258743, -8.830177118335141628 ) ) ;
#10716=AXIS2_PLACEMENT_3D ( 'NONE', #15221, #3983, #16519 ) ;
#10717=( BOUNDED_CURVE ( )  B_SPLINE_CURVE ( 2, ( #15017, #12212, #10917, #17897, #3693, #1286, #15199, #1098, #12478 ),
 .UNSPECIFIED., .F., .T. ) 
 B_SPLINE_CURVE_WITH_KNOTS ( ( 3, 2, 2, 2, 3 ),
 ( 0.09482758620689656082, 0.09770114942528736190, 0.1034482758620689641, 0.1091954022988505801, 0.1120689655172413812 ),
 .UNSPECIFIED. ) 
 CURVE ( )  GEOMETRIC_REPRESENTATION_ITEM ( )  RATIONAL_B_SPLINE_CURVE ( ( 0.9330127018922194093, 0.9330127018922195203, 1.000000000000000000, 0.8660254037844387076, 1.000000000000000000, 0.8660254037844387076, 1.000000000000000000, 0.9330127018922194093, 0.9330127018922194093 ) ) 
 REPRESENTATION_ITEM ( '' )  );
#10719=DIRECTION ( 'NONE',  ( -0.000000000000000000, 1.000000000000000000, -0.000000000000000000 ) ) ;
#10721=CARTESIAN_POINT ( 'NONE',  ( -1.098144841579475894, -23.88987786432218385, -16.68580408662743864 ) ) ;
#10722=CARTESIAN_POINT ( 'NONE',  ( 9.175740695410866010, -10.00000000000000178, -2.948767207631089793 ) ) ;
#10723=CARTESIAN_POINT ( 'NONE',  ( 4.000000000000003553, -22.71293939747845769, -12.18227696742093791 ) ) ;
#10724=CARTESIAN_POINT ( 'NONE',  ( -4.243569643750005227, -22.53027904986517527, -3.623602937346249497 ) ) ;
#10725=ORIENTED_EDGE ( 'NONE', *, *, #9426, .T. ) ;
#10728=CARTESIAN_POINT ( 'NONE',  ( -5.279047395330986450E-15, -27.24820807026550540, -6.580358161266123496 ) ) ;
#10729=AXIS2_PLACEMENT_3D ( 'NONE', #10460, #6291, #458 ) ;
#10732=ORIENTED_EDGE ( 'NONE', *, *, #4053, .F. ) ;
#10734=EDGE_CURVE ( 'NONE', #8825, #4590, #12498, .T. ) ;
#10740=VERTEX_POINT ( 'NONE', #9646 ) ;
#10742=CARTESIAN_POINT ( 'NONE',  ( -4.000000000000000888, -20.36739408704506715, -4.806173200523589095 ) ) ;
#10748=CARTESIAN_POINT ( 'NONE',  ( 1.071796769724500109, -22.07091849049882271, -14.21284536423708467 ) ) ;
#10749=CARTESIAN_POINT ( 'NONE',  ( 2.121784821874994176, -22.92074116793234140, -2.045495577151484223 ) ) ;
#10750=CARTESIAN_POINT ( 'NONE',  ( 4.243569643750000786, -24.02932114822622722, -10.03594703378452024 ) ) ;
#10751=CARTESIAN_POINT ( 'NONE',  ( -1.657547274258957426, -30.02955948770827277, -12.21735830786932731 ) ) ;
#10753=CARTESIAN_POINT ( 'NONE',  ( -3.132887738848217918, -10.75727755901226956, 20.85177242120514407 ) ) ;
#10755=CARTESIAN_POINT ( 'NONE',  ( -1.071796769724486786, -19.46677112548146127, -10.49373749562478153 ) ) ;
#10756=CARTESIAN_POINT ( 'NONE',  ( -2.121784821874996396, -23.51396284310121487, -15.70717426502434044 ) ) ;
#10757=VERTEX_POINT ( 'NONE', #9468 ) ;
#10758=VECTOR ( 'NONE', #12686, 1000.000000000000000 ) ;
#10762=CARTESIAN_POINT ( 'NONE',  ( 2.121784821874994176, -23.43695996064828435, -2.782732417011581028 ) ) ;
#10765=CARTESIAN_POINT ( 'NONE',  ( -3.999999999999997335, -22.88501232838376254, -12.42802258070763877 ) ) ;
#10767=CARTESIAN_POINT ( 'NONE',  ( -4.243569643749997233, -18.81751894128008118, -6.864212212041558736 ) ) ;
#10772=CARTESIAN_POINT ( 'NONE',  ( -8.500000000000005329, 10.00000000000000000, 22.50000000000000000 ) ) ;
#10773=CARTESIAN_POINT ( 'NONE',  ( -5.577813053751546416E-15, -25.96698683212770931, -5.829433235496615850 ) ) ;
#10774=VERTEX_POINT ( 'NONE', #5816 ) ;
#10777=CARTESIAN_POINT ( 'NONE',  ( -3.706921591972381904E-14, -18.25227819420489439, -8.759261836619732122 ) ) ;
#10778=CARTESIAN_POINT ( 'NONE',  ( 1.533898589781675205E-14, -27.45111586048108521, -7.948989149087622330 ) ) ;
#10781=CARTESIAN_POINT ( 'NONE',  ( 2.121784821874994176, -26.79238211330187625, -7.574771876102201595 ) ) ;
#10783=CARTESIAN_POINT ( 'NONE',  ( -3.604268994871580034, -29.27461685626023424, -13.12700564398634917 ) ) ;
#10784=CARTESIAN_POINT ( 'NONE',  ( -1.999999999999996225, -21.18631794911805599, -12.01519454243453211 ) ) ;
#10785=CARTESIAN_POINT ( 'NONE',  ( 2.121784821874994176, -27.85708337327849549, -9.095322858313648950 ) ) ;
#10788=EDGE_CURVE ( 'NONE', #7842, #17988, #5517, .T. ) ;
#10793=CARTESIAN_POINT ( 'NONE',  ( -5.577813053751546416E-15, -23.38589286854802296, -2.143249036196138047 ) ) ;
#10795=CARTESIAN_POINT ( 'NONE',  ( 4.243569643749996345, -23.96063528801558462, -5.666363347791923744 ) ) ;
#10796=ORIENTED_EDGE ( 'NONE', *, *, #8082, .T. ) ;
#10804=CARTESIAN_POINT ( 'NONE',  ( -5.577813053751546416E-15, -23.32136551875358776, -2.051094430206859887 ) ) ;
#10807=VERTEX_POINT ( 'NONE', #18124 ) ;
#10808=CARTESIAN_POINT ( 'NONE',  ( -2.121784821874996396, -18.35177491594184218, -8.334805866423387499 ) ) ;
#10810=VERTEX_POINT ( 'NONE', #14262 ) ;
#10811=CARTESIAN_POINT ( 'NONE',  ( 1.071796769724504328, -25.11660459254052924, -4.614961535061283371 ) ) ;
#10813=CARTESIAN_POINT ( 'NONE',  ( -0.5794581908436565731, -23.80035312255054691, -16.75679979387895102 ) ) ;
#10814=CARTESIAN_POINT ( 'NONE',  ( 6.428571428571432378, -11.73421655796352248, 14.25837509840158290 ) ) ;
#10816=CARTESIAN_POINT ( 'NONE',  ( 2.121784821874994176, -23.46922363519303190, -2.828809719502837439 ) ) ;
#10819=CARTESIAN_POINT ( 'NONE',  ( -4.000000000000000888, -23.27112479677715839, -8.953130425743392351 ) ) ;
#10822=ORIENTED_EDGE ( 'NONE', *, *, #17154, .T. ) ;
#10823=CARTESIAN_POINT ( 'NONE',  ( 0.000000000000000000, 4.000000000000007105, 4.000000000000000000 ) ) ;
#10827=( BOUNDED_CURVE ( )  B_SPLINE_CURVE ( 2, ( #3529, #17555, #5000, #9080, #9175, #13159, #3439, #10748, #14855 ),
 .UNSPECIFIED., .F., .F. ) 
 B_SPLINE_CURVE_WITH_KNOTS ( ( 3, 2, 2, 2, 3 ),
 ( 0.2327586206896551657, 0.2356321839080459668, 0.2413793103448275967, 0.2471264367816091989, 0.2500000000000000000 ),
 .UNSPECIFIED. ) 
 CURVE ( )  GEOMETRIC_REPRESENTATION_ITEM ( )  RATIONAL_B_SPLINE_CURVE ( ( 0.9330127018922194093, 0.9330127018922194093, 1.000000000000000000, 0.8660254037844387076, 1.000000000000000000, 0.8660254037844387076, 1.000000000000000000, 0.9330127018922197424, 0.9330127018922194093 ) ) 
 REPRESENTATION_ITEM ( '' )  );
#10828=ORIENTED_EDGE ( 'NONE', *, *, #16261, .F. ) ;
#10830=AXIS2_PLACEMENT_3D ( 'NONE', #12828, #224, #5875 ) ;
#10831=CARTESIAN_POINT ( 'NONE',  ( 2.000000000000004441, -17.35769523647485713, -6.547354646805487732 ) ) ;
#10833=CARTESIAN_POINT ( 'NONE',  ( 15.00000000000000355, 10.00000000000000000, -30.00000000000000000 ) ) ;
#10837=CARTESIAN_POINT ( 'NONE',  ( -4.243569643750000786, -24.41648524276317289, -10.58887466367959540 ) ) ;
#10842=DIRECTION ( 'NONE',  ( -0.000000000000000000, -0.000000000000000000, 1.000000000000000000 ) ) ;
#10843=CARTESIAN_POINT ( 'NONE',  ( -3.706921591972381904E-14, -18.76849698692083379, -9.496498676479825818 ) ) ;
#10844=CARTESIAN_POINT ( 'NONE',  ( -4.243569643750000786, -26.73946980998488954, -13.90644044305002502 ) ) ;
#10848=CARTESIAN_POINT ( 'NONE',  ( -2.121784821874996396, -17.02896425960724969, -6.445636464281891520 ) ) ;
#10852=CARTESIAN_POINT ( 'NONE',  ( -4.000000000000004441, -26.36738592551932925, -9.348731678031116488 ) ) ;
#10853=VERTEX_POINT ( 'NONE', #12858 ) ;
#10854=CARTESIAN_POINT ( 'NONE',  ( -1.999999999999996225, -22.79950167706030228, -14.31905966800409402 ) ) ;
#10858=CARTESIAN_POINT ( 'NONE',  ( 2.121784821875004390, -20.94362343770310986, -12.03634916655427922 ) ) ;
#10859=EDGE_CURVE ( 'NONE', #9470, #11559, #330, .T. ) ;
#10860=CARTESIAN_POINT ( 'NONE',  ( -1.071796769724496334, -28.75318954298976237, -9.808543083393779227 ) ) ;
#10861=CARTESIAN_POINT ( 'NONE',  ( 4.299564228933482956E-15, -21.02695420434810814, -12.72190984986098172 ) ) ;
#10863=ORIENTED_EDGE ( 'NONE', *, *, #6381, .F. ) ;
#10866=CARTESIAN_POINT ( 'NONE',  ( -4.000000000000007105, 0.000000000000000000, 5.000000000000000888 ) ) ;
#10867=CARTESIAN_POINT ( 'NONE',  ( 1.999999999999994449, -29.63624580000097097, -12.00398843855210629 ) ) ;
#10868=DIRECTION ( 'NONE',  ( 1.000000000000000000, 0.000000000000000000, 0.000000000000000000 ) ) ;
#10871=CARTESIAN_POINT ( 'NONE',  ( -4.243569643750005227, -25.59532813161604636, -8.000946674015564142 ) ) ;
#10874=DIRECTION ( 'NONE',  ( -0.000000000000000000, -0.5735764363510414965, -0.8191520442889950182 ) ) ;
#10875=CARTESIAN_POINT ( 'NONE',  ( 4.243569643750000786, -27.11050206724947742, -14.43632942169946531 ) ) ;
#10876=CARTESIAN_POINT ( 'NONE',  ( -2.121784821875005722, -26.86766402057294556, -7.682285581915135886 ) ) ;
#10879=AXIS2_PLACEMENT_3D ( 'NONE', #5884, #4678, #236 ) ;
#10880=CARTESIAN_POINT ( 'NONE',  ( -8.500000000000005329, 0.000000000000000000, -18.49999999999999645 ) ) ;
#10882=DIRECTION ( 'NONE',  ( -1.000000000000000000, 0.000000000000000000, 0.000000000000000000 ) ) ;
#10885=CARTESIAN_POINT ( 'NONE',  ( 4.730628863548789710E-15, -17.33754842334290913, -9.022085378453862603 ) ) ;
#10887=FACE_BOUND ( 'NONE', #13354, .T. ) ;
#10890=CARTESIAN_POINT ( 'NONE',  ( 2.000000000000004441, -20.51953534256492162, -11.06293029195533784 ) ) ;
#10898=VERTEX_POINT ( 'NONE', #1946 ) ;
#10899=CARTESIAN_POINT ( 'NONE',  ( 4.730628863548789710E-15, -16.85359330517172083, -8.330925841085024430 ) ) ;
#10903=CARTESIAN_POINT ( 'NONE',  ( 4.243569643750000786, -27.09437022997710187, -14.41329077045383578 ) ) ;
#10904=AXIS2_PLACEMENT_3D ( 'NONE', #14628, #13209, #9228 ) ;
#10907=CARTESIAN_POINT ( 'NONE',  ( -1.999999999999996225, -19.63766157097024490, -9.803484022854247470 ) ) ;
#10909=CARTESIAN_POINT ( 'NONE',  ( -3.999999999999997335, -19.01337138301423124, -6.898746281756922727 ) ) ;
#10910=CARTESIAN_POINT ( 'NONE',  ( 2.121784821875004390, -23.00849860856686036, -14.98529652599465933 ) ) ;
#10911=ORIENTED_EDGE ( 'NONE', *, *, #16258, .F. ) ;
#10913=CARTESIAN_POINT ( 'NONE',  ( 2.000000000000004441, -18.71276956805914082, -8.482601352445005460 ) ) ;
#10915=ORIENTED_EDGE ( 'NONE', *, *, #15904, .F. ) ;
#10916=ORIENTED_EDGE ( 'NONE', *, *, #17852, .T. ) ;
#10917=CARTESIAN_POINT ( 'NONE',  ( 1.999999999999994449, -29.12002700728503513, -11.26675159869200904 ) ) ;
#10920=EDGE_CURVE ( 'NONE', #11829, #94, #8479, .T. ) ;
#10923=CARTESIAN_POINT ( 'NONE',  ( 2.121784821875004390, -22.52454349039567205, -14.29413698862582294 ) ) ;
#10925=CARTESIAN_POINT ( 'NONE',  ( 4.000000000000000888, -20.49644878522406088, -4.990482410488609410 ) ) ;
#10930=CARTESIAN_POINT ( 'NONE',  ( -2.121784821874996396, -17.28707365596521939, -6.814254884211938368 ) ) ;
#10931=CARTESIAN_POINT ( 'NONE',  ( -4.243569643750005227, -24.85326361708688836, -6.941168716716678233 ) ) ;
#10934=DIRECTION ( 'NONE',  ( -0.000000000000000000, -0.5735764363510414965, -0.8191520442889950182 ) ) ;
#10936=CARTESIAN_POINT ( 'NONE',  ( 4.000000000000000888, -23.91639828767208442, -9.874676475568506362 ) ) ;
#10937=DIRECTION ( 'NONE',  ( 0.000000000000000000, 0.8191520442889952403, -0.5735764363510413855 ) ) ;
#10939=ORIENTED_EDGE ( 'NONE', *, *, #11082, .F. ) ;
#10942=CARTESIAN_POINT ( 'NONE',  ( 2.121784821874994176, -23.17885056429031465, -2.414113997081532847 ) ) ;
#10945=CARTESIAN_POINT ( 'NONE',  ( -4.000000000000004441, -27.39982351095120450, -10.82320535775130566 ) ) ;
#10948=CARTESIAN_POINT ( 'NONE',  ( -4.243569643750005227, -22.27216965350720201, -3.254984517416200873 ) ) ;
#10951=CARTESIAN_POINT ( 'NONE',  ( 4.243569643750000786, -24.77138566275538523, -11.09572499108340793 ) ) ;
#10952=CARTESIAN_POINT ( 'NONE',  ( -2.000000000000005773, -28.84040849385894845, -10.86741497609436280 ) ) ;
#10953=CARTESIAN_POINT ( 'NONE',  ( -3.706921591972381904E-14, -17.99416879784692469, -8.390643416689682610 ) ) ;
#10954=AXIS2_PLACEMENT_3D ( 'NONE', #14507, #11700, #17769 ) ;
#10955=CARTESIAN_POINT ( 'NONE',  ( -4.000000000000004441, -25.14136629352392660, -7.597794184370154191 ) ) ;
#10956=ORIENTED_EDGE ( 'NONE', *, *, #12476, .F. ) ;
#10960=EDGE_CURVE ( 'NONE', #2307, #1671, #5414, .T. ) ;
#10962=CARTESIAN_POINT ( 'NONE',  ( 7.143939857752706679, -13.70057337075539117, 0.6943083681407321572 ) ) ;
#10966=CARTESIAN_POINT ( 'NONE',  ( 2.121784821874994176, -27.05049150965984595, -7.943390296032248443 ) ) ;
#10968=EDGE_CURVE ( 'NONE', #18352, #3556, #7383, .T. ) ;
#10970=DIRECTION ( 'NONE',  ( 0.000000000000000000, 0.8191520442889952403, -0.5735764363510413855 ) ) ;
#10972=PLANE ( 'NONE',  #7868 ) ;
#10973=EDGE_CURVE ( 'NONE', #2986, #15033, #14737, .T. ) ;
#10974=CARTESIAN_POINT ( 'NONE',  ( 4.243569643749996345, -25.79966473706612007, -8.292769589793513418 ) ) ;
#10980=CARTESIAN_POINT ( 'NONE',  ( -4.243569643749997233, -20.07580224852517858, -8.661227009200541005 ) ) ;
#10984=FACE_OUTER_BOUND ( 'NONE', #2728, .T. ) ;
#10987=CARTESIAN_POINT ( 'NONE',  ( 0.000000000000000000, 5.977523610840987267, 32.81826849749789687 ) ) ;
#10988=AXIS2_PLACEMENT_3D ( 'NONE', #5703, #2666, #5613 ) ;
#10990=CARTESIAN_POINT ( 'NONE',  ( -4.243569643750000786, -21.06106309010958100, -5.796835204588974833 ) ) ;
#10992=CARTESIAN_POINT ( 'NONE',  ( 0.000000000000000000, -21.06365275836378004, -18.87638460130267148 ) ) ;
#10993=CARTESIAN_POINT ( 'NONE',  ( 2.121784821874994176, -29.63158547323952874, -11.62957449533272580 ) ) ;
#10996=CARTESIAN_POINT ( 'NONE',  ( 3.999999999999993339, 0.000000000000000000, 30.00000000000000000 ) ) ;
#10997=CARTESIAN_POINT ( 'NONE',  ( 4.243569643750000786, -27.12663390452184942, -14.45936807294509308 ) ) ;
#10998=CARTESIAN_POINT ( 'NONE',  ( -4.243569643749997233, -23.68933379753673663, -13.82188488822120931 ) ) ;
#11001=PLANE ( 'NONE',  #627 ) ;
#11002=CARTESIAN_POINT ( 'NONE',  ( 1.999999999999994449, -23.95783908012565888, -3.894383200091054320 ) ) ;
#11008=VERTEX_POINT ( 'NONE', #14831 ) ;
#11009=CARTESIAN_POINT ( 'NONE',  ( 4.730628863548789710E-15, -20.98334364689921827, -14.22882055996578998 ) ) ;
#11012=CARTESIAN_POINT ( 'NONE',  ( 4.713407268011036227E-15, -16.64842020991469695, -7.547563884930901246 ) ) ;
#11019=CARTESIAN_POINT ( 'NONE',  ( -2.121784821874996396, -20.41665008680558913, -11.28375322586376939 ) ) ;
#11024=CARTESIAN_POINT ( 'NONE',  ( -5.279047395330986450E-15, -28.79686444841332360, -8.792068680846410800 ) ) ;
#11025=CARTESIAN_POINT ( 'NONE',  ( 0.000000000000000000, 5.977523610840987267, 32.81826849749789687 ) ) ;
#11027=CARTESIAN_POINT ( 'NONE',  ( 1.475796370471763337E-14, -21.86580974321645598, -13.91991971564040220 ) ) ;
#11031=CARTESIAN_POINT ( 'NONE',  ( 4.713407268011036227E-15, -23.16568246865834979, -16.85517898917136748 ) ) ;
#11035=VECTOR ( 'NONE', #14081, 1000.000000000000000 ) ;
#11036=CARTESIAN_POINT ( 'NONE',  ( 4.713407268011036227E-15, -21.29438934435813024, -14.18269544367176316 ) ) ;
#11039=CARTESIAN_POINT ( 'NONE',  ( -2.121784821875005722, -23.25413247156138397, -2.521627702894468470 ) ) ;
#11042=CARTESIAN_POINT ( 'NONE',  ( -4.243569643749998122, -20.33391164488314828, -9.029845429130586965 ) ) ;
#11047=CARTESIAN_POINT ( 'NONE',  ( -8.500000000000005329, 0.000000000000000000, -20.49999999999999645 ) ) ;
#11051=DIRECTION ( 'NONE',  ( -0.000000000000000000, -0.5735764363510414965, -0.8191520442889950182 ) ) ;
#11052=CARTESIAN_POINT ( 'NONE',  ( 3.999999999999996447, -23.50667344992347196, -5.263210858146513793 ) ) ;
#11054=ORIENTED_EDGE ( 'NONE', *, *, #16322, .F. ) ;
#11056=CARTESIAN_POINT ( 'NONE',  ( -5.330712181944245322E-15, -27.81736316408238707, -6.902851464902143519 ) ) ;
#11062=CARTESIAN_POINT ( 'NONE',  ( 4.243569643750003451, -22.51708695574430763, -12.14774289770557303 ) ) ;
#11063=CARTESIAN_POINT ( 'NONE',  ( 0.5181399714639640663, -10.00000000000201794, -3.173488174263044304 ) ) ;
#11065=CARTESIAN_POINT ( 'NONE',  ( 0.000000000000000000, 5.977523610840987267, 32.81826849749789687 ) ) ;
#11066=CARTESIAN_POINT ( 'NONE',  ( 0.000000000000000000, -27.20729309053124112, -14.57456132866985499 ) ) ;
#11067=CARTESIAN_POINT ( 'NONE',  ( -4.243569643749997233, -19.55958345580923918, -7.923990169340445533 ) ) ;
#11069=LINE ( 'NONE', #2562, #15987 ) ;
#11071=CARTESIAN_POINT ( 'NONE',  ( -1.661723472263481630E-14, -20.05904396871067874, -11.33959077613006450 ) ) ;
#11075=VERTEX_POINT ( 'NONE', #17806 ) ;
#11076=CARTESIAN_POINT ( 'NONE',  ( -4.243569643750004339, -24.07893542801298281, -5.835313456926535025 ) ) ;
#11078=CARTESIAN_POINT ( 'NONE',  ( -5.040478647146445113, -10.97734431112249531, 19.36653379754668336 ) ) ;
#11079=CARTESIAN_POINT ( 'NONE',  ( -5.330712181944246111E-15, -30.65656652402004312, -10.95765408413266861 ) ) ;
#11081=CARTESIAN_POINT ( 'NONE',  ( -2.000000000000005773, -25.22687694484738685, -5.706757097073694496 ) ) ;
#11082=EDGE_CURVE ( 'NONE', #3053, #3352, #14399, .T. ) ;
#11084=CARTESIAN_POINT ( 'NONE',  ( 4.243569643750000786, -26.32004204090319632, -13.30743551066369257 ) ) ;
#11086=CARTESIAN_POINT ( 'NONE',  ( -2.000000000000005773, -26.25931453027926210, -7.181230776793885440 ) ) ;
#11087=CARTESIAN_POINT ( 'NONE',  ( -5.279047395330986450E-15, -26.21577048483363015, -5.105884481545933440 ) ) ;
#11091=CARTESIAN_POINT ( 'NONE',  ( 4.299564228933482956E-15, -17.92964144805248594, -8.298488810700408891 ) ) ;
#11093=CARTESIAN_POINT ( 'NONE',  ( 4.299564228933482956E-15, -17.15531325897858039, -7.192633550910265683 ) ) ;
#11095=ORIENTED_EDGE ( 'NONE', *, *, #3781, .F. ) ;
#11096=CARTESIAN_POINT ( 'NONE',  ( -5.330712181944246111E-15, -29.65639261313291186, -9.529257706903733194 ) ) ;
#11098=CARTESIAN_POINT ( 'NONE',  ( -4.000000000000004441, -23.01196377286574091, -4.556692218940495032 ) ) ;
#11102=DIRECTION ( 'NONE',  ( -0.000000000000000000, -0.5735764363510414965, -0.8191520442889950182 ) ) ;
#11104=CARTESIAN_POINT ( 'NONE',  ( 4.243569643750003451, -21.22653997395446623, -10.30465079805533435 ) ) ;
#11105=ORIENTED_EDGE ( 'NONE', *, *, #9998, .F. ) ;
#11108=CARTESIAN_POINT ( 'NONE',  ( -5.279047395330986450E-15, -27.76442686298143769, -7.317595001126219856 ) ) ;
#11115=CARTESIAN_POINT ( 'NONE',  ( -4.000000000000000888, -26.11032815671481444, -13.00793304497391567 ) ) ;
#11119=EDGE_CURVE ( 'NONE', #10036, #6155, #17762, .T. ) ;
#11120=CARTESIAN_POINT ( 'NONE',  ( -5.279047395330986450E-15, -28.47422770226091160, -8.331295654927085792 ) ) ;
#11121=ORIENTED_EDGE ( 'NONE', *, *, #10973, .T. ) ;
#11122=EDGE_CURVE ( 'NONE', #1667, #15966, #13583, .T. ) ;
#11123=CARTESIAN_POINT ( 'NONE',  ( 2.121784821875004390, -17.36235556323629936, -6.921768590024867329 ) ) ;
#11128=CARTESIAN_POINT ( 'NONE',  ( -4.243569643750004339, -24.30478114982620497, -6.157854574365327238 ) ) ;
#11132=ORIENTED_EDGE ( 'NONE', *, *, #7254, .F. ) ;
#11135=EDGE_CURVE ( 'NONE', #13443, #10810, #14300, .T. ) ;
#11137=CARTESIAN_POINT ( 'NONE',  ( -6.938893903907228378E-15, 6.938893903907228378E-15, 30.00000000000000000 ) ) ;
#11140=CARTESIAN_POINT ( 'NONE',  ( 4.243569643750000786, -24.51327626639741553, -10.72710657115335842 ) ) ;
#11146=CARTESIAN_POINT ( 'NONE',  ( -2.121784821874996396, -20.41665008680558913, -11.28375322586376939 ) ) ;
#11151=CARTESIAN_POINT ( 'NONE',  ( 2.121784821875004390, -19.13685766319732906, -9.456020227043945070 ) ) ;
#11152=FACE_BOUND ( 'NONE', #8100, .T. ) ;
#11157=CARTESIAN_POINT ( 'NONE',  ( 4.000000000000000888, -25.72316406217786522, -12.45500541507884051 ) ) ;
#11160=CARTESIAN_POINT ( 'NONE',  ( 2.121784821874994176, -23.98544242790896774, -3.566046559362932467 ) ) ;
#11167=CARTESIAN_POINT ( 'NONE',  ( -4.648177544792955347E-16, -29.77410042770280185, -11.26655492845805107 ) ) ;
#11168=CARTESIAN_POINT ( 'NONE',  ( 3.604268994871579590, -24.91053875026183562, -15.69445619563776617 ) ) ;
#11170=CARTESIAN_POINT ( 'NONE',  ( -2.121784821875005722, -28.90027551689194496, -10.58515563886426136 ) ) ;
#11173=CARTESIAN_POINT ( 'NONE',  ( 4.000000000000000888, -22.10963251316630362, -7.294347536058173098 ) ) ;
#11174=VECTOR ( 'NONE', #17963, 1000.000000000000000 ) ;
#11178=CARTESIAN_POINT ( 'NONE',  ( -4.000000000000000888, -22.23868721134528670, -7.478656746023200519 ) ) ;
#11181=CARTESIAN_POINT ( 'NONE',  ( -4.000000000000000888, -20.36739408704506715, -4.806173200523589095 ) ) ;
#11184=CARTESIAN_POINT ( 'NONE',  ( -4.243569643749998122, -22.94726928300757862, -12.76210693092232162 ) ) ;
#11187=ORIENTED_EDGE ( 'NONE', *, *, #5587, .T. ) ;
#11188=CIRCLE ( 'NONE', #15951, 4.000000000000000000 ) ;
#11189=DIRECTION ( 'NONE',  ( -0.000000000000000000, -0.5735764363510414965, -0.8191520442889950182 ) ) ;
#11193=CARTESIAN_POINT ( 'NONE',  ( 8.500000000000019540, 0.000000000000000000, 18.49999999999998934 ) ) ;
#11195=( BOUNDED_CURVE ( )  B_SPLINE_CURVE ( 2, ( #162, #9973, #5992, #14349, #1649, #5813, #5901, #4422, #15743 ),
 .UNSPECIFIED., .F., .T. ) 
 B_SPLINE_CURVE_WITH_KNOTS ( ( 3, 2, 2, 2, 3 ),
 ( 0.5775862068965517127, 0.5804597701149425415, 0.5862068965517240882, 0.5919540229885057459, 0.5948275862068965747 ),
 .UNSPECIFIED. ) 
 CURVE ( )  GEOMETRIC_REPRESENTATION_ITEM ( )  RATIONAL_B_SPLINE_CURVE ( ( 0.9330127018922194093, 0.9330127018922194093, 1.000000000000000000, 0.8660254037844387076, 1.000000000000000000, 0.8660254037844387076, 1.000000000000000000, 0.9330127018922194093, 0.9330127018922194093 ) ) 
 REPRESENTATION_ITEM ( '' )  );
#11196=CARTESIAN_POINT ( 'NONE',  ( 4.243569643750000786, -22.22255537372044998, -7.455618094274186092 ) ) ;
#11200=CARTESIAN_POINT ( 'NONE',  ( -1.999999999999996225, -21.76706409162843059, -12.84458598828390130 ) ) ;
#11201=CARTESIAN_POINT ( 'NONE',  ( 0.000000000000000000, -10.00000000000000178, -12.59063537424807677 ) ) ;
#11207=CARTESIAN_POINT ( 'NONE',  ( 4.713407268011036227E-15, -22.39135427958444069, -15.74932372938122427 ) ) ;
#11210=CARTESIAN_POINT ( 'NONE',  ( 2.000000000000004441, -20.71311738912845257, -11.33939410589610652 ) ) ;
#11212=CARTESIAN_POINT ( 'NONE',  ( -4.243569643749997233, -18.55940954492211503, -6.495593792111509224 ) ) ;
#11214=FACE_OUTER_BOUND ( 'NONE', #6720, .T. ) ;
#11215=AXIS2_PLACEMENT_3D ( 'NONE', #16855, #6989, #8119 ) ;
#11216=CARTESIAN_POINT ( 'NONE',  ( 4.730628863548789710E-15, -19.40242359420666318, -11.97103273789424449 ) ) ;
#11219=CARTESIAN_POINT ( 'NONE',  ( 1.533898589781675205E-14, -28.03186200299146336, -8.778380594936995962 ) ) ;
#11220=CARTESIAN_POINT ( 'NONE',  ( 3.999999999999996447, -24.21647428920293876, -6.276911511947378841 ) ) ;
#11223=ORIENTED_EDGE ( 'NONE', *, *, #18203, .T. ) ;
#11226=DIRECTION ( 'NONE',  ( 0.000000000000000000, 0.8191520442889952403, -0.5735764363510413855 ) ) ;
#11231=CARTESIAN_POINT ( 'NONE',  ( -4.243569643749997233, -21.36634923031502353, -10.50431910885077791 ) ) ;
#11233=AXIS2_PLACEMENT_3D ( 'NONE', #12409, #5545, #2695 ) ;
#11235=CARTESIAN_POINT ( 'NONE',  ( 15.00000000000000355, -4.000000000000000000, 30.00000000000000000 ) ) ;
#11236=CYLINDRICAL_SURFACE ( 'NONE', #1659, 4.000000000000000000 ) ;
#11237=CARTESIAN_POINT ( 'NONE',  ( 4.730628863548789710E-15, -19.43468726875141073, -12.01711004038550001 ) ) ;
#11245=CARTESIAN_POINT ( 'NONE',  ( 4.730628863548789710E-15, -17.07943902698494298, -8.653466958523816643 ) ) ;
#11246=DIRECTION ( 'NONE',  ( -0.000000000000000000, -0.5735764363510414965, -0.8191520442889950182 ) ) ;
#11250=CARTESIAN_POINT ( 'NONE',  ( -1.071796769724496334, -25.39776739033617048, -5.016503624303159548 ) ) ;
#11251=CARTESIAN_POINT ( 'NONE',  ( 4.898587196589413815E-16, 2.700915433685006750, 35.11257424290206330 ) ) ;
#11254=CARTESIAN_POINT ( 'NONE',  ( 4.243569643750000786, -20.67389899557263533, -5.243907574693898788 ) ) ;
#11260=CARTESIAN_POINT ( 'NONE',  ( -4.000000000000004441, -24.30251075465558586, -6.399784318590733712 ) ) ;
#11262=CARTESIAN_POINT ( 'NONE',  ( 2.121784821874994176, -29.63158547323952874, -11.62957449533272580 ) ) ;
#11264=CARTESIAN_POINT ( 'NONE',  ( -2.000000000000005773, -26.51742392663723180, -7.549849196723933176 ) ) ;
#11265=CARTESIAN_POINT ( 'NONE',  ( -4.000000000000000888, -21.72246841862934730, -6.741419906163105047 ) ) ;
#11269=CARTESIAN_POINT ( 'NONE',  ( -1.071796769724486786, -19.01507968255996417, -9.848655261753959778 ) ) ;
#11270=EDGE_CURVE ( 'NONE', #13588, #15144, #10276, .T. ) ;
#11275=CARTESIAN_POINT ( 'NONE',  ( 4.243569643750000786, -25.57797752637403832, -12.24765755336480666 ) ) ;
#11277=ORIENTED_EDGE ( 'NONE', *, *, #4375, .T. ) ;
#11278=CARTESIAN_POINT ( 'NONE',  ( -1.071796769724486564, -27.26906051463638647, -7.688987169802764754 ) ) ;
#11281=CARTESIAN_POINT ( 'NONE',  ( 4.243569643749996345, -25.02533654799221097, -7.186914330003371099 ) ) ;
#11282=EDGE_CURVE ( 'NONE', #8773, #9873, #825, .T. ) ;
#11286=CARTESIAN_POINT ( 'NONE',  ( -4.000000000000004441, -25.91569448259783215, -8.703649444160298287 ) ) ;
#11287=CARTESIAN_POINT ( 'NONE',  ( 0.000000000000000000, 5.977523610840987267, 32.81826849749789687 ) ) ;
#11288=EDGE_CURVE ( 'NONE', #13336, #451, #143, .T. ) ;
#11289=CARTESIAN_POINT ( 'NONE',  ( -5.577813053751546416E-15, -28.99977223862889275, -10.16069966866791141 ) ) ;
#11292=CARTESIAN_POINT ( 'NONE',  ( 4.713407268011036227E-15, -22.64946367594241039, -16.11794214931127556 ) ) ;
#11295=CARTESIAN_POINT ( 'NONE',  ( -1.999999999999996225, -20.41198976004415044, -10.90933928264438890 ) ) ;
#11301=( BOUNDED_CURVE ( )  B_SPLINE_CURVE ( 2, ( #8502, #1660, #15660, #365, #3143, #13053, #14268, #5645, #14080 ),
 .UNSPECIFIED., .F., .F. ) 
 B_SPLINE_CURVE_WITH_KNOTS ( ( 3, 2, 2, 2, 3 ),
 ( 0.8706896551724138122, 0.8735632183908046411, 0.8793103448275861878, 0.8850574712643678454, 0.8879310344827586743 ),
 .UNSPECIFIED. ) 
 CURVE ( )  GEOMETRIC_REPRESENTATION_ITEM ( )  RATIONAL_B_SPLINE_CURVE ( ( 0.9330127018922194093, 0.9330127018922194093, 1.000000000000000000, 0.8660254037844387076, 1.000000000000000000, 0.8660254037844387076, 1.000000000000000000, 0.9330127018922180770, 0.9330127018922194093 ) ) 
 REPRESENTATION_ITEM ( '' )  );
#11302=CARTESIAN_POINT ( 'NONE',  ( -9.566989785610495289, -9.974423619177718692, -0.6215033074179308059 ) ) ;
#11303=CARTESIAN_POINT ( 'NONE',  ( 4.243569643750003451, -21.19427629940971869, -10.25857349556407527 ) ) ;
#11306=CARTESIAN_POINT ( 'NONE',  ( -2.000000000000005773, -26.06573248371572760, -6.904766962853115864 ) ) ;
#11313=CIRCLE ( 'NONE', #3344, 2.000000000000001776 ) ;
#11315=ORIENTED_EDGE ( 'NONE', *, *, #103, .T. ) ;
#11316=AXIS2_PLACEMENT_3D ( 'NONE', #14747, #9069, #7490 ) ;
#11318=CARTESIAN_POINT ( 'NONE',  ( 4.730628863548789710E-15, -18.36998600877478438, -10.49655905817405355 ) ) ;
#11323=CARTESIAN_POINT ( 'NONE',  ( 4.730628863548789710E-15, -18.14414028696156933, -10.17401794073526311 ) ) ;
#11329=( BOUNDED_CURVE ( )  B_SPLINE_CURVE ( 2, ( #10012, #14294, #1596, #7229, #6962, #4460, #1330, #7049, #8359 ),
 .UNSPECIFIED., .F., .T. ) 
 B_SPLINE_CURVE_WITH_KNOTS ( ( 3, 2, 2, 2, 3 ),
 ( 0.7327586206896552490, 0.7356321839080459668, 0.7413793103448276245, 0.7471264367816091712, 0.7500000000000000000 ),
 .UNSPECIFIED. ) 
 CURVE ( )  GEOMETRIC_REPRESENTATION_ITEM ( )  RATIONAL_B_SPLINE_CURVE ( ( 0.9330127018922194093, 0.9330127018922206306, 1.000000000000000000, 0.8660254037844387076, 1.000000000000000000, 0.8660254037844387076, 1.000000000000000000, 0.9330127018922194093, 0.9330127018922194093 ) ) 
 REPRESENTATION_ITEM ( '' )  );
#11330=CARTESIAN_POINT ( 'NONE',  ( 4.730628863548789710E-15, -16.56322023426900714, -7.916230118663721171 ) ) ;
#11332=ORIENTED_EDGE ( 'NONE', *, *, #9430, .T. ) ;
#11334=CARTESIAN_POINT ( 'NONE',  ( 3.579096709490575479E-14, -26.67678767140717966, -6.843133889297480899 ) ) ;
#11340=ORIENTED_EDGE ( 'NONE', *, *, #8693, .T. ) ;
#11346=CARTESIAN_POINT ( 'NONE',  ( -4.243569643750000786, -25.41665915365029704, -12.01727104090852905 ) ) ;
#11351=CARTESIAN_POINT ( 'NONE',  ( -2.121784821874996396, -21.67493339405068653, -13.08076802302275077 ) ) ;
#11354=CARTESIAN_POINT ( 'NONE',  ( -3.999999999999997335, -18.30357054373476444, -5.885045627956057679 ) ) ;
#11357=EDGE_CURVE ( 'NONE', #4590, #3584, #6910, .T. ) ;
#11358=CYLINDRICAL_SURFACE ( 'NONE', #14898, 4.000000000000000000 ) ;
#11359=CARTESIAN_POINT ( 'NONE',  ( -3.999999999999997335, -21.14277390367241694, -9.939848247186583663 ) ) ;
#11362=CARTESIAN_POINT ( 'NONE',  ( 2.121784821875004390, -21.75021530132177006, -13.18828172883567973 ) ) ;
#11365=CARTESIAN_POINT ( 'NONE',  ( 0.000000000000000000, 5.977523610840987267, 32.81826849749789687 ) ) ;
#11367=CARTESIAN_POINT ( 'NONE',  ( 4.000000000000003553, -18.13149761282945605, -5.639300014669354155 ) ) ;
#11368=PLANE ( 'NONE',  #11411 ) ;
#11370=CARTESIAN_POINT ( 'NONE',  ( 3.999999999999996447, -28.08811523457247006, -11.80618781089809488 ) ) ;
#11371=CARTESIAN_POINT ( 'NONE',  ( -2.121784821874996396, -18.86799370865777803, -9.072042706283481195 ) ) ;
#11374=CARTESIAN_POINT ( 'NONE',  ( 1.533898589781675205E-14, -27.96733465319702105, -8.686225988947720467 ) ) ;
#11382=CARTESIAN_POINT ( 'NONE',  ( 4.000000000000003553, -23.80990433270476458, -13.74890525313040612 ) ) ;
#11385=CARTESIAN_POINT ( 'NONE',  ( 4.000000000000000888, -23.59376154151967953, -9.413903449649181354 ) ) ;
#11387=DIRECTION ( 'NONE',  ( -0.000000000000000000, -0.5735764363510414965, -0.8191520442889950182 ) ) ;
#11389=CARTESIAN_POINT ( 'NONE',  ( 9.324435358932730011, -9.992494772396325331, -2.158019202327493336 ) ) ;
#11390=CARTESIAN_POINT ( 'NONE',  ( -4.243569643750000786, -22.57745579371264455, -7.962468421678005726 ) ) ;
#11398=CARTESIAN_POINT ( 'NONE',  ( -1.999999999999996225, -23.31572046977624169, -15.05629650786418772 ) ) ;
#11402=CARTESIAN_POINT ( 'NONE',  ( -4.243569643749997233, -20.33391164488314828, -9.029845429130588741 ) ) ;
#11408=( BOUNDED_CURVE ( )  B_SPLINE_CURVE ( 2, ( #8809, #5849, #11495, #17472, #17190, #4463, #12985, #299, #14490 ),
 .UNSPECIFIED., .F., .T. ) 
 B_SPLINE_CURVE_WITH_KNOTS ( ( 3, 2, 2, 2, 3 ),
 ( 0.07758620689655172653, 0.08045977011494252762, 0.08620689655172414367, 0.09195402298850574585, 0.09482758620689656082 ),
 .UNSPECIFIED. ) 
 CURVE ( )  GEOMETRIC_REPRESENTATION_ITEM ( )  RATIONAL_B_SPLINE_CURVE ( ( 0.9330127018922194093, 0.9330127018922194093, 1.000000000000000000, 0.8660254037844387076, 1.000000000000000000, 0.8660254037844387076, 1.000000000000000000, 0.9330127018922191873, 0.9330127018922194093 ) ) 
 REPRESENTATION_ITEM ( '' )  );
#11409=CARTESIAN_POINT ( 'NONE',  ( 2.121784821875004390, -19.94344952681598926, -10.60795278932534558 ) ) ;
#11410=EDGE_CURVE ( 'NONE', #7842, #16544, #17039, .T. ) ;
#11411=AXIS2_PLACEMENT_3D ( 'NONE', #8585, #17058, #15484 ) ;
#11412=CARTESIAN_POINT ( 'NONE',  ( -2.649389826664908298, -10.00000000000000178, -4.175485738723567763 ) ) ;
#11413=CARTESIAN_POINT ( 'NONE',  ( -5.577813053751546416E-15, -23.90211166126395881, -2.880485876056233518 ) ) ;
#11414=CARTESIAN_POINT ( 'NONE',  ( -8.500000000000005329, 10.00000000000000000, -20.49999999999999645 ) ) ;
#11415=CARTESIAN_POINT ( 'NONE',  ( 2.121784821874994176, -23.43695996064828435, -2.782732417011581028 ) ) ;
#11419=ORIENTED_EDGE ( 'NONE', *, *, #17831, .F. ) ;
#11427=CARTESIAN_POINT ( 'NONE',  ( 4.730628863548789710E-15, -16.33737451245578498, -7.593689001224929847 ) ) ;
#11429=CARTESIAN_POINT ( 'NONE',  ( -2.000000000000005773, -22.64578298126770051, -2.020572897773216692 ) ) ;
#11432=CARTESIAN_POINT ( 'NONE',  ( 4.243569643750003451, -24.29158905570533733, -14.68199453472465521 ) ) ;
#11433=FACE_OUTER_BOUND ( 'NONE', #11710, .T. ) ;
#11436=CARTESIAN_POINT ( 'NONE',  ( 2.121784821875004390, -22.23417041949295481, -13.87944126620451790 ) ) ;
#11437=EDGE_CURVE ( 'NONE', #4809, #13013, #17734, .T. ) ;
#11439=CARTESIAN_POINT ( 'NONE',  ( 1.999999999999994449, -22.66729209833581749, -2.051291100440815640 ) ) ;
#11440=EDGE_CURVE ( 'NONE', #4695, #18119, #7290, .T. ) ;
#11442=VERTEX_POINT ( 'NONE', #16188 ) ;
#11449=VERTEX_POINT ( 'NONE', #11718 ) ;
#11450=CARTESIAN_POINT ( 'NONE',  ( 2.121784821875004390, -21.23399650860583066, -12.45104488897558248 ) ) ;
#11452=EDGE_LOOP ( 'NONE', ( #5549, #6172, #2863, #16060, #4612, #647 ) ) ;
#11455=CARTESIAN_POINT ( 'NONE',  ( 3.579096709490575479E-14, -24.61191250054342916, -3.894186529857098567 ) ) ;
#11458=VECTOR ( 'NONE', #2284, 1000.000000000000000 ) ;
#11460=CARTESIAN_POINT ( 'NONE',  ( -4.243569643750005227, -22.78838844622314497, -3.992221357276296345 ) ) ;
#11462=EDGE_CURVE ( 'NONE', #12907, #16218, #5576, .T. ) ;
#11463=CARTESIAN_POINT ( 'NONE',  ( 4.000000000000000888, -23.07754274880374368, -8.676666609789087659 ) ) ;
#11468=CARTESIAN_POINT ( 'NONE',  ( -1.999999999999996225, -22.99308372362383679, -14.59552348194486626 ) ) ;
#11475=AXIS2_PLACEMENT_3D ( 'NONE', #1584, #11387, #14188 ) ;
#11477=CARTESIAN_POINT ( 'NONE',  ( -4.000000000000004441, -25.33494834008745755, -7.874257998310924656 ) ) ;
#11478=ORIENTED_EDGE ( 'NONE', *, *, #15984, .T. ) ;
#11481=CARTESIAN_POINT ( 'NONE',  ( -4.968818199243726141, -10.12411597883879999, -1.720161685108341221 ) ) ;
#11482=CARTESIAN_POINT ( 'NONE',  ( 4.243569643750003451, -19.64561992126190049, -8.046862975983790633 ) ) ;
#11486=ORIENTED_EDGE ( 'NONE', *, *, #2081, .F. ) ;
#11493=EDGE_LOOP ( 'NONE', ( #15205, #82, #3967, #1415, #5952, #17110 ) ) ;
#11495=CARTESIAN_POINT ( 'NONE',  ( -1.999999999999996225, -23.57382986613421139, -15.42491492779423723 ) ) ;
#11496=CARTESIAN_POINT ( 'NONE',  ( 4.243569643749996345, -24.99307287344746342, -7.140837027512114688 ) ) ;
#11499=CARTESIAN_POINT ( 'NONE',  ( 0.000000000000000000, -2.372474330222551941, 20.89323558166710626 ) ) ;
#11503=CARTESIAN_POINT ( 'NONE',  ( 4.730628863548789710E-15, -19.17657787239344458, -11.64849162045545583 ) ) ;
#11504=CARTESIAN_POINT ( 'NONE',  ( -4.000000000000003553, -2.343145750507612313, 16.84997118393183513 ) ) ;
#11505=ADVANCED_FACE ( 'NONE', ( #8942 ), #17413, .F. ) ;
#11506=CARTESIAN_POINT ( 'NONE',  ( -5.679766210340590149, -14.60833734475422752, -5.139172057957636319 ) ) ;
#11509=AXIS2_PLACEMENT_3D ( 'NONE', #16659, #2741, #6805 ) ;
#11511=CARTESIAN_POINT ( 'NONE',  ( -4.243569643749997233, -18.52714587037736393, -6.449516489620252813 ) ) ;
#11519=CARTESIAN_POINT ( 'NONE',  ( -4.243569643750000786, -26.44909673908217584, -13.49174472062871999 ) ) ;
#11522=DIRECTION ( 'NONE',  ( 0.000000000000000000, 0.8191520442889952403, -0.5735764363510413855 ) ) ;
#11523=ORIENTED_EDGE ( 'NONE', *, *, #778, .T. ) ;
#11524=CARTESIAN_POINT ( 'NONE',  ( 4.730628863548789710E-15, -15.82115571973984736, -6.856452161364833486 ) ) ;
#11526=CARTESIAN_POINT ( 'NONE',  ( -4.000000000000004441, -21.72141679107589596, -2.713600119290256352 ) ) ;
#11529=CARTESIAN_POINT ( 'NONE',  ( -4.243569643749998122, -23.43122440117877048, -13.45326646829116157 ) ) ;
#11533=CARTESIAN_POINT ( 'NONE',  ( -4.243569643750000786, -25.41665915365029704, -12.01727104090852905 ) ) ;
#11535=CARTESIAN_POINT ( 'NONE',  ( 1.999999999999994449, -23.44162028740971948, -3.157146360230959292 ) ) ;
#11540=DIRECTION ( 'NONE',  ( -0.000000000000000000, -0.5735764363510414965, -0.8191520442889950182 ) ) ;
#11542=CARTESIAN_POINT ( 'NONE',  ( 4.299564228933482956E-15, -19.80093457235270549, -10.97097235620001854 ) ) ;
#11543=CIRCLE ( 'NONE', #3571, 4.000000000000000000 ) ;
#11545=ORIENTED_EDGE ( 'NONE', *, *, #8787, .T. ) ;
#11546=CARTESIAN_POINT ( 'NONE',  ( -5.330712181944246111E-15, -28.62395502770104017, -8.054784027183542250 ) ) ;
#11551=CARTESIAN_POINT ( 'NONE',  ( -4.243569643749997233, -23.46348807572352158, -13.49934377078241710 ) ) ;
#11556=CARTESIAN_POINT ( 'NONE',  ( 4.730628863548789710E-15, -17.36981209788766378, -9.068162680945119902 ) ) ;
#11558=CARTESIAN_POINT ( 'NONE',  ( -8.999999999999996447, -10.00000000000000000, -30.00000000000000000 ) ) ;
#11559=VERTEX_POINT ( 'NONE', #14524 ) ;
#11561=CARTESIAN_POINT ( 'NONE',  ( 3.579096709490575479E-14, -24.93454924669583406, -4.354959555776423130 ) ) ;
#11562=CARTESIAN_POINT ( 'NONE',  ( 3.604268994871579590, -24.91053875026183562, -15.69445619563776617 ) ) ;
#11569=CARTESIAN_POINT ( 'NONE',  ( -3.999999999999997335, -21.85257474295189084, -10.95354890098744605 ) ) ;
#11570=ORIENTED_EDGE ( 'NONE', *, *, #8861, .T. ) ;
#11575=CARTESIAN_POINT ( 'NONE',  ( -5.348698796015789014, -10.20673381021435411, -1.142656398237904991 ) ) ;
#11577=CARTESIAN_POINT ( 'NONE',  ( 4.243569643750000786, -22.19029169917569888, -7.409540791782929681 ) ) ;
#11582=ORIENTED_EDGE ( 'NONE', *, *, #9219, .F. ) ;
#11585=CARTESIAN_POINT ( 'NONE',  ( -1.071796769724496334, -29.33393568550013342, -10.63793452924315375 ) ) ;
#11586=CARTESIAN_POINT ( 'NONE',  ( 0.000000000000000000, -10.00099999999999767, 0.000000000000000000 ) ) ;
#11587=CARTESIAN_POINT ( 'NONE',  ( -4.648177544792955347E-16, -29.77410042770280185, -11.26655492845805107 ) ) ;
#11591=CARTESIAN_POINT ( 'NONE',  ( -5.330712181944245322E-15, -26.78492557865051538, -5.428377785181952575 ) ) ;
#11596=CARTESIAN_POINT ( 'NONE',  ( 4.243569643750000786, -27.12663390452184942, -14.45936807294509308 ) ) ;
#11597=CARTESIAN_POINT ( 'NONE',  ( 2.000000000000004441, -24.32664893814001417, -16.50005198491677305 ) ) ;
#11599=CARTESIAN_POINT ( 'NONE',  ( 4.243569643749996345, -25.02533654799221097, -7.186914330003371099 ) ) ;
#11602=CARTESIAN_POINT ( 'NONE',  ( -4.757769075324985941, -14.90261145393141895, -7.125238870421979342 ) ) ;
#11606=DIRECTION ( 'NONE',  ( 0.000000000000000000, -0.5735764363510414965, -0.8191520442889950182 ) ) ;
#11608=CARTESIAN_POINT ( 'NONE',  ( -4.243569643750005227, -22.49801537532042062, -3.577525634854993086 ) ) ;
#11614=DIRECTION ( 'NONE',  ( 0.000000000000000000, 0.000000000000000000, 1.000000000000000000 ) ) ;
#11616=CARTESIAN_POINT ( 'NONE',  ( 3.049298716198209913, -9.999999999999397815, -3.862741893372411806 ) ) ;
#11621=CARTESIAN_POINT ( 'NONE',  ( -4.243569643750000786, -26.22325101726895369, -13.16920360318992955 ) ) ;
#11622=CARTESIAN_POINT ( 'NONE',  ( -4.000000000000004441, -26.94813206802970740, -10.17812312388048746 ) ) ;
#11623=CARTESIAN_POINT ( 'NONE',  ( 4.243569643750003451, -23.51726086663143533, -13.57613927493450667 ) ) ;
#11627=FACE_OUTER_BOUND ( 'NONE', #1940, .T. ) ;
#11628=CARTESIAN_POINT ( 'NONE',  ( -4.243569643750005227, -27.40209390612182716, -10.58127561352589829 ) ) ;
#11629=CARTESIAN_POINT ( 'NONE',  ( 4.000000000000000888, -21.85152311680833748, -6.925729116128124474 ) ) ;
#11630=CARTESIAN_POINT ( 'NONE',  ( -2.000000000000005773, -22.96841972742010540, -2.481345923692543920 ) ) ;
#11633=VERTEX_POINT ( 'NONE', #11815 ) ;
#11640=CARTESIAN_POINT ( 'NONE',  ( -2.121784821875005722, -27.38388281328888141, -8.419522421775232246 ) ) ;
#11642=ORIENTED_EDGE ( 'NONE', *, *, #7961, .T. ) ;
#11644=CARTESIAN_POINT ( 'NONE',  ( 2.000000000000004441, -18.64824221826470207, -8.390446746455726412 ) ) ;
#11645=ADVANCED_FACE ( 'NONE', ( #11627 ), #6737, .F. ) ;
#11646=LINE ( 'NONE', #14443, #15090 ) ;
#11648=CARTESIAN_POINT ( 'NONE',  ( -5.330712181944245322E-15, -30.17261140584885126, -10.26649454676382867 ) ) ;
#11651=CARTESIAN_POINT ( 'NONE',  ( 4.000000000000000888, -23.65828889131411827, -9.506058055638460402 ) ) ;
#11653=CARTESIAN_POINT ( 'NONE',  ( 2.121784821875004390, -17.87857435595223876, -7.659005429884962801 ) ) ;
#11660=DIRECTION ( 'NONE',  ( 0.000000000000000000, -0.000000000000000000, 1.000000000000000000 ) ) ;
#11667=CARTESIAN_POINT ( 'NONE',  ( 2.000000000000004441, -19.42257040733860762, -9.496302006245869620 ) ) ;
#11671=CARTESIAN_POINT ( 'NONE',  ( -7.496931198983602052, -13.00340931249926157, 5.026614306467389603 ) ) ;
#11672=CARTESIAN_POINT ( 'NONE',  ( -4.243569643750000786, -21.54501820828076930, -6.487994741957813005 ) ) ;
#11677=CARTESIAN_POINT ( 'NONE',  ( -1.071796769724486786, -19.98298991819740422, -11.23097433548487700 ) ) ;
#11679=CARTESIAN_POINT ( 'NONE',  ( -8.999999999999996447, -10.00000000000000000, 15.14468620625656925 ) ) ;
#11680=CARTESIAN_POINT ( 'NONE',  ( -4.000000000000000888, -26.56201959963631509, -13.65301527884473387 ) ) ;
#11685=CARTESIAN_POINT ( 'NONE',  ( 4.243569643749996345, -22.92819770258371292, -4.191889668071731911 ) ) ;
#11687=( BOUNDED_CURVE ( )  B_SPLINE_CURVE ( 2, ( #12584, #3882, #5456, #16609, #8324, #2599, #15393, #11278, #7009 ),
 .UNSPECIFIED., .F., .F. ) 
 B_SPLINE_CURVE_WITH_KNOTS ( ( 3, 2, 2, 2, 3 ),
 ( 0.3879310344827586188, 0.3908045977011494476, 0.3965517241379310498, 0.4022988505747126520, 0.4051724137931034808 ),
 .UNSPECIFIED. ) 
 CURVE ( )  GEOMETRIC_REPRESENTATION_ITEM ( )  RATIONAL_B_SPLINE_CURVE ( ( 0.9330127018922194093, 0.9330127018922194093, 1.000000000000000000, 0.8660254037844387076, 1.000000000000000000, 0.8660254037844387076, 1.000000000000000000, 0.9330127018922187432, 0.9330127018922194093 ) ) 
 REPRESENTATION_ITEM ( '' )  );
#11689=CARTESIAN_POINT ( 'NONE',  ( -4.243569643749998122, -25.01214445387132912, -15.71105429036270351 ) ) ;
#11690=CARTESIAN_POINT ( 'NONE',  ( 3.999999999999996447, -28.60433402728840946, -12.54342465075819035 ) ) ;
#11691=EDGE_CURVE ( 'NONE', #8670, #12774, #15625, .T. ) ;
#11692=CARTESIAN_POINT ( 'NONE',  ( -4.243569643749997233, -20.10806592306992613, -8.707304311691796528 ) ) ;
#11696=CARTESIAN_POINT ( 'NONE',  ( -2.000000000000005773, -27.54986151206910350, -9.024322876444124120 ) ) ;
#11697=ORIENTED_EDGE ( 'NONE', *, *, #5157, .T. ) ;
#11699=CARTESIAN_POINT ( 'NONE',  ( -5.330712181944245322E-15, -23.68761282235488963, -1.004956746021377967 ) ) ;
#11700=DIRECTION ( 'NONE',  ( 0.000000000000000000, 0.000000000000000000, 1.000000000000000000 ) ) ;
#11701=ORIENTED_EDGE ( 'NONE', *, *, #13795, .F. ) ;
#11704=CARTESIAN_POINT ( 'NONE',  ( -2.121784821875005722, -28.38405672417600911, -9.847918799004165891 ) ) ;
#11705=DIRECTION ( 'NONE',  ( 1.049727191973305394E-16, 0.5150380737757255245, -0.8571673013836856869 ) ) ;
#11706=AXIS2_PLACEMENT_3D ( 'NONE', #11499, #9011, #11782 ) ;
#11709=CARTESIAN_POINT ( 'NONE',  ( 7.003832385457680054, -10.00000000000000178, -7.945690313593527954 ) ) ;
#11710=EDGE_LOOP ( 'NONE', ( #8080, #5818, #3411 ) ) ;
#11712=CARTESIAN_POINT ( 'NONE',  ( 4.730628863548789710E-15, -22.27389062868906677, -16.07191265961602511 ) ) ;
#11714=CARTESIAN_POINT ( 'NONE',  ( -2.121784821874996396, -22.96548037584052793, -14.92386012267298945 ) ) ;
#11715=VECTOR ( 'NONE', #2904, 1000.000000000000000 ) ;
#11716=CYLINDRICAL_SURFACE ( 'NONE', #5810, 4.000000000000000000 ) ;
#11718=CARTESIAN_POINT ( 'NONE',  ( 3.579096709490575479E-14, -24.61191250054342916, -3.894186529857098567 ) ) ;
#11720=CARTESIAN_POINT ( 'NONE',  ( -4.243569643750000786, -23.86800277550248950, -9.805560521328242629 ) ) ;
#11726=CARTESIAN_POINT ( 'NONE',  ( 8.500000000000019540, 0.000000000000000000, 18.49999999999998934 ) ) ;
#11727=CARTESIAN_POINT ( 'NONE',  ( -4.000000000000004441, -27.46435086074563969, -10.91535996374058293 ) ) ;
#11728=CARTESIAN_POINT ( 'NONE',  ( 2.000000000000004441, -17.42222258626929943, -6.639509252794765892 ) ) ;
#11730=EDGE_LOOP ( 'NONE', ( #7579, #349 ) ) ;
#11731=CARTESIAN_POINT ( 'NONE',  ( 4.730628863548789710E-15, -20.20901545782531628, -13.12296530017564500 ) ) ;
#11733=AXIS2_PLACEMENT_3D ( 'NONE', #4583, #14711, #12922 ) ;
#11736=CARTESIAN_POINT ( 'NONE',  ( 4.000000000000000888, -20.04475734230255668, -4.345400176617791210 ) ) ;
#11737=CARTESIAN_POINT ( 'NONE',  ( 4.243569643750000786, -25.83608692273200802, -12.61627597329485440 ) ) ;
#11738=CARTESIAN_POINT ( 'NONE',  ( -4.000000000000004441, -27.20624146438767710, -10.54674154381053697 ) ) ;
#11740=CARTESIAN_POINT ( 'NONE',  ( 4.243569643750000786, -21.19011778828857118, -5.981144414553994260 ) ) ;
#11741=ORIENTED_EDGE ( 'NONE', *, *, #506, .T. ) ;
#11742=CARTESIAN_POINT ( 'NONE',  ( 2.610817454768295409, -22.11373505648317916, -1.875566028523329321 ) ) ;
#11744=CARTESIAN_POINT ( 'NONE',  ( 4.299564228933482956E-15, -19.99451661891623289, -11.24743617014079078 ) ) ;
#11745=LINE ( 'NONE', #1759, #7615 ) ;
#11747=AXIS2_PLACEMENT_3D ( 'NONE', #704, #6351, #7821 ) ;
#11748=ORIENTED_EDGE ( 'NONE', *, *, #10859, .T. ) ;
#11749=CARTESIAN_POINT ( 'NONE',  ( 3.999999999999996447, -26.08776741350315831, -8.949395057446990265 ) ) ;
#11755=EDGE_CURVE ( 'NONE', #9470, #1591, #5136, .T. ) ;
#11759=CARTESIAN_POINT ( 'NONE',  ( -4.000000000000000888, -21.65794106883490855, -6.649265300173826887 ) ) ;
#11765=CARTESIAN_POINT ( 'NONE',  ( 4.243569643749997233, -23.18630709894168263, -4.560508088001781424 ) ) ;
#11767=CARTESIAN_POINT ( 'NONE',  ( 3.999999999999996447, -21.89348972198121857, -2.959345732576948773 ) ) ;
#11768=ORIENTED_EDGE ( 'NONE', *, *, #11119, .F. ) ;
#11772=CYLINDRICAL_SURFACE ( 'NONE', #8632, 4.000000000000000000 ) ;
#11775=CIRCLE ( 'NONE', #8508, 2.000000000000001776 ) ;
#11779=CARTESIAN_POINT ( 'NONE',  ( -4.243569643750005227, -24.04667175346823527, -5.789236154435278614 ) ) ;
#11782=DIRECTION ( 'NONE',  ( 0.000000000000000000, 0.8191520442889952403, -0.5735764363510411634 ) ) ;
#11783=CARTESIAN_POINT ( 'NONE',  ( -5.279047395330986450E-15, -30.02288408040872625, -10.54300617450737043 ) ) ;
#11784=CARTESIAN_POINT ( 'NONE',  ( -4.243569643750000786, -21.57728188282551685, -6.534072044449069416 ) ) ;
#11788=CARTESIAN_POINT ( 'NONE',  ( -8.999999999999996447, -10.00000000000000178, -3.713574246709370641 ) ) ;
#11789=CARTESIAN_POINT ( 'NONE',  ( 1.071796769724494114, -23.61957486864662314, -16.42455588381737286 ) ) ;
#11793=( BOUNDED_CURVE ( )  B_SPLINE_CURVE ( 2, ( #9309, #3744, #3664, #13479, #13304, #9395, #14902, #792, #14983 ),
 .UNSPECIFIED., .F., .F. ) 
 B_SPLINE_CURVE_WITH_KNOTS ( ( 3, 2, 2, 2, 3 ),
 ( 0.1120689655172413812, 0.1149425287356321823, 0.1206896551724137984, 0.1264367816091954144, 0.1293103448275862155 ),
 .UNSPECIFIED. ) 
 CURVE ( )  GEOMETRIC_REPRESENTATION_ITEM ( )  RATIONAL_B_SPLINE_CURVE ( ( 0.9330127018922194093, 0.9330127018922194093, 1.000000000000000000, 0.8660254037844387076, 1.000000000000000000, 0.8660254037844387076, 1.000000000000000000, 0.9330127018922194093, 0.9330127018922194093 ) ) 
 REPRESENTATION_ITEM ( '' )  );
#11799=CARTESIAN_POINT ( 'NONE',  ( 4.243569643750003451, -23.51726086663143533, -13.57613927493450667 ) ) ;
#11803=DIRECTION ( 'NONE',  ( -0.000000000000000000, -0.5735764363510414965, -0.8191520442889950182 ) ) ;
#11804=ORIENTED_EDGE ( 'NONE', *, *, #13450, .T. ) ;
#11806=CARTESIAN_POINT ( 'NONE',  ( -2.121784821875005722, -28.67442979507872636, -10.26261452142547093 ) ) ;
#11810=CARTESIAN_POINT ( 'NONE',  ( 4.243569643750000786, -23.99705747368147968, -9.989869731293264721 ) ) ;
#11811=DIRECTION ( 'NONE',  ( -0.000000000000000000, -0.000000000000000000, -1.000000000000000000 ) ) ;
#11813=CARTESIAN_POINT ( 'NONE',  ( -8.500000000000005329, 0.000000000000000000, -18.49999999999999645 ) ) ;
#11815=CARTESIAN_POINT ( 'NONE',  ( -8.500000000000005329, -1.201721234452885367, -20.49999999999999645 ) ) ;
#11816=CARTESIAN_POINT ( 'NONE',  ( 2.121784821875004390, -20.42740464498717401, -11.29911232669418197 ) ) ;
#11817=CARTESIAN_POINT ( 'NONE',  ( 1.999999999999994449, -24.73216726919956443, -5.000238459881198416 ) ) ;
#11824=CARTESIAN_POINT ( 'NONE',  ( -4.000000000000004441, -27.20624146438767355, -10.54674154381053697 ) ) ;
#11826=CARTESIAN_POINT ( 'NONE',  ( 4.299564228933482956E-15, -17.92964144805248594, -8.298488810700408891 ) ) ;
#11828=( BOUNDED_SURFACE ( )  B_SPLINE_SURFACE ( 1, 2, ( 
 ( #7164, #12824, #16938, #15804, #3006, #10217, #3100, #17028, #15616, #8641, #320, #15897, #14319, #9945, #8461, #8732, #14406, #7071, #14511, #1617, #7250, #2917, #1529, #220, #12910, #18332, #5869, #8832, #14129, #13007, #11519, #17209, #6981, #1712, #4211, #9858, #2830, #4298, #16365, #604, #3651, #3566, #508, #14606, #10692, #9298, #16273, #2000, #4944, #11894, #17593, #13291, #5036, #9212, #10313, #12075, #6244, #1808, #2093, #6343, #17774, #8925, #4856, #1908, #10507, #17680, #7538, #14890, #13382, #7444, #16176, #6150, #13191, #11799, #13102, #17496, #416, #17399, #13472, #6054, #11704, #4761, #2187, #4663, #3473, #15996, #9117, #3289, #7721, #7815, #10413, #16092, #14796, #3384, #9025, #7626, #14702, #697, #11986, #10599, #783, #6430, #16551, #16737, #2367, #9573, #12350, #13936, #6878, #971, #15337, #3921, #12259, #875, #18137, #1244, #13750, #5494, #18225, #9658, #11140, #12169, #1060, #2274, #2548, #7903, #4014, #12536, #6520, #13651, #2458, #5314, #8088, #6790, #16830, #4101, #13558, #17860, #6695, #18041, #2636, #8277, #10966, #1149, #14977, #15252, #16648, #8179, #13839, #12445, #7997, #5124, #5405, #11056, #10781, #16454, #3735, #9386, #15063, #3827, #6616, #17946, #5218, #10871, #9478, #15153, #12892, #10101, #112, #8363, #14023, #5585, #4283, #11231, #15433, #17012, #8443, #2815, #12718, #15784, #22, #14387, #12986, #300, #18314, #5673, #8714, #15691, #16919, #2989, #15598, #11496, #9926, #4195, #9752, #2900, #1691, #4464, #7325, #12806, #5942, #11591, #14113, #7234, #1426, #17287, #8534, #199, #14205, #5765, #1334, #2730, #1510, #9842, #7053, #17191, #6966, #15518, #12624, #11318, #7144, #11402, #17094, #4366, #10016, #8621, #14298, #1599, #5850, #3081, #6127, #16160, #17377, #3269, #11970, #11779, #6321, #10295, #17566, #1979, #3544, #14870, #8906, #4924, #11874, #1888, #8811, #7701, #9188, #3363, #13453, #7796, #17662, #765, #1790, #9008, #10197, #10486, #15876, #10575, #2164, #14491, #14583, #10390, #13267, #16068, #14775, #6410, #12055, #3173, #7422, #14683, #7606, #16251, #4557, #584, #9093, #13079, #4838, #6225, #3452, #2072, #13362, #15975, #397, #674, #6033, #11685, #4642, #7519, #13171, #485, #17473, #4742, #2255, #16339, #7880, #6676, #9547, #2525, #18112, #8061, #3631, #9280, #13537, #12237, #854, #5013, #6587, #16437, #10762, #2347, #5382, #7978, #3987, #2614, #8254, #6500, #13631, #16714, #5289, #12144, #10942, #5197, #1128, #17925, #17837, #17752, #10848, #9636, #12421, #15314, #2435, #13912, #1220, #3715, #15225, #9365, #6857, #16524, #8155, #3803, #13724, #14960, #10669, #9458, #5101, #15041, #6764 ),
 ( #13818, #15131, #943, #11031, #1035, #12329, #18015, #16625, #3900, #12691, #15496, #13997, #14535, #3220, #6944, #1934, #1486, #7120, #2793, #8424, #5742, #14086, #18206, #1398, #6074, #1312, #13126, #11292, #7026, #14631, #68, #12511, #5650, #15575, #5558, #8952, #16984, #5470, #1831, #11207, #12597, #3310, #11115, #8854, #4261, #15921, #9904, #2876, #8506, #16018, #7467, #2706, #4689, #14179, #16804, #12781, #17069, #10338, #18285, #89, #16896, #11382, #10243, #4172, #435, #4593, #4074, #11727, #9815, #17422, #9728, #15411, #8338, #7557, #529, #14723, #13213, #6176, #10436, #11824, #17521, #4783, #16113, #3405, #9047, #12592, #14078, #12414, #8501, #4067, #2519, #14173, #12504, #11024, #16798, #9717, #15404, #8418, #18197, #6937, #15307, #2700, #8331, #5552, #8147, #5463, #4254, #7782, #12321, #13992, #1305, #18279, #11200, #16889, #9541, #4166, #3892, #9630, #6669, #2606, #8245, #13811, #15569, #9810, #18010, #15491, #2788, #1392, #7018, #12685, #15218, #5644, #1121, #13906, #5280, #1214, #6850, #6756, #2869, #11286, #16979, #11108, #9898, #16618, #10936, #18106, #5375, #16706, #3980, #12207, #7763, #12024, #5072, #9335, #11940, #13599, #17893, #5165, #17538, #4893, #7943, #14933, #16133, #2225, #14836, #10728, #3512, #4805, #8975, #16217, #913, #3689, #6557, #17717, #10819, #16494, #7665, #6466, #645, #14649, #13423, #12115, #737, #4984, #13232, #1950, #9158, #10455, #13332, #16404, #7576, #14741, #549, #2040, #6193, #3423, #9064, #17633, #10638, #10542, #7852, #6286, #2133, #15012, #6380, #2309, #16311, #3597, #9248, #11842, #13506, #821, #17810, #11087, #1095, #8035, #6914, #8394, #2583, #12659, #6997, #16864, #18350, #1008, #8215, #9424, #9692, #15100, #11173, #14055, #13693, #2496, #9611, #12474, #15283, #13966, #5621, #1366, #2402, #6647, #13880, #6826, #4140, #9787, #1190, #8310, #11265, #16772, #18171, #5440, #4041, #15376, #1281, #3772, #10913, #2675, #16588, #12570, #18258, #3867, #15469, #5528, #12296, #2764, #8126, #9514, #15194, #17986, #13784, #5256, #6734, #12391, #18079, #5349, #11002, #16680, #3958, #14336, #4233, #5887, #57, #4501, #5978, #4314, #430, #1634, #12755, #6068, #4408, #2935, #8658, #7271, #12927, #339, #10049, #17227, #7183, #240, #11535, #15823, #5714, #15726, #14528, #10237, #9875, #10142, #3119, #8753, #14427, #1730, #1460, #7365, #14147, #1546, #16954, #12842, #146, #11354, #7461, #13025, #11630, #17130, #3025, #8476, #17324, #4588, #1824, #15914, #9961, #5796, #3212, #17043, #8848, #13121, #11439, #15635, #15550, #2846, #8570, #7090, #14242, #710, #2015, #14717, #4959, #7642, #17416, #621, #5049 ) ),
 .UNSPECIFIED., .F., .F., .F. ) 
 B_SPLINE_SURFACE_WITH_KNOTS ( ( 2, 2 ),
 ( 3, 2, 2, 2, 2, 2, 2, 2, 2, 2, 2, 2, 2, 2, 2, 2, 2, 2, 2, 2, 2, 2, 2, 2, 2, 2, 2, 2, 2, 2, 2, 2, 2, 2, 2, 2, 2, 2, 2, 2, 2, 2, 2, 2, 2, 2, 2, 2, 2, 2, 2, 2, 2, 2, 2, 2, 2, 2, 2, 2, 2, 2, 2, 2, 2, 2, 2, 2, 2, 2, 2, 2, 2, 2, 2, 2, 2, 2, 2, 2, 2, 2, 2, 2, 2, 2, 2, 2, 2, 2, 2, 2, 2, 2, 2, 2, 2, 2, 2, 2, 2, 2, 2, 2, 2, 2, 2, 2, 2, 2, 2, 2, 2, 2, 2, 2, 2, 2, 2, 2, 2, 2, 2, 2, 2, 2, 2, 2, 2, 2, 2, 2, 2, 2, 2, 2, 2, 2, 2, 2, 2, 2, 2, 2, 2, 2, 2, 2, 2, 2, 2, 2, 2, 2, 2, 2, 2, 2, 2, 2, 2, 2, 2, 2, 2, 2, 2, 2, 2, 2, 2, 2, 2, 2, 3 ),
 ( 0.000000000000000000, 1.000000000000000000 ),
 ( 0.000000000000000000, 0.005747126436781609116, 0.01149425287356321823, 0.01724137931034482735, 0.02298850574712643646, 0.02873563218390804558, 0.03448275862068965469, 0.04022988505747126381, 0.04597701149425287293, 0.05172413793103448204, 0.05747126436781609116, 0.06321839080459770721, 0.06896551724137930939, 0.07471264367816092544, 0.08045977011494252762, 0.08620689655172414367, 0.09195402298850574585, 0.09770114942528736190, 0.1034482758620689641, 0.1091954022988505801, 0.1149425287356321823, 0.1206896551724137984, 0.1264367816091954144, 0.1321839080459770166, 0.1379310344827586188, 0.1436781609195402210, 0.1494252873563218509, 0.1551724137931034531, 0.1609195402298850552, 0.1666666666666666574, 0.1724137931034482873, 0.1781609195402298895, 0.1839080459770114917, 0.1896551724137930939, 0.1954022988505747238, 0.2011494252873563260, 0.2068965517241379282, 0.2126436781609195303, 0.2183908045977011603, 0.2241379310344827624, 0.2298850574712643646, 0.2356321839080459668, 0.2413793103448275967, 0.2471264367816091989, 0.2528735632183908288, 0.2586206896551724310, 0.2643678160919540332, 0.2701149425287356354, 0.2758620689655172376, 0.2816091954022988397, 0.2873563218390804419, 0.2931034482758620441, 0.2988505747126437018, 0.3045977011494253039, 0.3103448275862069061, 0.3160919540229885083, 0.3218390804597701105, 0.3275862068965517127, 0.3333333333333333148, 0.3390804597701149170, 0.3448275862068965747, 0.3505747126436781769, 0.3563218390804597790, 0.3620689655172413812, 0.3678160919540229834, 0.3735632183908045856, 0.3793103448275861878, 0.3850574712643677899, 0.3908045977011494476, 0.3965517241379310498, 0.4022988505747126520, 0.4080459770114942541, 0.4137931034482758563, 0.4195402298850574585, 0.4252873563218390607, 0.4310344827586206629, 0.4367816091954023205, 0.4425287356321839227, 0.4482758620689655249, 0.4540229885057471271, 0.4597701149425287293, 0.4655172413793103314, 0.4712643678160919336, 0.4770114942528735358, 0.4827586206896551935, 0.4885057471264367956, 0.4942528735632183978, 0.5000000000000000000, 0.5057471264367816577, 0.5114942528735632044, 0.5172413793103448620, 0.5229885057471264087, 0.5287356321839080664, 0.5344827586206896131, 0.5402298850574712707, 0.5459770114942529284, 0.5517241379310344751, 0.5574712643678161328, 0.5632183908045976795, 0.5689655172413793371, 0.5747126436781608838, 0.5804597701149425415, 0.5862068965517240882, 0.5919540229885057459, 0.5977011494252874035, 0.6034482758620689502, 0.6091954022988506079, 0.6149425287356321546, 0.6206896551724138122, 0.6264367816091953589, 0.6321839080459770166, 0.6379310344827586743, 0.6436781609195402210, 0.6494252873563218786, 0.6551724137931034253, 0.6609195402298850830, 0.6666666666666666297, 0.6724137931034482873, 0.6781609195402298340, 0.6839080459770114917, 0.6896551724137931494, 0.6954022988505746961, 0.7011494252873563537, 0.7068965517241379004, 0.7126436781609195581, 0.7183908045977011048, 0.7241379310344827624, 0.7298850574712644201, 0.7356321839080459668, 0.7413793103448276245, 0.7471264367816091712, 0.7528735632183908288, 0.7586206896551723755, 0.7643678160919540332, 0.7701149425287355799, 0.7758620689655172376, 0.7816091954022988952, 0.7873563218390804419, 0.7931034482758620996, 0.7988505747126436463, 0.8045977011494253039, 0.8103448275862068506, 0.8160919540229885083, 0.8218390804597701660, 0.8275862068965517127, 0.8333333333333333703, 0.8390804597701149170, 0.8448275862068965747, 0.8505747126436781214, 0.8563218390804597790, 0.8620689655172413257, 0.8678160919540229834, 0.8735632183908046411, 0.8793103448275861878, 0.8850574712643678454, 0.8908045977011493921, 0.8965517241379310498, 0.9022988505747125965, 0.9080459770114942541, 0.9137931034482759118, 0.9195402298850574585, 0.9252873563218391162, 0.9310344827586206629, 0.9367816091954023205, 0.9425287356321838672, 0.9482758620689655249, 0.9540229885057470716, 0.9597701149425287293, 0.9655172413793103869, 0.9712643678160919336, 0.9770114942528735913, 0.9827586206896551380, 0.9885057471264367956, 0.9942528735632183423, 0.9961881922148684287 ),
 .UNSPECIFIED. ) 
 GEOMETRIC_REPRESENTATION_ITEM ( )  RATIONAL_B_SPLINE_SURFACE ( (
 ( 1.000000000000000000, 0.8660254037844387076, 1.000000000000000000, 0.8660254037844387076, 1.000000000000000000, 0.8660254037844387076, 1.000000000000000000, 0.8660254037844387076, 1.000000000000000000, 0.8660254037844387076, 1.000000000000000000, 0.8660254037844387076, 1.000000000000000000, 0.8660254037844387076, 1.000000000000000000, 0.8660254037844387076, 1.000000000000000000, 0.8660254037844387076, 1.000000000000000000, 0.8660254037844387076, 1.000000000000000000, 0.8660254037844387076, 1.000000000000000000, 0.8660254037844387076, 1.000000000000000000, 0.8660254037844387076, 1.000000000000000000, 0.8660254037844387076, 1.000000000000000000, 0.8660254037844387076, 1.000000000000000000, 0.8660254037844387076, 1.000000000000000000, 0.8660254037844387076, 1.000000000000000000, 0.8660254037844387076, 1.000000000000000000, 0.8660254037844387076, 1.000000000000000000, 0.8660254037844387076, 1.000000000000000000, 0.8660254037844387076, 1.000000000000000000, 0.8660254037844387076, 1.000000000000000000, 0.8660254037844387076, 1.000000000000000000, 0.8660254037844387076, 1.000000000000000000, 0.8660254037844387076, 1.000000000000000000, 0.8660254037844387076, 1.000000000000000000, 0.8660254037844387076, 1.000000000000000000, 0.8660254037844387076, 1.000000000000000000, 0.8660254037844387076, 1.000000000000000000, 0.8660254037844387076, 1.000000000000000000, 0.8660254037844387076, 1.000000000000000000, 0.8660254037844387076, 1.000000000000000000, 0.8660254037844387076, 1.000000000000000000, 0.8660254037844387076, 1.000000000000000000, 0.8660254037844387076, 1.000000000000000000, 0.8660254037844387076, 1.000000000000000000, 0.8660254037844387076, 1.000000000000000000, 0.8660254037844387076, 1.000000000000000000, 0.8660254037844387076, 1.000000000000000000, 0.8660254037844387076, 1.000000000000000000, 0.8660254037844387076, 1.000000000000000000, 0.8660254037844387076, 1.000000000000000000, 0.8660254037844387076, 1.000000000000000000, 0.8660254037844387076, 1.000000000000000000, 0.8660254037844387076, 1.000000000000000000, 0.8660254037844387076, 1.000000000000000000, 0.8660254037844387076, 1.000000000000000000, 0.8660254037844387076, 1.000000000000000000, 0.8660254037844387076, 1.000000000000000000, 0.8660254037844387076, 1.000000000000000000, 0.8660254037844387076, 1.000000000000000000, 0.8660254037844387076, 1.000000000000000000, 0.8660254037844387076, 1.000000000000000000, 0.8660254037844387076, 1.000000000000000000, 0.8660254037844387076, 1.000000000000000000, 0.8660254037844387076, 1.000000000000000000, 0.8660254037844387076, 1.000000000000000000, 0.8660254037844387076, 1.000000000000000000, 0.8660254037844387076, 1.000000000000000000, 0.8660254037844387076, 1.000000000000000000, 0.8660254037844387076, 1.000000000000000000, 0.8660254037844387076, 1.000000000000000000, 0.8660254037844387076, 1.000000000000000000, 0.8660254037844387076, 1.000000000000000000, 0.8660254037844387076, 1.000000000000000000, 0.8660254037844387076, 1.000000000000000000, 0.8660254037844387076, 1.000000000000000000, 0.8660254037844387076, 1.000000000000000000, 0.8660254037844387076, 1.000000000000000000, 0.8660254037844387076, 1.000000000000000000, 0.8660254037844387076, 1.000000000000000000, 0.8660254037844387076, 1.000000000000000000, 0.8660254037844387076, 1.000000000000000000, 0.8660254037844387076, 1.000000000000000000, 0.8660254037844387076, 1.000000000000000000, 0.8660254037844387076, 1.000000000000000000, 0.8660254037844387076, 1.000000000000000000, 0.8660254037844387076, 1.000000000000000000, 0.8660254037844387076, 1.000000000000000000, 0.8660254037844387076, 1.000000000000000000, 0.8660254037844387076, 1.000000000000000000, 0.8660254037844387076, 1.000000000000000000, 0.8660254037844387076, 1.000000000000000000, 0.8660254037844387076, 1.000000000000000000, 0.8660254037844387076, 1.000000000000000000, 0.8660254037844387076, 1.000000000000000000, 0.8660254037844387076, 1.000000000000000000, 0.8660254037844387076, 1.000000000000000000, 0.8660254037844387076, 1.000000000000000000, 0.8660254037844387076, 1.000000000000000000, 0.8660254037844387076, 1.000000000000000000, 0.8660254037844387076, 1.000000000000000000, 0.8660254037844387076, 1.000000000000000000, 0.8660254037844387076, 1.000000000000000000, 0.8660254037844387076, 1.000000000000000000, 0.8660254037844387076, 1.000000000000000000, 0.8660254037844387076, 1.000000000000000000, 0.8660254037844387076, 1.000000000000000000, 0.8660254037844387076, 1.000000000000000000, 0.8660254037844387076, 1.000000000000000000, 0.8660254037844387076, 1.000000000000000000, 0.8660254037844387076, 1.000000000000000000, 0.8660254037844387076, 1.000000000000000000, 0.8660254037844387076, 1.000000000000000000, 0.8660254037844387076, 1.000000000000000000, 0.8660254037844387076, 1.000000000000000000, 0.8660254037844387076, 1.000000000000000000, 0.8660254037844387076, 1.000000000000000000, 0.8660254037844387076, 1.000000000000000000, 0.8660254037844387076, 1.000000000000000000, 0.8660254037844387076, 1.000000000000000000, 0.8660254037844387076, 1.000000000000000000, 0.8660254037844387076, 1.000000000000000000, 0.8660254037844387076, 1.000000000000000000, 0.8660254037844387076, 1.000000000000000000, 0.8660254037844387076, 1.000000000000000000, 0.8660254037844387076, 1.000000000000000000, 0.8660254037844387076, 1.000000000000000000, 0.8660254037844387076, 1.000000000000000000, 0.8660254037844387076, 1.000000000000000000, 0.8660254037844387076, 1.000000000000000000, 0.8660254037844387076, 1.000000000000000000, 0.8660254037844387076, 1.000000000000000000, 0.8660254037844387076, 1.000000000000000000, 0.8660254037844387076, 1.000000000000000000, 0.8660254037844387076, 1.000000000000000000, 0.8660254037844387076, 1.000000000000000000, 0.8660254037844387076, 1.000000000000000000, 0.8660254037844387076, 1.000000000000000000, 0.8660254037844387076, 1.000000000000000000, 0.8660254037844387076, 1.000000000000000000, 0.8660254037844387076, 1.000000000000000000, 0.8660254037844387076, 1.000000000000000000, 0.8660254037844387076, 1.000000000000000000, 0.8660254037844387076, 1.000000000000000000, 0.8660254037844387076, 1.000000000000000000, 0.8660254037844387076, 1.000000000000000000, 0.8660254037844387076, 1.000000000000000000, 0.8660254037844387076, 1.000000000000000000, 0.8660254037844387076, 1.000000000000000000, 0.8660254037844387076, 1.000000000000000000, 0.8660254037844387076, 1.000000000000000000, 0.8660254037844387076, 1.000000000000000000, 0.8660254037844387076, 1.000000000000000000, 0.8660254037844387076, 1.000000000000000000, 0.8660254037844387076, 1.000000000000000000, 0.8660254037844387076, 1.000000000000000000, 0.8660254037844387076, 1.000000000000000000, 0.8660254037844387076, 1.000000000000000000, 0.8660254037844387076, 1.000000000000000000, 0.8660254037844387076, 1.000000000000000000, 0.8660254037844387076, 1.000000000000000000, 0.8660254037844387076, 1.000000000000000000, 0.8660254037844387076, 1.000000000000000000, 0.8660254037844387076, 1.000000000000000000, 0.8660254037844387076, 1.000000000000000000, 0.8660254037844387076, 1.000000000000000000, 0.8660254037844387076, 1.000000000000000000, 0.8660254037844387076, 1.000000000000000000, 0.8660254037844387076, 1.000000000000000000, 0.8660254037844387076, 1.000000000000000000, 0.8660254037844387076, 1.000000000000000000, 0.8660254037844387076, 1.000000000000000000, 0.8660254037844387076, 1.000000000000000000, 0.8660254037844387076, 1.000000000000000000, 0.8660254037844387076, 1.000000000000000000, 0.8660254037844387076, 1.000000000000000000, 0.8660254037844387076, 1.000000000000000000, 0.8660254037844387076, 1.000000000000000000, 0.8660254037844387076, 1.000000000000000000, 0.8660254037844387076, 1.000000000000000000, 0.8660254037844387076, 1.000000000000000000, 0.8660254037844387076, 1.000000000000000000, 0.9548846649268323272, 0.9401540970596700131),
 ( 1.000000000000000000, 0.8660254037844387076, 1.000000000000000000, 0.8660254037844387076, 1.000000000000000000, 0.8660254037844387076, 1.000000000000000000, 0.8660254037844387076, 1.000000000000000000, 0.8660254037844387076, 1.000000000000000000, 0.8660254037844387076, 1.000000000000000000, 0.8660254037844387076, 1.000000000000000000, 0.8660254037844387076, 1.000000000000000000, 0.8660254037844387076, 1.000000000000000000, 0.8660254037844387076, 1.000000000000000000, 0.8660254037844387076, 1.000000000000000000, 0.8660254037844387076, 1.000000000000000000, 0.8660254037844387076, 1.000000000000000000, 0.8660254037844387076, 1.000000000000000000, 0.8660254037844387076, 1.000000000000000000, 0.8660254037844387076, 1.000000000000000000, 0.8660254037844387076, 1.000000000000000000, 0.8660254037844387076, 1.000000000000000000, 0.8660254037844387076, 1.000000000000000000, 0.8660254037844387076, 1.000000000000000000, 0.8660254037844387076, 1.000000000000000000, 0.8660254037844387076, 1.000000000000000000, 0.8660254037844387076, 1.000000000000000000, 0.8660254037844387076, 1.000000000000000000, 0.8660254037844387076, 1.000000000000000000, 0.8660254037844387076, 1.000000000000000000, 0.8660254037844387076, 1.000000000000000000, 0.8660254037844387076, 1.000000000000000000, 0.8660254037844387076, 1.000000000000000000, 0.8660254037844387076, 1.000000000000000000, 0.8660254037844387076, 1.000000000000000000, 0.8660254037844387076, 1.000000000000000000, 0.8660254037844387076, 1.000000000000000000, 0.8660254037844387076, 1.000000000000000000, 0.8660254037844387076, 1.000000000000000000, 0.8660254037844387076, 1.000000000000000000, 0.8660254037844387076, 1.000000000000000000, 0.8660254037844387076, 1.000000000000000000, 0.8660254037844387076, 1.000000000000000000, 0.8660254037844387076, 1.000000000000000000, 0.8660254037844387076, 1.000000000000000000, 0.8660254037844387076, 1.000000000000000000, 0.8660254037844387076, 1.000000000000000000, 0.8660254037844387076, 1.000000000000000000, 0.8660254037844387076, 1.000000000000000000, 0.8660254037844387076, 1.000000000000000000, 0.8660254037844387076, 1.000000000000000000, 0.8660254037844387076, 1.000000000000000000, 0.8660254037844387076, 1.000000000000000000, 0.8660254037844387076, 1.000000000000000000, 0.8660254037844387076, 1.000000000000000000, 0.8660254037844387076, 1.000000000000000000, 0.8660254037844387076, 1.000000000000000000, 0.8660254037844387076, 1.000000000000000000, 0.8660254037844387076, 1.000000000000000000, 0.8660254037844387076, 1.000000000000000000, 0.8660254037844387076, 1.000000000000000000, 0.8660254037844387076, 1.000000000000000000, 0.8660254037844387076, 1.000000000000000000, 0.8660254037844387076, 1.000000000000000000, 0.8660254037844387076, 1.000000000000000000, 0.8660254037844387076, 1.000000000000000000, 0.8660254037844387076, 1.000000000000000000, 0.8660254037844387076, 1.000000000000000000, 0.8660254037844387076, 1.000000000000000000, 0.8660254037844387076, 1.000000000000000000, 0.8660254037844387076, 1.000000000000000000, 0.8660254037844387076, 1.000000000000000000, 0.8660254037844387076, 1.000000000000000000, 0.8660254037844387076, 1.000000000000000000, 0.8660254037844387076, 1.000000000000000000, 0.8660254037844387076, 1.000000000000000000, 0.8660254037844387076, 1.000000000000000000, 0.8660254037844387076, 1.000000000000000000, 0.8660254037844387076, 1.000000000000000000, 0.8660254037844387076, 1.000000000000000000, 0.8660254037844387076, 1.000000000000000000, 0.8660254037844387076, 1.000000000000000000, 0.8660254037844387076, 1.000000000000000000, 0.8660254037844387076, 1.000000000000000000, 0.8660254037844387076, 1.000000000000000000, 0.8660254037844387076, 1.000000000000000000, 0.8660254037844387076, 1.000000000000000000, 0.8660254037844387076, 1.000000000000000000, 0.8660254037844387076, 1.000000000000000000, 0.8660254037844387076, 1.000000000000000000, 0.8660254037844387076, 1.000000000000000000, 0.8660254037844387076, 1.000000000000000000, 0.8660254037844387076, 1.000000000000000000, 0.8660254037844387076, 1.000000000000000000, 0.8660254037844387076, 1.000000000000000000, 0.8660254037844387076, 1.000000000000000000, 0.8660254037844387076, 1.000000000000000000, 0.8660254037844387076, 1.000000000000000000, 0.8660254037844387076, 1.000000000000000000, 0.8660254037844387076, 1.000000000000000000, 0.8660254037844387076, 1.000000000000000000, 0.8660254037844387076, 1.000000000000000000, 0.8660254037844387076, 1.000000000000000000, 0.8660254037844387076, 1.000000000000000000, 0.8660254037844387076, 1.000000000000000000, 0.8660254037844387076, 1.000000000000000000, 0.8660254037844387076, 1.000000000000000000, 0.8660254037844387076, 1.000000000000000000, 0.8660254037844387076, 1.000000000000000000, 0.8660254037844387076, 1.000000000000000000, 0.8660254037844387076, 1.000000000000000000, 0.8660254037844387076, 1.000000000000000000, 0.8660254037844387076, 1.000000000000000000, 0.8660254037844387076, 1.000000000000000000, 0.8660254037844387076, 1.000000000000000000, 0.8660254037844387076, 1.000000000000000000, 0.8660254037844387076, 1.000000000000000000, 0.8660254037844387076, 1.000000000000000000, 0.8660254037844387076, 1.000000000000000000, 0.8660254037844387076, 1.000000000000000000, 0.8660254037844387076, 1.000000000000000000, 0.8660254037844387076, 1.000000000000000000, 0.8660254037844387076, 1.000000000000000000, 0.8660254037844387076, 1.000000000000000000, 0.8660254037844387076, 1.000000000000000000, 0.8660254037844387076, 1.000000000000000000, 0.8660254037844387076, 1.000000000000000000, 0.8660254037844387076, 1.000000000000000000, 0.8660254037844387076, 1.000000000000000000, 0.8660254037844387076, 1.000000000000000000, 0.8660254037844387076, 1.000000000000000000, 0.8660254037844387076, 1.000000000000000000, 0.8660254037844387076, 1.000000000000000000, 0.8660254037844387076, 1.000000000000000000, 0.8660254037844387076, 1.000000000000000000, 0.8660254037844387076, 1.000000000000000000, 0.8660254037844387076, 1.000000000000000000, 0.8660254037844387076, 1.000000000000000000, 0.8660254037844387076, 1.000000000000000000, 0.8660254037844387076, 1.000000000000000000, 0.8660254037844387076, 1.000000000000000000, 0.8660254037844387076, 1.000000000000000000, 0.8660254037844387076, 1.000000000000000000, 0.8660254037844387076, 1.000000000000000000, 0.8660254037844387076, 1.000000000000000000, 0.8660254037844387076, 1.000000000000000000, 0.8660254037844387076, 1.000000000000000000, 0.8660254037844387076, 1.000000000000000000, 0.8660254037844387076, 1.000000000000000000, 0.8660254037844387076, 1.000000000000000000, 0.8660254037844387076, 1.000000000000000000, 0.8660254037844387076, 1.000000000000000000, 0.8660254037844387076, 1.000000000000000000, 0.8660254037844387076, 1.000000000000000000, 0.8660254037844387076, 1.000000000000000000, 0.8660254037844387076, 1.000000000000000000, 0.8660254037844387076, 1.000000000000000000, 0.8660254037844387076, 1.000000000000000000, 0.8660254037844387076, 1.000000000000000000, 0.8660254037844387076, 1.000000000000000000, 0.8660254037844387076, 1.000000000000000000, 0.8660254037844387076, 1.000000000000000000, 0.8660254037844387076, 1.000000000000000000, 0.8660254037844387076, 1.000000000000000000, 0.8660254037844387076, 1.000000000000000000, 0.8660254037844387076, 1.000000000000000000, 0.8660254037844387076, 1.000000000000000000, 0.8660254037844387076, 1.000000000000000000, 0.8660254037844387076, 1.000000000000000000, 0.8660254037844387076, 1.000000000000000000, 0.8660254037844387076, 1.000000000000000000, 0.8660254037844387076, 1.000000000000000000, 0.8660254037844387076, 1.000000000000000000, 0.8660254037844387076, 1.000000000000000000, 0.8660254037844387076, 1.000000000000000000, 0.8660254037844387076, 1.000000000000000000, 0.8660254037844387076, 1.000000000000000000, 0.9548846649268323272, 0.9401540970596700131) ) ) 
 REPRESENTATION_ITEM ( '' )  SURFACE ( )  );
#11829=VERTEX_POINT ( 'NONE', #18054 ) ;
#11830=CARTESIAN_POINT ( 'NONE',  ( -5.330712181944246111E-15, -27.33340804591119522, -6.211691927533303570 ) ) ;
#11832=ORIENTED_EDGE ( 'NONE', *, *, #10205, .F. ) ;
#11835=CARTESIAN_POINT ( 'NONE',  ( 2.121784821875004390, -22.78265288675364175, -14.66275540855586890 ) ) ;
#11837=CARTESIAN_POINT ( 'NONE',  ( -4.000000000000004441, -27.72246025710361295, -11.28397838367063244 ) ) ;
#11838=CARTESIAN_POINT ( 'NONE',  ( 4.730628863548789710E-15, -16.33737451245578498, -7.593689001224928958 ) ) ;
#11840=CARTESIAN_POINT ( 'NONE',  ( -4.000000000000004441, -25.39947568988189985, -7.966412604300202815 ) ) ;
#11841=EDGE_CURVE ( 'NONE', #14660, #12399, #2197, .T. ) ;
#11842=CARTESIAN_POINT ( 'NONE',  ( -3.999999999999997335, -20.62655511095648109, -9.202611407326488191 ) ) ;
#11845=EDGE_LOOP ( 'NONE', ( #14021, #15516 ) ) ;
#11847=CARTESIAN_POINT ( 'NONE',  ( 3.579096709490575479E-14, -24.61191250054342916, -3.894186529857098567 ) ) ;
#11848=DIRECTION ( 'NONE',  ( -0.000000000000000000, 1.000000000000000000, 0.000000000000000000 ) ) ;
#11854=CARTESIAN_POINT ( 'NONE',  ( -3.999999999999997335, -20.82013715752001559, -9.479075221267256879 ) ) ;
#11855=ORIENTED_EDGE ( 'NONE', *, *, #10050, .F. ) ;
#11857=DIRECTION ( 'NONE',  ( 0.000000000000000000, -0.5735764363510547081, -0.8191520442889856923 ) ) ;
#11860=LINE ( 'NONE', #17458, #2235 ) ;
#11861=CARTESIAN_POINT ( 'NONE',  ( 4.243569643750000786, -20.89974471738585748, -5.566448692132691001 ) ) ;
#11862=CARTESIAN_POINT ( 'NONE',  ( 4.243569643750000786, -24.54553994094216307, -10.77318387364461572 ) ) ;
#11864=CARTESIAN_POINT ( 'NONE',  ( 1.999999999999994449, -29.37813640364300127, -11.63537001862205855 ) ) ;
#11866=CARTESIAN_POINT ( 'NONE',  ( 3.678256433395794112, -9.999999999998108180, 21.51556408013178157 ) ) ;
#11868=CARTESIAN_POINT ( 'NONE',  ( -5.577813053751546416E-15, -25.45076803941176991, -5.092196395636519490 ) ) ;
#11870=ORIENTED_EDGE ( 'NONE', *, *, #3497, .F. ) ;
#11873=CARTESIAN_POINT ( 'NONE',  ( 4.005420803925811235, -27.01550616763517709, -14.30066121701663029 ) ) ;
#11874=CARTESIAN_POINT ( 'NONE',  ( -2.121784821874996396, -18.83573003411303048, -9.025965403792225672 ) ) ;
#11878=CARTESIAN_POINT ( 'NONE',  ( -1.999999999999996225, -23.25119311998180649, -14.96414190187491400 ) ) ;
#11879=CARTESIAN_POINT ( 'NONE',  ( 4.243569643749996345, -22.96046137712846047, -4.237966970562988323 ) ) ;
#11880=CARTESIAN_POINT ( 'NONE',  ( -7.082115535667631079, -12.11711825479596172, 11.44395564418984002 ) ) ;
#11885=CARTESIAN_POINT ( 'NONE',  ( -1.071796769724486564, -27.97886135391585682, -8.702687823603630690 ) ) ;
#11886=ORIENTED_EDGE ( 'NONE', *, *, #2441, .T. ) ;
#11887=ORIENTED_EDGE ( 'NONE', *, *, #4909, .F. ) ;
#11889=FACE_OUTER_BOUND ( 'NONE', #8766, .T. ) ;
#11894=CARTESIAN_POINT ( 'NONE',  ( 4.243569643750003451, -24.03347965934736763, -14.31337611479460037 ) ) ;
#11897=PLANE ( 'NONE',  #9287 ) ;
#11898=CARTESIAN_POINT ( 'NONE',  ( 2.237551826325104631, -10.00000000000000178, -12.18738508574795176 ) ) ;
#11899=AXIS2_PLACEMENT_3D ( 'NONE', #1044, #18024, #3907 ) ;
#11900=CARTESIAN_POINT ( 'NONE',  ( -2.121784821875005722, -28.15821100236278696, -9.525377681565375454 ) ) ;
#11902=CARTESIAN_POINT ( 'NONE',  ( -2.000000000000005773, -27.03364271935316765, -8.287086036584028648 ) ) ;
#11904=CARTESIAN_POINT ( 'NONE',  ( 4.243569643750003451, -22.48482328119956009, -12.10166559521431573 ) ) ;
#11905=( BOUNDED_CURVE ( )  B_SPLINE_CURVE ( 3, ( #3905, #8160, #12519, #8696 ),
 .UNSPECIFIED., .F., .F. ) 
 B_SPLINE_CURVE_WITH_KNOTS ( ( 4, 4 ),
 ( 8.673617379884036458E-16, 1.570796326794896558 ),
 .UNSPECIFIED. ) 
 CURVE ( )  GEOMETRIC_REPRESENTATION_ITEM ( )  RATIONAL_B_SPLINE_CURVE ( ( 1.000000000000000000, 0.8047378541243652705, 0.8047378541243652705, 1.000000000000000000 ) ) 
 REPRESENTATION_ITEM ( '' )  );
#11910=CARTESIAN_POINT ( 'NONE',  ( -2.121784821875005722, -26.06107215695429247, -6.530353019633736267 ) ) ;
#11911=CARTESIAN_POINT ( 'NONE',  ( -6.158835246850665095E-15, -22.64013793229036509, -15.02577497543054186 ) ) ;
#11914=EDGE_LOOP ( 'NONE', ( #17086, #11886, #6336, #227 ) ) ;
#11919=CARTESIAN_POINT ( 'NONE',  ( 3.999999999999996447, -22.21612646813362346, -3.420118758496274225 ) ) ;
#11922=ORIENTED_EDGE ( 'NONE', *, *, #14431, .F. ) ;
#11923=CARTESIAN_POINT ( 'NONE',  ( 4.243569643750003451, -20.45221178488055713, -9.198795538265191141 ) ) ;
#11930=CARTESIAN_POINT ( 'NONE',  ( -4.243569643750005227, -27.17624818430860856, -10.25873449608710608 ) ) ;
#11931=CARTESIAN_POINT ( 'NONE',  ( -1.071796769724496334, -28.55960749642623142, -9.532079269453008763 ) ) ;
#11935=CARTESIAN_POINT ( 'NONE',  ( 1.999999999999994449, -25.44196810847903478, -6.013939113682064352 ) ) ;
#11936=CARTESIAN_POINT ( 'NONE',  ( 4.730628863548789710E-15, -16.07926511609781528, -7.225070581294880334 ) ) ;
#11939=CARTESIAN_POINT ( 'NONE',  ( 1.999999999999994449, -26.02271425098940938, -6.843330559531437984 ) ) ;
#11940=CARTESIAN_POINT ( 'NONE',  ( 1.999999999999994449, -26.53893304370534523, -7.580567399391532568 ) ) ;
#11942=( BOUNDED_CURVE ( )  B_SPLINE_CURVE ( 2, ( #12554, #18239, #5509, #10124, #7346, #15708, #5605, #11250, #127 ),
 .UNSPECIFIED., .F., .T. ) 
 B_SPLINE_CURVE_WITH_KNOTS ( ( 3, 2, 2, 2, 3 ),
 ( 0.6637931034482759118, 0.6666666666666666297, 0.6724137931034482873, 0.6781609195402298340, 0.6810344827586206629 ),
 .UNSPECIFIED. ) 
 CURVE ( )  GEOMETRIC_REPRESENTATION_ITEM ( )  RATIONAL_B_SPLINE_CURVE ( ( 0.9330127018922194093, 0.9330127018922206306, 1.000000000000000000, 0.8660254037844387076, 1.000000000000000000, 0.8660254037844387076, 1.000000000000000000, 0.9330127018922194093, 0.9330127018922194093 ) ) 
 REPRESENTATION_ITEM ( '' )  );
#11951=ORIENTED_EDGE ( 'NONE', *, *, #3061, .T. ) ;
#11953=CARTESIAN_POINT ( 'NONE',  ( -5.279047395330986450E-15, -25.37691494596528941, -3.907874615766512960 ) ) ;
#11954=ORIENTED_EDGE ( 'NONE', *, *, #4671, .T. ) ;
#11958=CARTESIAN_POINT ( 'NONE',  ( -4.243569643749998122, -18.26903647401939779, -6.080898069690205965 ) ) ;
#11959=CARTESIAN_POINT ( 'NONE',  ( 4.243569643750003451, -22.51708695574430763, -12.14774289770557303 ) ) ;
#11961=CARTESIAN_POINT ( 'NONE',  ( 4.000000000000000888, -26.49749225125177432, -13.56086067486898372 ) ) ;
#11963=CARTESIAN_POINT ( 'NONE',  ( 8.535862155146745067, -10.00000000000000178, 16.49127580077287902 ) ) ;
#11966=CARTESIAN_POINT ( 'NONE',  ( -5.330712181944245322E-15, -30.94693959492275681, -11.37234980655397010 ) ) ;
#11967=ORIENTED_EDGE ( 'NONE', *, *, #15610, .T. ) ;
#11970=CARTESIAN_POINT ( 'NONE',  ( -4.243569643750000786, -22.06123700099670870, -7.225231581817909365 ) ) ;
#11973=CARTESIAN_POINT ( 'NONE',  ( 4.730628863548789710E-15, -22.27389062868905967, -16.07191265961602511 ) ) ;
#11974=CARTESIAN_POINT ( 'NONE',  ( 4.000000000000003553, -24.26159577562626524, -14.39398748700122077 ) ) ;
#11975=CARTESIAN_POINT ( 'NONE',  ( -4.243569643750000786, -21.06106309010958100, -5.796835204588974833 ) ) ;
#11979=ORIENTED_EDGE ( 'NONE', *, *, #11440, .T. ) ;
#11981=EDGE_CURVE ( 'NONE', #17584, #16586, #15016, .T. ) ;
#11984=VERTEX_POINT ( 'NONE', #1523 ) ;
#11986=CARTESIAN_POINT ( 'NONE',  ( 2.121784821875004390, -21.97606102313498511, -13.51082284627447017 ) ) ;
#11989=CARTESIAN_POINT ( 'NONE',  ( 0.000000000000000000, 0.000000000000000000, 30.00000000000000000 ) ) ;
#11991=CARTESIAN_POINT ( 'NONE',  ( 3.122678035296257093, -15.23680830283740129, -9.380745725235836829 ) ) ;
#11992=CARTESIAN_POINT ( 'NONE',  ( -4.243569643749997233, -23.72159747208149128, -13.86796219071246306 ) ) ;
#11996=CARTESIAN_POINT ( 'NONE',  ( -2.121784821874996396, -20.12627701590287543, -10.86905750344246435 ) ) ;
#12000=CARTESIAN_POINT ( 'NONE',  ( 0.000000000000000000, 9.254131787996968228, 30.52396275209373044 ) ) ;
#12002=FACE_OUTER_BOUND ( 'NONE', #3971, .T. ) ;
#12004=CARTESIAN_POINT ( 'NONE',  ( -3.999999999999997335, -24.75630545268398208, -15.10050612620724841 ) ) ;
#12008=CARTESIAN_POINT ( 'NONE',  ( -4.243569643750004339, -24.33704482437095251, -6.203931876856584537 ) ) ;
#12010=( BOUNDED_SURFACE ( )  B_SPLINE_SURFACE ( 3, 2, ( 
 ( #3106, #8644, #1620 ),
 ( #8736, #1716, #7352 ),
 ( #13012, #324, #14514 ),
 ( #5962, #11616, #1812 ),
 ( #7448, #13105, #6057 ),
 ( #11709, #2003, #16097 ),
 ( #10416, #3292, #511 ),
 ( #7541, #2097, #1913 ),
 ( #787, #13196, #6348 ),
 ( #17499, #16179, #4764 ),
 ( #6523, #7724, #11991 ),
 ( #14800, #8931, #3654 ),
 ( #9302, #880, #3476 ),
 ( #11898, #6247, #14894 ),
 ( #17780, #13385, #17685 ),
 ( #14979, #700, #17596 ),
 ( #12173, #4862, #12078 ),
 ( #14707, #17863, #4947 ) ),
 .UNSPECIFIED., .F., .F., .T. ) 
 B_SPLINE_SURFACE_WITH_KNOTS ( ( 4, 2, 2, 2, 2, 2, 2, 2, 4 ),
 ( 3, 3 ),
 ( 5.253488506341834174, 5.382200606446552626, 5.510912706551271967, 5.639624806655991307, 5.768336906760710647, 5.897049006865429988, 6.025761106970148440, 6.154473207074866892, 6.283185307179586232 ),
 ( 0.000000000000000000, 1.000000000000000000 ),
 .UNSPECIFIED. ) 
 GEOMETRIC_REPRESENTATION_ITEM ( )  RATIONAL_B_SPLINE_SURFACE ( (
 ( 1.000000000000000000, 0.5376207706124462860, 1.000000000000000000),
 ( 1.000000000000000000, 0.5236136374383226766, 1.000000000000000000),
 ( 1.000000000000000000, 0.5095962305068678644, 1.000000000000000000),
 ( 1.000000000000000000, 0.4818058245216391144, 1.000000000000000000),
 ( 1.000000000000000000, 0.4680310812906506301, 1.000000000000000000),
 ( 1.000000000000000000, 0.4410557726863417738, 1.000000000000000000),
 ( 1.000000000000000000, 0.4278543698619108882, 1.000000000000000000),
 ( 1.000000000000000000, 0.4024558808744606586, 1.000000000000000000),
 ( 1.000000000000000000, 0.3902583003213770385, 1.000000000000000000),
 ( 1.000000000000000000, 0.3674181228096251028, 1.000000000000000000),
 ( 1.000000000000000000, 0.3567764320979142645, 1.000000000000000000),
 ( 1.000000000000000000, 0.3377179606062171713, 1.000000000000000000),
 ( 1.000000000000000000, 0.3293051245441800390, 1.000000000000000000),
 ( 1.000000000000000000, 0.3154271731554472158, 1.000000000000000000),
 ( 1.000000000000000000, 0.3099694920613502158, 1.000000000000000000),
 ( 1.000000000000000000, 0.3026053347213686351, 1.000000000000000000),
 ( 1.000000000000000000, 0.3006987634938562692, 1.000000000000000000),
 ( 1.000000000000000000, 0.3007057995042700660, 1.000000000000000000) ) ) 
 REPRESENTATION_ITEM ( '' )  SURFACE ( )  );
#12011=ORIENTED_EDGE ( 'NONE', *, *, #8243, .F. ) ;
#12013=CARTESIAN_POINT ( 'NONE',  ( 1.071796769724485232, -24.85849519618256664, -4.246343115131230306 ) ) ;
#12014=AXIS2_PLACEMENT_3D ( 'NONE', #17403, #15711, #12913 ) ;
#12016=EDGE_CURVE ( 'NONE', #10059, #14859, #8810, .T. ) ;
#12021=CARTESIAN_POINT ( 'NONE',  ( 4.243569643750000786, -20.67389899557263533, -5.243907574693898788 ) ) ;
#12022=ORIENTED_EDGE ( 'NONE', *, *, #8300, .F. ) ;
#12023=FACE_OUTER_BOUND ( 'NONE', #7860, .T. ) ;
#12024=CARTESIAN_POINT ( 'NONE',  ( -4.000000000000004441, -25.65758508623986600, -8.335031024230250551 ) ) ;
#12032=VECTOR ( 'NONE', #9307, 1000.000000000000000 ) ;
#12034=EDGE_LOOP ( 'NONE', ( #18128, #15834, #6048 ) ) ;
#12036=CARTESIAN_POINT ( 'NONE',  ( 4.713407268011036227E-15, -18.19707658806250805, -9.759274404511186773 ) ) ;
#12038=CARTESIAN_POINT ( 'NONE',  ( -5.577813053751546416E-15, -29.25788163498686245, -10.52931808859795559 ) ) ;
#12041=DIRECTION ( 'NONE',  ( 0.000000000000000000, 0.000000000000000000, 1.000000000000000000 ) ) ;
#12043=CARTESIAN_POINT ( 'NONE',  ( 2.121784821874994176, -23.69506935700625050, -3.151350836941627875 ) ) ;
#12044=EDGE_CURVE ( 'NONE', #11008, #4334, #2328, .T. ) ;
#12046=CARTESIAN_POINT ( 'NONE',  ( -5.330712181944245322E-15, -27.84962683862713106, -6.948928767393398154 ) ) ;
#12048=VERTEX_POINT ( 'NONE', #9765 ) ;
#12049=CARTESIAN_POINT ( 'NONE',  ( -4.000000000000000888, -19.85117529432912775, -4.068936360663492735 ) ) ;
#12051=CARTESIAN_POINT ( 'NONE',  ( -2.121784821875005722, -29.70686738051060161, -11.73708820114566009 ) ) ;
#12055=CARTESIAN_POINT ( 'NONE',  ( -2.121784821874996396, -18.31951124139709464, -8.288728563932130200 ) ) ;
#12059=CARTESIAN_POINT ( 'NONE',  ( -5.279047395330986450E-15, -29.50666528769278685, -9.805769334647276736 ) ) ;
#12060=CARTESIAN_POINT ( 'NONE',  ( -4.243569643750000786, -20.80295369375161130, -5.428216784658927985 ) ) ;
#12062=DIRECTION ( 'NONE',  ( -0.000000000000000000, -0.5735764363510414965, -0.8191520442889950182 ) ) ;
#12063=CARTESIAN_POINT ( 'NONE',  ( 3.082316921986471225, -29.06618978543598786, -12.78463801463987437 ) ) ;
#12065=DIRECTION ( 'NONE',  ( -0.000000000000000000, -0.5735764363510414965, -0.8191520442889950182 ) ) ;
#12068=DIRECTION ( 'NONE',  ( -0.000000000000000000, -0.5735764363510414965, -0.8191520442889950182 ) ) ;
#12071=CARTESIAN_POINT ( 'NONE',  ( -3.604268994871580478, -29.04518628171981476, -12.79934482627075276 ) ) ;
#12072=ORIENTED_EDGE ( 'NONE', *, *, #2587, .T. ) ;
#12074=SURFACE_STYLE_FILL_AREA ( #7814 ) ;
#12075=CARTESIAN_POINT ( 'NONE',  ( -4.243569643750005227, -27.91831269883777011, -11.31851245338599377 ) ) ;
#12077=CARTESIAN_POINT ( 'NONE',  ( 0.000000000000000000, 9.254131787996968228, 30.52396275209373044 ) ) ;
#12078=CARTESIAN_POINT ( 'NONE',  ( 0.3217809247882234547, -15.45745613286858244, -10.86990606519723279 ) ) ;
#12081=CARTESIAN_POINT ( 'NONE',  ( -4.243569643750005227, -27.17624818430860856, -10.25873449608710608 ) ) ;
#12088=CARTESIAN_POINT ( 'NONE',  ( -4.243569643750005227, -25.59532813161604636, -8.000946674015564142 ) ) ;
#12090=CARTESIAN_POINT ( 'NONE',  ( 4.898587196589413815E-16, 2.700915433685006750, 35.11257424290206330 ) ) ;
#12099=DIRECTION ( 'NONE',  ( -0.9454169814551715012, 0.000000000000000000, 0.3258630558627224061 ) ) ;
#12100=ORIENTED_EDGE ( 'NONE', *, *, #16828, .F. ) ;
#12101=CARTESIAN_POINT ( 'NONE',  ( 2.121784821874994176, -25.79220820241474854, -6.146375498873266174 ) ) ;
#12103=VERTEX_POINT ( 'NONE', #5773 ) ;
#12106=CIRCLE ( 'NONE', #18070, 0.3999999999999991895 ) ;
#12109=CARTESIAN_POINT ( 'NONE',  ( 7.471583913895156748, -13.11946146044265227, 4.276027703312072603 ) ) ;
#12110=ADVANCED_FACE ( 'NONE', ( #17021 ), #4292, .F. ) ;
#12111=CARTESIAN_POINT ( 'NONE',  ( 3.999999999999996447, -26.53945885642465186, -9.594477291317806689 ) ) ;
#12112=CARTESIAN_POINT ( 'NONE',  ( 4.243569643749996345, -22.18613318805455847, -3.132111710772846891 ) ) ;
#12115=CARTESIAN_POINT ( 'NONE',  ( 4.000000000000003553, -21.22881036912508179, -10.06272105382992521 ) ) ;
#12119=ORIENTED_EDGE ( 'NONE', *, *, #18203, .F. ) ;
#12127=CARTESIAN_POINT ( 'NONE',  ( -4.000000000000004441, -22.75385437650777476, -4.188073799010446407 ) ) ;
#12128=ORIENTED_EDGE ( 'NONE', *, *, #2527, .F. ) ;
#12131=CARTESIAN_POINT ( 'NONE',  ( -8.500000000000005329, 10.00000000000000000, 18.49999999999999645 ) ) ;
#12133=CARTESIAN_POINT ( 'NONE',  ( -4.243569643750004339, -22.49801537532042417, -3.577525634854993086 ) ) ;
#12134=CARTESIAN_POINT ( 'NONE',  ( 4.730628863548789710E-15, -19.69279666510938043, -12.38572846031554953 ) ) ;
#12135=CARTESIAN_POINT ( 'NONE',  ( -0.4744323633459381351, -30.28477276999926460, -12.01443746324198258 ) ) ;
#12137=CARTESIAN_POINT ( 'NONE',  ( 3.544496300715735071, -10.00000000000000178, 23.01862375599375099 ) ) ;
#12139=CARTESIAN_POINT ( 'NONE',  ( 4.299564228933482956E-15, -19.47829782620029704, -10.51019933028069708 ) ) ;
#12140=CARTESIAN_POINT ( 'NONE',  ( 4.730628863548789710E-15, -22.53200002504703647, -16.44053107954607640 ) ) ;
#12141=VERTEX_POINT ( 'NONE', #13944 ) ;
#12144=CARTESIAN_POINT ( 'NONE',  ( -5.330712181944245322E-15, -24.20383161507082193, -1.742193585881474771 ) ) ;
#12147=AXIS2_PLACEMENT_3D ( 'NONE', #6137, #17484, #17846 ) ;
#12150=CARTESIAN_POINT ( 'NONE',  ( -2.000000000000005773, -28.32418970114301260, -10.13017813623426733 ) ) ;
#12152=EDGE_CURVE ( 'NONE', #1548, #7899, #2346, .T. ) ;
#12153=CARTESIAN_POINT ( 'NONE',  ( 2.121784821874994176, -24.50166122062490359, -4.303283399223027494 ) ) ;
#12157=AXIS2_PLACEMENT_3D ( 'NONE', #17716, #4983, #3771 ) ;
#12159=CARTESIAN_POINT ( 'NONE',  ( 4.000000000000003553, -20.71259157640914594, -9.325484213969829739 ) ) ;
#12164=CARTESIAN_POINT ( 'NONE',  ( 4.000000000000000888, -26.75560164760974047, -13.92947909479903146 ) ) ;
#12168=( LENGTH_UNIT ( ) NAMED_UNIT ( * ) SI_UNIT ( .MILLI., .METRE. ) );
#12169=CARTESIAN_POINT ( 'NONE',  ( 4.243569643750003451, -22.48482328119956009, -12.10166559521431573 ) ) ;
#12172=DIRECTION ( 'NONE',  ( -0.000000000000000000, -0.5735764363510414965, -0.8191520442889950182 ) ) ;
#12173=CARTESIAN_POINT ( 'NONE',  ( 0.4504932947034594459, -10.00000000000000178, -12.59063537424963997 ) ) ;
#12175=( GEOMETRIC_REPRESENTATION_CONTEXT ( 3 ) GLOBAL_UNCERTAINTY_ASSIGNED_CONTEXT ( ( #9551 ) ) GLOBAL_UNIT_ASSIGNED_CONTEXT ( ( #12168, #2186, #505 ) ) REPRESENTATION_CONTEXT ( 'NONE', 'WORKASPACE' ) );
#12176=CARTESIAN_POINT ( 'NONE',  ( 4.243569643750000786, -25.57797752637403832, -12.24765755336480666 ) ) ;
#12180=DIRECTION ( 'NONE',  ( -0.000000000000000000, -0.5735764363510414965, -0.8191520442889950182 ) ) ;
#12181=CARTESIAN_POINT ( 'NONE',  ( -4.243569643749997233, -20.59202104124112154, -9.398463849060638253 ) ) ;
#12188=CARTESIAN_POINT ( 'NONE',  ( 3.250762944584260072, -21.87258937905581746, -2.200190645090608577 ) ) ;
#12194=CARTESIAN_POINT ( 'NONE',  ( 4.243569643749997233, -24.76722715163424127, -6.818295910073324251 ) ) ;
#12201=CARTESIAN_POINT ( 'NONE',  ( 9.996570547186806266, -9.916659267309226422, 4.908050019500779015 ) ) ;
#12202=CARTESIAN_POINT ( 'NONE',  ( -3.706921591972381904E-14, -17.67153205169451624, -7.929870390770359379 ) ) ;
#12203=CARTESIAN_POINT ( 'NONE',  ( -2.121784821874996396, -16.80311853779403108, -6.123095346843099307 ) ) ;
#12205=CARTESIAN_POINT ( 'NONE',  ( -4.648177544792955347E-16, -30.03220982406077155, -11.63517334838810058 ) ) ;
#12207=CARTESIAN_POINT ( 'NONE',  ( -3.999999999999997335, -21.91710209274632604, -11.04570350697672332 ) ) ;
#12208=CIRCLE ( 'NONE', #6592, 4.000000000000000000 ) ;
#12210=EDGE_LOOP ( 'NONE', ( #12684, #292, #11095, #12389 ) ) ;
#12212=CARTESIAN_POINT ( 'NONE',  ( 1.071796769724487675, -29.56899168042044224, -10.97362927986136860 ) ) ;
#12219=CARTESIAN_POINT ( 'NONE',  ( 1.999999999999994449, -23.11898354125731458, -2.696373334311634284 ) ) ;
#12220=ORIENTED_EDGE ( 'NONE', *, *, #4671, .F. ) ;
#12226=CARTESIAN_POINT ( 'NONE',  ( 4.730628863548789710E-15, -16.04700144155307129, -7.178993278803623035 ) ) ;
#12227=CARTESIAN_POINT ( 'NONE',  ( -4.243569643749997233, -21.65672230121773723, -10.91901483127208294 ) ) ;
#12228=FACE_OUTER_BOUND ( 'NONE', #9832, .T. ) ;
#12233=CARTESIAN_POINT ( 'NONE',  ( 3.579096709490575479E-14, -25.90245948233327056, -5.737278629507336802 ) ) ;
#12234=CARTESIAN_POINT ( 'NONE',  ( 4.730628863548789710E-15, -23.04821881776296877, -17.17776791940616832 ) ) ;
#12237=CARTESIAN_POINT ( 'NONE',  ( -4.243569643749997233, -18.52714587037736393, -6.449516489620252813 ) ) ;
#12240=CARTESIAN_POINT ( 'NONE',  ( -5.279047395330986450E-15, -29.24855589133481715, -9.437150914717227224 ) ) ;
#12242=CARTESIAN_POINT ( 'NONE',  ( 2.121784821874994176, -22.95300484247709250, -2.091572879642740634 ) ) ;
#12246=CARTESIAN_POINT ( 'NONE',  ( -2.121784821875005722, -27.09350974238616416, -8.004826699353927211 ) ) ;
#12248=ADVANCED_FACE ( 'NONE', ( #408 ), #10117, .F. ) ;
#12252=ORIENTED_EDGE ( 'NONE', *, *, #18191, .T. ) ;
#12255=CARTESIAN_POINT ( 'NONE',  ( 4.299564228933482956E-15, -18.70396963712639504, -9.404344070490550322 ) ) ;
#12256=CARTESIAN_POINT ( 'NONE',  ( 1.999999999999994449, -28.79739026113263023, -10.80597857277268403 ) ) ;
#12257=ORIENTED_EDGE ( 'NONE', *, *, #11135, .T. ) ;
#12259=CARTESIAN_POINT ( 'NONE',  ( -2.121784821874996396, -21.67493339405068653, -13.08076802302275077 ) ) ;
#12264=CARTESIAN_POINT ( 'NONE',  ( 0.000000000000000000, 5.977523610840987267, 32.81826849749789687 ) ) ;
#12265=CARTESIAN_POINT ( 'NONE',  ( -4.000000000000002665, 2.343145750507628300, -2.343145750507621194 ) ) ;
#12266=CARTESIAN_POINT ( 'NONE',  ( -2.121784821875005722, -27.64199220964684756, -8.788140841705278206 ) ) ;
#12267=DIRECTION ( 'NONE',  ( -0.000000000000000000, -0.5735764363510414965, -0.8191520442889950182 ) ) ;
#12272=CARTESIAN_POINT ( 'NONE',  ( -5.330712181944245322E-15, -26.52681618229254212, -5.059759365251903951 ) ) ;
#12274=DIRECTION ( 'NONE',  ( 0.000000000000000000, -1.000000000000000000, 0.000000000000000000 ) ) ;
#12275=LINE ( 'NONE', #10359, #6451 ) ;
#12279=CARTESIAN_POINT ( 'NONE',  ( -1.071796769724496334, -23.33289221947241998, -2.067556264862776771 ) ) ;
#12282=( BOUNDED_SURFACE ( )  B_SPLINE_SURFACE ( 3, 2, ( 
 ( #15259, #5596, #2555 ),
 ( #8186, #1253, #4202 ),
 ( #13851, #11063, #1158 ),
 ( #9667, #13942, #6887 ),
 ( #1340, #9851, #15526 ),
 ( #7242, #8629, #1702 ),
 ( #12997, #4377, #119 ),
 ( #211, #14308, #7151 ),
 ( #4751, #14593, #16078 ),
 ( #5950, #495, #1609 ),
 ( #14396, #6135, #5771 ),
 ( #17299, #10403, #11602 ),
 ( #17385, #4564, #10204 ),
 ( #3280, #11412, #6044 ),
 ( #15886, #4472, #11506 ),
 ( #1521, #3181, #15698 ),
 ( #3089, #308, #8915 ),
 ( #11788, #7338, #12817 ) ),
 .UNSPECIFIED., .F., .F., .T. ) 
 B_SPLINE_SURFACE_WITH_KNOTS ( ( 4, 2, 2, 2, 2, 2, 2, 2, 4 ),
 ( 3, 3 ),
 ( 0.000000000000000000, 0.1287121001047187574, 0.2574242002094375148, 0.3861363003141562444, 0.5148484004188750296, 0.6435605005235938147, 0.7722726006283124889, 0.9009847007330312740, 1.029696800837750059 ),
 ( 0.000000000000000000, 1.000000000000000000 ),
 .UNSPECIFIED. ) 
 GEOMETRIC_REPRESENTATION_ITEM ( )  RATIONAL_B_SPLINE_SURFACE ( (
 ( 1.000000000000000000, 0.3007057995042700660, 1.000000000000000000),
 ( 1.000000000000000000, 0.3006987634935809339, 1.000000000000000000),
 ( 1.000000000000000000, 0.3026053347217343426, 1.000000000000000000),
 ( 1.000000000000000000, 0.3099694920609858961, 1.000000000000000000),
 ( 1.000000000000000000, 0.3154271731552417135, 1.000000000000000000),
 ( 1.000000000000000000, 0.3293051245443847641, 1.000000000000000000),
 ( 1.000000000000000000, 0.3377179606062847839, 1.000000000000000000),
 ( 1.000000000000000000, 0.3567764320978462078, 1.000000000000000000),
 ( 1.000000000000000000, 0.3674181228096374263, 1.000000000000000000),
 ( 1.000000000000000000, 0.3902583003213647150, 1.000000000000000000),
 ( 1.000000000000000000, 0.4024558808744609362, 1.000000000000000000),
 ( 1.000000000000000000, 0.4278543698619110547, 1.000000000000000000),
 ( 1.000000000000000000, 0.4410557726863888472, 1.000000000000000000),
 ( 1.000000000000000000, 0.4680310812906007811, 1.000000000000000000),
 ( 1.000000000000000000, 0.4818058245216468860, 1.000000000000000000),
 ( 1.000000000000000000, 0.5095962305068602038, 1.000000000000000000),
 ( 1.000000000000000000, 0.5236136374383265624, 1.000000000000000000),
 ( 1.000000000000000000, 0.5376207706124457308, 1.000000000000000000) ) ) 
 REPRESENTATION_ITEM ( '' )  SURFACE ( )  );
#12283=ORIENTED_EDGE ( 'NONE', *, *, #14075, .F. ) ;
#12284=CARTESIAN_POINT ( 'NONE',  ( -4.243569643750000786, -21.57728188282551685, -6.534072044449069416 ) ) ;
#12287=CARTESIAN_POINT ( 'NONE',  ( 1.071796769724476128, -18.45738694148725401, -9.052187485216423468 ) ) ;
#12289=CARTESIAN_POINT ( 'NONE',  ( 4.243569643750000786, -26.83626083361913217, -14.04467235052378804 ) ) ;
#12291=CARTESIAN_POINT ( 'NONE',  ( 4.968999162825121552, -10.12416982780653463, -1.719962025120755023 ) ) ;
#12292=CARTESIAN_POINT ( 'NONE',  ( -4.000000000000000888, -21.72246841862934730, -6.741419906163105047 ) ) ;
#12293=CARTESIAN_POINT ( 'NONE',  ( -5.330712181944245322E-15, -29.88223833494613402, -9.851798824342527183 ) ) ;
#12294=ORIENTED_EDGE ( 'NONE', *, *, #1019, .T. ) ;
#12296=CARTESIAN_POINT ( 'NONE',  ( 1.999999999999994449, -24.21594847648362858, -4.263001620021102944 ) ) ;
#12302=CARTESIAN_POINT ( 'NONE',  ( 1.999999999999994449, -26.47440569391090648, -7.488412793402255296 ) ) ;
#12306=CARTESIAN_POINT ( 'NONE',  ( 2.121784821874994176, -28.88952095871037429, -10.56979653803383989 ) ) ;
#12308=AXIS2_PLACEMENT_3D ( 'NONE', #4666, #7253, #1445 ) ;
#12309=CARTESIAN_POINT ( 'NONE',  ( -3.999999999999997335, -18.49715259029829539, -6.161509441896827255 ) ) ;
#12313=CARTESIAN_POINT ( 'NONE',  ( 9.000000000000005329, -10.00000000000000000, 15.14468620625654616 ) ) ;
#12314=EDGE_CURVE ( 'NONE', #6787, #13443, #16315, .T. ) ;
#12315=CARTESIAN_POINT ( 'NONE',  ( 4.243569643750003451, -18.35507293947206264, -6.203770876333551954 ) ) ;
#12316=CARTESIAN_POINT ( 'NONE',  ( 2.121784821875004390, -20.20155892317395541, -10.97657120925539154 ) ) ;
#12321=CARTESIAN_POINT ( 'NONE',  ( 4.000000000000000888, -24.69072647674599352, -10.98053173535865135 ) ) ;
#12329=CARTESIAN_POINT ( 'NONE',  ( -3.999999999999997335, -25.01441484904194823, -15.46912454613729793 ) ) ;
#12332=CARTESIAN_POINT ( 'NONE',  ( 4.000000000000000888, -24.62619912695155477, -10.88837712936937230 ) ) ;
#12333=ORIENTED_EDGE ( 'NONE', *, *, #4444, .F. ) ;
#12335=AXIS2_PLACEMENT_3D ( 'NONE', #5415, #18232, #15605 ) ;
#12337=CARTESIAN_POINT ( 'NONE',  ( -2.121784821874996396, -20.90060520497677743, -11.97491276323260756 ) ) ;
#12339=CARTESIAN_POINT ( 'NONE',  ( 1.071796769724476128, -18.00569549856575335, -8.407105251345607044 ) ) ;
#12341=VERTEX_POINT ( 'NONE', #4754 ) ;
#12345=CYLINDRICAL_SURFACE ( 'NONE', #13678, 4.000000000000000000 ) ;
#12346=CARTESIAN_POINT ( 'NONE',  ( 1.071796769724494780, -27.43958915976224944, -7.932527314431709442 ) ) ;
#12350=CARTESIAN_POINT ( 'NONE',  ( 2.121784821874994176, -27.82481969873374794, -9.049245555822391651 ) ) ;
#12354=CARTESIAN_POINT ( 'NONE',  ( -2.121784821874996396, -21.44908767223746437, -12.75822690558396033 ) ) ;
#12362=CARTESIAN_POINT ( 'NONE',  ( 2.121784821875004390, -19.65307645591326846, -10.19325706690404054 ) ) ;
#12363=CARTESIAN_POINT ( 'NONE',  ( 1.999999999999994449, -27.57137062913722048, -9.055041079111724400 ) ) ;
#12364=CARTESIAN_POINT ( 'NONE',  ( 4.000000000000000888, -25.20694526946192937, -11.71776857521874504 ) ) ;
#12366=CARTESIAN_POINT ( 'NONE',  ( 3.999999999999996447, -22.40970851469716152, -3.696582572437044245 ) ) ;
#12370=VECTOR ( 'NONE', #10868, 1000.000000000000000 ) ;
#12375=CARTESIAN_POINT ( 'NONE',  ( -2.121784821875005722, -24.54467945335122536, -4.364719802544705374 ) ) ;
#12381=CARTESIAN_POINT ( 'NONE',  ( -4.243569643750004339, -28.95075028426963826, -12.79298613310618471 ) ) ;
#12382=AXIS2_PLACEMENT_3D ( 'NONE', #6894, #14039, #9402 ) ;
#12385=CARTESIAN_POINT ( 'NONE',  ( 2.000000000000004441, -23.55232074906610507, -15.39419672512663340 ) ) ;
#12387=CARTESIAN_POINT ( 'NONE',  ( -4.000000000000004441, -23.59270991537611550, -5.386083664789866887 ) ) ;
#12388=CARTESIAN_POINT ( 'NONE',  ( 4.730628863548789710E-15, -21.46729876507041013, -14.91998009733462816 ) ) ;
#12389=ORIENTED_EDGE ( 'NONE', *, *, #13450, .F. ) ;
#12391=CARTESIAN_POINT ( 'NONE',  ( -4.000000000000004441, -23.07649112266017610, -4.648846824929771415 ) ) ;
#12394=( BOUNDED_SURFACE ( )  B_SPLINE_SURFACE ( 1, 2, ( 
 ( #9089, #9275, #670, #12234, #10665, #14769, #5009, #14864, #10571, #11966, #6583, #3711, #16335, #7876, #14956, #7697, #13358, #6495, #10844, #6316, #12051, #9361, #17658, #4920, #16245, #2160, #13533, #12140, #10756, #17833, #7791, #5097, #17920, #16432, #13447, #761, #16520, #2341, #6406, #7974, #5192, #3798, #4885, #13225, #446, #11648, #12946, #16124, #7569, #10536, #16210, #3230, #1842, #540, #8867, #5993, #14446, #6186, #14543, #6087, #11737, #1752, #11835, #3131, #17244, #13325, #8964, #9057, #4517, #3502, #7476, #13136, #10161, #257, #7286, #13040, #14642, #11551, #4602, #17532, #4796, #5903, #15931, #17432, #17342, #3414, #14350, #4699, #10350, #8768, #10446, #11930, #14734, #7380, #1650, #16030, #10253, #17625, #15837, #2033, #3320, #1943, #7656, #637, #355, #6277, #10695, #16424, #17740, #845, #14950, #2333, #5091, #7784, #5002, #2152, #6214, #16514, #10659, #933, #11862, #11959, #2244, #13714, #17914, #17557, #10837, #17652, #10564, #13441, #663, #3705, #16152, #9267, #754, #4828, #9354, #13527, #6309, #9447, #16330, #7869, #7964, #15122, #10750, #3618, #3531, #10474, #13620, #17827, #2423, #8053, #6399, #12046, #15030, #6485, #16239, #4913, #6576, #12134, #3792, #12227, #3442, #5183, #14857, #2060, #9083, #14762, #7692, #13352, #9178, #15397, #11019, #16793, #17575, #8413, #7014, #5372, #1387, #13899, #16883, #11104, #12316, #12410, #5640, #13806, #9537, #16702, #1116, #12588, #8239, #11281, #14073, #16974, #18192, #9626, #15215, #5459, #1301, #10931, #12499, #5277, #2696, #3975, #4063, #4250, #12681, #9894, #15302, #15564, #1210, #4159, #9713, #18007, #18103, #2862, #6753, #2516, #2602, #8327, #6846, #13988, #8497, #1026, #8144, #6932, #18274, #5548, #11196, #6666, #9806, #16614, #15487, #2784, #3888, #13140, #1847, #7202, #8871, #15841, #14454, #4606, #14548, #10354, #11371, #261, #10257, #1476, #14169, #15937, #450, #78, #12859, #1654, #3135, #5908, #10165, #1756, #6091, #7112, #12773, #7291, #5731, #7482, #12952, #16033, #5999, #11556, #8772, #4523, #3234, #13046, #15747, #17248, #10069, #17061, #11740, #7384, #17438, #4333, #1566, #359, #3324, #4704, #9980, #15655, #166, #5817, #3049, #8590, #11653, #2955, #17346, #8677, #14263, #11460, #17152, #4427, #14354, #7759, #12021, #5069, #17890, #7849, #13420, #6282, #7573, #10724, #2223, #5162, #10816, #16214, #14832, #13502, #3509, #11838, #13229, #1947, #7660, #9244, #6190, #17629, #817, #12112, #545, #10539, #733, #11936, #16401, #8972, #6376, #2130, #16130, #6463, #6554, #3686, #14738, #16491, #17714, #4890, #12203, #14646, #9332, #4981, #10634, #16308, #15009, #17536, #17807 ),
 ( #3594, #2305, #4800, #911, #14930, #7939, #642, #13596, #9155, #10451, #13329, #3420, #9061, #2037, #1005, #15466, #5525, #14052, #9511, #12656, #6823, #6644, #11262, #9784, #12470, #3863, #9608, #2672, #15280, #9421, #4137, #1092, #2760, #1363, #16676, #15190, #11084, #3955, #13963, #16769, #18255, #13877, #18167, #2580, #8390, #8212, #18075, #5618, #1187, #6994, #10910, #15097, #18347, #3769, #2399, #5345, #11170, #12293, #6731, #8032, #16584, #5437, #4039, #17983, #9689, #10998, #13689, #5253, #16861, #2493, #8123, #15373, #8307, #13781, #1276, #12388, #6911, #12567, #11533, #11628, #7087, #6066, #5794, #10047, #4586, #14525, #11436, #4311, #5885, #17128, #8751, #17225, #13023, #8655, #7269, #4406, #17322, #15724, #12840, #428, #3023, #1822, #5710, #4229, #7459, #10235, #13119, #144, #336, #12752, #14240, #16951, #11351, #14334, #237, #14144, #1632, #12925, #9872, #15546, #5976, #54, #8847, #4499, #10139, #17040, #15821, #9958, #1457, #15912, #3117, #3210, #15633, #2843, #14425, #1728, #2933, #8473, #8568, #1544, #7362, #7179, #2013, #4957, #14904, #16009, #13306, #10518, #14715, #13481, #11720, #9129, #4868, #522, #10610, #9311, #795, #17512, #13569, #14809, #7640, #14985, #17414, #12088, #3482, #2107, #7735, #6441, #10330, #16286, #11816, #13395, #7825, #6257, #5046, #6354, #707, #7550, #1925, #618, #16190, #17786, #4679, #3666, #11996, #10701, #3396, #16378, #11910, #17605, #10427, #17691, #9038, #3574, #8943, #2286, #7915, #888, #4774, #3301, #9223, #14622, #13205, #6166, #2198, #16105, #12362, #5418, #18055, #12181, #6891, #3844, #15074, #12272, #13663, #6710, #2471, #18235, #1072, #15444, #16750, #5329, #9489, #5504, #12548, #17959, #1258, #8193, #6804, #15352, #11151, #2740, #3747, #10980, #2650, #17870, #6531, #8288, #16842, #10795, #5230, #16658, #13855, #3934, #2560, #12453, #4117, #5138, #16464, #9584, #9397, #9766, #15263, #8374, #4023, #1163, #18149, #11067, #13945, #9671, #8099, #14035, #13761, #2379, #8009, #983, #6627, #10885, #16564, #15165, #8827, #13001, #1343, #5953, #12734, #5687, #2912, #14124, #17204, #11245, #4381, #8545, #6974, #4475, #8634, #1437, #4569, #122, #10026, #15800, #10211, #215, #5774, #17023, #18326, #3094, #12904, #15891, #3188, #14220, #7158, #5864, #1524, #11330, #7065, #11511, #12820, #11608, #14400, #17303, #11415, #9940, #15529, #17107, #1612, #16932, #15703, #5598, #3001, #4293, #14313, #313, #8727, #7341, #15609, #1707, #7245, #10118, #12637, #4207, #35, #9854, #2826, #8453, #500, #10500, #1903, #6144, #14882, #17768, #17392, #13097, #7436, #13186, #14790, #11699, #4757, #7717, #17674 ) ),
 .UNSPECIFIED., .F., .F., .T. ) 
 B_SPLINE_SURFACE_WITH_KNOTS ( ( 2, 2 ),
 ( 3, 2, 2, 2, 2, 2, 2, 2, 2, 2, 2, 2, 2, 2, 2, 2, 2, 2, 2, 2, 2, 2, 2, 2, 2, 2, 2, 2, 2, 2, 2, 2, 2, 2, 2, 2, 2, 2, 2, 2, 2, 2, 2, 2, 2, 2, 2, 2, 2, 2, 2, 2, 2, 2, 2, 2, 2, 2, 2, 2, 2, 2, 2, 2, 2, 2, 2, 2, 2, 2, 2, 2, 2, 2, 2, 2, 2, 2, 2, 2, 2, 2, 2, 2, 2, 2, 2, 2, 2, 2, 2, 2, 2, 2, 2, 2, 2, 2, 2, 2, 2, 2, 2, 2, 2, 2, 2, 2, 2, 2, 2, 2, 2, 2, 2, 2, 2, 2, 2, 2, 2, 2, 2, 2, 2, 2, 2, 2, 2, 2, 2, 2, 2, 2, 2, 2, 2, 2, 2, 2, 2, 2, 2, 2, 2, 2, 2, 2, 2, 2, 2, 2, 2, 2, 2, 2, 2, 2, 2, 2, 2, 2, 2, 2, 2, 2, 2, 2, 2, 2, 2, 2, 2, 2, 3 ),
 ( 0.000000000000000000, 1.000000000000000000 ),
 ( 0.000000000000000000, 0.005747126436781609116, 0.01149425287356321823, 0.01724137931034482735, 0.02298850574712643646, 0.02873563218390804558, 0.03448275862068965469, 0.04022988505747126381, 0.04597701149425287293, 0.05172413793103448204, 0.05747126436781609116, 0.06321839080459770721, 0.06896551724137930939, 0.07471264367816092544, 0.08045977011494252762, 0.08620689655172414367, 0.09195402298850574585, 0.09770114942528736190, 0.1034482758620689641, 0.1091954022988505801, 0.1149425287356321823, 0.1206896551724137984, 0.1264367816091954144, 0.1321839080459770166, 0.1379310344827586188, 0.1436781609195402210, 0.1494252873563218509, 0.1551724137931034531, 0.1609195402298850552, 0.1666666666666666574, 0.1724137931034482873, 0.1781609195402298895, 0.1839080459770114917, 0.1896551724137930939, 0.1954022988505747238, 0.2011494252873563260, 0.2068965517241379282, 0.2126436781609195303, 0.2183908045977011603, 0.2241379310344827624, 0.2298850574712643646, 0.2356321839080459668, 0.2413793103448275967, 0.2471264367816091989, 0.2528735632183908288, 0.2586206896551724310, 0.2643678160919540332, 0.2701149425287356354, 0.2758620689655172376, 0.2816091954022988397, 0.2873563218390804419, 0.2931034482758620441, 0.2988505747126437018, 0.3045977011494253039, 0.3103448275862069061, 0.3160919540229885083, 0.3218390804597701105, 0.3275862068965517127, 0.3333333333333333148, 0.3390804597701149170, 0.3448275862068965747, 0.3505747126436781769, 0.3563218390804597790, 0.3620689655172413812, 0.3678160919540229834, 0.3735632183908045856, 0.3793103448275861878, 0.3850574712643677899, 0.3908045977011494476, 0.3965517241379310498, 0.4022988505747126520, 0.4080459770114942541, 0.4137931034482758563, 0.4195402298850574585, 0.4252873563218390607, 0.4310344827586206629, 0.4367816091954023205, 0.4425287356321839227, 0.4482758620689655249, 0.4540229885057471271, 0.4597701149425287293, 0.4655172413793103314, 0.4712643678160919336, 0.4770114942528735358, 0.4827586206896551935, 0.4885057471264367956, 0.4942528735632183978, 0.5000000000000000000, 0.5057471264367816577, 0.5114942528735632044, 0.5172413793103448620, 0.5229885057471264087, 0.5287356321839080664, 0.5344827586206896131, 0.5402298850574712707, 0.5459770114942529284, 0.5517241379310344751, 0.5574712643678161328, 0.5632183908045976795, 0.5689655172413793371, 0.5747126436781608838, 0.5804597701149425415, 0.5862068965517240882, 0.5919540229885057459, 0.5977011494252874035, 0.6034482758620689502, 0.6091954022988506079, 0.6149425287356321546, 0.6206896551724138122, 0.6264367816091953589, 0.6321839080459770166, 0.6379310344827586743, 0.6436781609195402210, 0.6494252873563218786, 0.6551724137931034253, 0.6609195402298850830, 0.6666666666666666297, 0.6724137931034482873, 0.6781609195402298340, 0.6839080459770114917, 0.6896551724137931494, 0.6954022988505746961, 0.7011494252873563537, 0.7068965517241379004, 0.7126436781609195581, 0.7183908045977011048, 0.7241379310344827624, 0.7298850574712644201, 0.7356321839080459668, 0.7413793103448276245, 0.7471264367816091712, 0.7528735632183908288, 0.7586206896551723755, 0.7643678160919540332, 0.7701149425287355799, 0.7758620689655172376, 0.7816091954022988952, 0.7873563218390804419, 0.7931034482758620996, 0.7988505747126436463, 0.8045977011494253039, 0.8103448275862068506, 0.8160919540229885083, 0.8218390804597701660, 0.8275862068965517127, 0.8333333333333333703, 0.8390804597701149170, 0.8448275862068965747, 0.8505747126436781214, 0.8563218390804597790, 0.8620689655172413257, 0.8678160919540229834, 0.8735632183908046411, 0.8793103448275861878, 0.8850574712643678454, 0.8908045977011493921, 0.8965517241379310498, 0.9022988505747125965, 0.9080459770114942541, 0.9137931034482759118, 0.9195402298850574585, 0.9252873563218391162, 0.9310344827586206629, 0.9367816091954023205, 0.9425287356321838672, 0.9482758620689655249, 0.9540229885057470716, 0.9597701149425287293, 0.9655172413793103869, 0.9712643678160919336, 0.9770114942528735913, 0.9827586206896551380, 0.9885057471264367956, 0.9942528735632183423, 0.9961881835133211682 ),
 .UNSPECIFIED. ) 
 GEOMETRIC_REPRESENTATION_ITEM ( )  RATIONAL_B_SPLINE_SURFACE ( (
 ( 1.000000000000000000, 0.8660254037844387076, 1.000000000000000000, 0.8660254037844387076, 1.000000000000000000, 0.8660254037844387076, 1.000000000000000000, 0.8660254037844387076, 1.000000000000000000, 0.8660254037844387076, 1.000000000000000000, 0.8660254037844387076, 1.000000000000000000, 0.8660254037844387076, 1.000000000000000000, 0.8660254037844387076, 1.000000000000000000, 0.8660254037844387076, 1.000000000000000000, 0.8660254037844387076, 1.000000000000000000, 0.8660254037844387076, 1.000000000000000000, 0.8660254037844387076, 1.000000000000000000, 0.8660254037844387076, 1.000000000000000000, 0.8660254037844387076, 1.000000000000000000, 0.8660254037844387076, 1.000000000000000000, 0.8660254037844387076, 1.000000000000000000, 0.8660254037844387076, 1.000000000000000000, 0.8660254037844387076, 1.000000000000000000, 0.8660254037844387076, 1.000000000000000000, 0.8660254037844387076, 1.000000000000000000, 0.8660254037844387076, 1.000000000000000000, 0.8660254037844387076, 1.000000000000000000, 0.8660254037844387076, 1.000000000000000000, 0.8660254037844387076, 1.000000000000000000, 0.8660254037844387076, 1.000000000000000000, 0.8660254037844387076, 1.000000000000000000, 0.8660254037844387076, 1.000000000000000000, 0.8660254037844387076, 1.000000000000000000, 0.8660254037844387076, 1.000000000000000000, 0.8660254037844387076, 1.000000000000000000, 0.8660254037844387076, 1.000000000000000000, 0.8660254037844387076, 1.000000000000000000, 0.8660254037844387076, 1.000000000000000000, 0.8660254037844387076, 1.000000000000000000, 0.8660254037844387076, 1.000000000000000000, 0.8660254037844387076, 1.000000000000000000, 0.8660254037844387076, 1.000000000000000000, 0.8660254037844387076, 1.000000000000000000, 0.8660254037844387076, 1.000000000000000000, 0.8660254037844387076, 1.000000000000000000, 0.8660254037844387076, 1.000000000000000000, 0.8660254037844387076, 1.000000000000000000, 0.8660254037844387076, 1.000000000000000000, 0.8660254037844387076, 1.000000000000000000, 0.8660254037844387076, 1.000000000000000000, 0.8660254037844387076, 1.000000000000000000, 0.8660254037844387076, 1.000000000000000000, 0.8660254037844387076, 1.000000000000000000, 0.8660254037844387076, 1.000000000000000000, 0.8660254037844387076, 1.000000000000000000, 0.8660254037844387076, 1.000000000000000000, 0.8660254037844387076, 1.000000000000000000, 0.8660254037844387076, 1.000000000000000000, 0.8660254037844387076, 1.000000000000000000, 0.8660254037844387076, 1.000000000000000000, 0.8660254037844387076, 1.000000000000000000, 0.8660254037844387076, 1.000000000000000000, 0.8660254037844387076, 1.000000000000000000, 0.8660254037844387076, 1.000000000000000000, 0.8660254037844387076, 1.000000000000000000, 0.8660254037844387076, 1.000000000000000000, 0.8660254037844387076, 1.000000000000000000, 0.8660254037844387076, 1.000000000000000000, 0.8660254037844387076, 1.000000000000000000, 0.8660254037844387076, 1.000000000000000000, 0.8660254037844387076, 1.000000000000000000, 0.8660254037844387076, 1.000000000000000000, 0.8660254037844387076, 1.000000000000000000, 0.8660254037844387076, 1.000000000000000000, 0.8660254037844387076, 1.000000000000000000, 0.8660254037844387076, 1.000000000000000000, 0.8660254037844387076, 1.000000000000000000, 0.8660254037844387076, 1.000000000000000000, 0.8660254037844387076, 1.000000000000000000, 0.8660254037844387076, 1.000000000000000000, 0.8660254037844387076, 1.000000000000000000, 0.8660254037844387076, 1.000000000000000000, 0.8660254037844387076, 1.000000000000000000, 0.8660254037844387076, 1.000000000000000000, 0.8660254037844387076, 1.000000000000000000, 0.8660254037844387076, 1.000000000000000000, 0.8660254037844387076, 1.000000000000000000, 0.8660254037844387076, 1.000000000000000000, 0.8660254037844387076, 1.000000000000000000, 0.8660254037844387076, 1.000000000000000000, 0.8660254037844387076, 1.000000000000000000, 0.8660254037844387076, 1.000000000000000000, 0.8660254037844387076, 1.000000000000000000, 0.8660254037844387076, 1.000000000000000000, 0.8660254037844387076, 1.000000000000000000, 0.8660254037844387076, 1.000000000000000000, 0.8660254037844387076, 1.000000000000000000, 0.8660254037844387076, 1.000000000000000000, 0.8660254037844387076, 1.000000000000000000, 0.8660254037844387076, 1.000000000000000000, 0.8660254037844387076, 1.000000000000000000, 0.8660254037844387076, 1.000000000000000000, 0.8660254037844387076, 1.000000000000000000, 0.8660254037844387076, 1.000000000000000000, 0.8660254037844387076, 1.000000000000000000, 0.8660254037844387076, 1.000000000000000000, 0.8660254037844387076, 1.000000000000000000, 0.8660254037844387076, 1.000000000000000000, 0.8660254037844387076, 1.000000000000000000, 0.8660254037844387076, 1.000000000000000000, 0.8660254037844387076, 1.000000000000000000, 0.8660254037844387076, 1.000000000000000000, 0.8660254037844387076, 1.000000000000000000, 0.8660254037844387076, 1.000000000000000000, 0.8660254037844387076, 1.000000000000000000, 0.8660254037844387076, 1.000000000000000000, 0.8660254037844387076, 1.000000000000000000, 0.8660254037844387076, 1.000000000000000000, 0.8660254037844387076, 1.000000000000000000, 0.8660254037844387076, 1.000000000000000000, 0.8660254037844387076, 1.000000000000000000, 0.8660254037844387076, 1.000000000000000000, 0.8660254037844387076, 1.000000000000000000, 0.8660254037844387076, 1.000000000000000000, 0.8660254037844387076, 1.000000000000000000, 0.8660254037844387076, 1.000000000000000000, 0.8660254037844387076, 1.000000000000000000, 0.8660254037844387076, 1.000000000000000000, 0.8660254037844387076, 1.000000000000000000, 0.8660254037844387076, 1.000000000000000000, 0.8660254037844387076, 1.000000000000000000, 0.8660254037844387076, 1.000000000000000000, 0.8660254037844387076, 1.000000000000000000, 0.8660254037844387076, 1.000000000000000000, 0.8660254037844387076, 1.000000000000000000, 0.8660254037844387076, 1.000000000000000000, 0.8660254037844387076, 1.000000000000000000, 0.8660254037844387076, 1.000000000000000000, 0.8660254037844387076, 1.000000000000000000, 0.8660254037844387076, 1.000000000000000000, 0.8660254037844387076, 1.000000000000000000, 0.8660254037844387076, 1.000000000000000000, 0.8660254037844387076, 1.000000000000000000, 0.8660254037844387076, 1.000000000000000000, 0.8660254037844387076, 1.000000000000000000, 0.8660254037844387076, 1.000000000000000000, 0.8660254037844387076, 1.000000000000000000, 0.8660254037844387076, 1.000000000000000000, 0.8660254037844387076, 1.000000000000000000, 0.8660254037844387076, 1.000000000000000000, 0.8660254037844387076, 1.000000000000000000, 0.8660254037844387076, 1.000000000000000000, 0.8660254037844387076, 1.000000000000000000, 0.8660254037844387076, 1.000000000000000000, 0.8660254037844387076, 1.000000000000000000, 0.8660254037844387076, 1.000000000000000000, 0.8660254037844387076, 1.000000000000000000, 0.8660254037844387076, 1.000000000000000000, 0.8660254037844387076, 1.000000000000000000, 0.8660254037844387076, 1.000000000000000000, 0.8660254037844387076, 1.000000000000000000, 0.8660254037844387076, 1.000000000000000000, 0.8660254037844387076, 1.000000000000000000, 0.8660254037844387076, 1.000000000000000000, 0.8660254037844387076, 1.000000000000000000, 0.8660254037844387076, 1.000000000000000000, 0.8660254037844387076, 1.000000000000000000, 0.8660254037844387076, 1.000000000000000000, 0.8660254037844387076, 1.000000000000000000, 0.8660254037844387076, 1.000000000000000000, 0.8660254037844387076, 1.000000000000000000, 0.8660254037844387076, 1.000000000000000000, 0.8660254037844387076, 1.000000000000000000, 0.8660254037844387076, 1.000000000000000000, 0.8660254037844387076, 1.000000000000000000, 0.8660254037844387076, 1.000000000000000000, 0.8660254037844387076, 1.000000000000000000, 0.8660254037844387076, 1.000000000000000000, 0.9548848677736452295, 0.9401542295229485813),
 ( 1.000000000000000000, 0.8660254037844387076, 1.000000000000000000, 0.8660254037844387076, 1.000000000000000000, 0.8660254037844387076, 1.000000000000000000, 0.8660254037844387076, 1.000000000000000000, 0.8660254037844387076, 1.000000000000000000, 0.8660254037844387076, 1.000000000000000000, 0.8660254037844387076, 1.000000000000000000, 0.8660254037844387076, 1.000000000000000000, 0.8660254037844387076, 1.000000000000000000, 0.8660254037844387076, 1.000000000000000000, 0.8660254037844387076, 1.000000000000000000, 0.8660254037844387076, 1.000000000000000000, 0.8660254037844387076, 1.000000000000000000, 0.8660254037844387076, 1.000000000000000000, 0.8660254037844387076, 1.000000000000000000, 0.8660254037844387076, 1.000000000000000000, 0.8660254037844387076, 1.000000000000000000, 0.8660254037844387076, 1.000000000000000000, 0.8660254037844387076, 1.000000000000000000, 0.8660254037844387076, 1.000000000000000000, 0.8660254037844387076, 1.000000000000000000, 0.8660254037844387076, 1.000000000000000000, 0.8660254037844387076, 1.000000000000000000, 0.8660254037844387076, 1.000000000000000000, 0.8660254037844387076, 1.000000000000000000, 0.8660254037844387076, 1.000000000000000000, 0.8660254037844387076, 1.000000000000000000, 0.8660254037844387076, 1.000000000000000000, 0.8660254037844387076, 1.000000000000000000, 0.8660254037844387076, 1.000000000000000000, 0.8660254037844387076, 1.000000000000000000, 0.8660254037844387076, 1.000000000000000000, 0.8660254037844387076, 1.000000000000000000, 0.8660254037844387076, 1.000000000000000000, 0.8660254037844387076, 1.000000000000000000, 0.8660254037844387076, 1.000000000000000000, 0.8660254037844387076, 1.000000000000000000, 0.8660254037844387076, 1.000000000000000000, 0.8660254037844387076, 1.000000000000000000, 0.8660254037844387076, 1.000000000000000000, 0.8660254037844387076, 1.000000000000000000, 0.8660254037844387076, 1.000000000000000000, 0.8660254037844387076, 1.000000000000000000, 0.8660254037844387076, 1.000000000000000000, 0.8660254037844387076, 1.000000000000000000, 0.8660254037844387076, 1.000000000000000000, 0.8660254037844387076, 1.000000000000000000, 0.8660254037844387076, 1.000000000000000000, 0.8660254037844387076, 1.000000000000000000, 0.8660254037844387076, 1.000000000000000000, 0.8660254037844387076, 1.000000000000000000, 0.8660254037844387076, 1.000000000000000000, 0.8660254037844387076, 1.000000000000000000, 0.8660254037844387076, 1.000000000000000000, 0.8660254037844387076, 1.000000000000000000, 0.8660254037844387076, 1.000000000000000000, 0.8660254037844387076, 1.000000000000000000, 0.8660254037844387076, 1.000000000000000000, 0.8660254037844387076, 1.000000000000000000, 0.8660254037844387076, 1.000000000000000000, 0.8660254037844387076, 1.000000000000000000, 0.8660254037844387076, 1.000000000000000000, 0.8660254037844387076, 1.000000000000000000, 0.8660254037844387076, 1.000000000000000000, 0.8660254037844387076, 1.000000000000000000, 0.8660254037844387076, 1.000000000000000000, 0.8660254037844387076, 1.000000000000000000, 0.8660254037844387076, 1.000000000000000000, 0.8660254037844387076, 1.000000000000000000, 0.8660254037844387076, 1.000000000000000000, 0.8660254037844387076, 1.000000000000000000, 0.8660254037844387076, 1.000000000000000000, 0.8660254037844387076, 1.000000000000000000, 0.8660254037844387076, 1.000000000000000000, 0.8660254037844387076, 1.000000000000000000, 0.8660254037844387076, 1.000000000000000000, 0.8660254037844387076, 1.000000000000000000, 0.8660254037844387076, 1.000000000000000000, 0.8660254037844387076, 1.000000000000000000, 0.8660254037844387076, 1.000000000000000000, 0.8660254037844387076, 1.000000000000000000, 0.8660254037844387076, 1.000000000000000000, 0.8660254037844387076, 1.000000000000000000, 0.8660254037844387076, 1.000000000000000000, 0.8660254037844387076, 1.000000000000000000, 0.8660254037844387076, 1.000000000000000000, 0.8660254037844387076, 1.000000000000000000, 0.8660254037844387076, 1.000000000000000000, 0.8660254037844387076, 1.000000000000000000, 0.8660254037844387076, 1.000000000000000000, 0.8660254037844387076, 1.000000000000000000, 0.8660254037844387076, 1.000000000000000000, 0.8660254037844387076, 1.000000000000000000, 0.8660254037844387076, 1.000000000000000000, 0.8660254037844387076, 1.000000000000000000, 0.8660254037844387076, 1.000000000000000000, 0.8660254037844387076, 1.000000000000000000, 0.8660254037844387076, 1.000000000000000000, 0.8660254037844387076, 1.000000000000000000, 0.8660254037844387076, 1.000000000000000000, 0.8660254037844387076, 1.000000000000000000, 0.8660254037844387076, 1.000000000000000000, 0.8660254037844387076, 1.000000000000000000, 0.8660254037844387076, 1.000000000000000000, 0.8660254037844387076, 1.000000000000000000, 0.8660254037844387076, 1.000000000000000000, 0.8660254037844387076, 1.000000000000000000, 0.8660254037844387076, 1.000000000000000000, 0.8660254037844387076, 1.000000000000000000, 0.8660254037844387076, 1.000000000000000000, 0.8660254037844387076, 1.000000000000000000, 0.8660254037844387076, 1.000000000000000000, 0.8660254037844387076, 1.000000000000000000, 0.8660254037844387076, 1.000000000000000000, 0.8660254037844387076, 1.000000000000000000, 0.8660254037844387076, 1.000000000000000000, 0.8660254037844387076, 1.000000000000000000, 0.8660254037844387076, 1.000000000000000000, 0.8660254037844387076, 1.000000000000000000, 0.8660254037844387076, 1.000000000000000000, 0.8660254037844387076, 1.000000000000000000, 0.8660254037844387076, 1.000000000000000000, 0.8660254037844387076, 1.000000000000000000, 0.8660254037844387076, 1.000000000000000000, 0.8660254037844387076, 1.000000000000000000, 0.8660254037844387076, 1.000000000000000000, 0.8660254037844387076, 1.000000000000000000, 0.8660254037844387076, 1.000000000000000000, 0.8660254037844387076, 1.000000000000000000, 0.8660254037844387076, 1.000000000000000000, 0.8660254037844387076, 1.000000000000000000, 0.8660254037844387076, 1.000000000000000000, 0.8660254037844387076, 1.000000000000000000, 0.8660254037844387076, 1.000000000000000000, 0.8660254037844387076, 1.000000000000000000, 0.8660254037844387076, 1.000000000000000000, 0.8660254037844387076, 1.000000000000000000, 0.8660254037844387076, 1.000000000000000000, 0.8660254037844387076, 1.000000000000000000, 0.8660254037844387076, 1.000000000000000000, 0.8660254037844387076, 1.000000000000000000, 0.8660254037844387076, 1.000000000000000000, 0.8660254037844387076, 1.000000000000000000, 0.8660254037844387076, 1.000000000000000000, 0.8660254037844387076, 1.000000000000000000, 0.8660254037844387076, 1.000000000000000000, 0.8660254037844387076, 1.000000000000000000, 0.8660254037844387076, 1.000000000000000000, 0.8660254037844387076, 1.000000000000000000, 0.8660254037844387076, 1.000000000000000000, 0.8660254037844387076, 1.000000000000000000, 0.8660254037844387076, 1.000000000000000000, 0.8660254037844387076, 1.000000000000000000, 0.8660254037844387076, 1.000000000000000000, 0.8660254037844387076, 1.000000000000000000, 0.8660254037844387076, 1.000000000000000000, 0.8660254037844387076, 1.000000000000000000, 0.8660254037844387076, 1.000000000000000000, 0.8660254037844387076, 1.000000000000000000, 0.8660254037844387076, 1.000000000000000000, 0.8660254037844387076, 1.000000000000000000, 0.8660254037844387076, 1.000000000000000000, 0.8660254037844387076, 1.000000000000000000, 0.8660254037844387076, 1.000000000000000000, 0.8660254037844387076, 1.000000000000000000, 0.8660254037844387076, 1.000000000000000000, 0.8660254037844387076, 1.000000000000000000, 0.8660254037844387076, 1.000000000000000000, 0.8660254037844387076, 1.000000000000000000, 0.8660254037844387076, 1.000000000000000000, 0.8660254037844387076, 1.000000000000000000, 0.8660254037844387076, 1.000000000000000000, 0.8660254037844387076, 1.000000000000000000, 0.9548848677736452295, 0.9401542295229485813) ) ) 
 REPRESENTATION_ITEM ( '' )  SURFACE ( )  );
#12395=CARTESIAN_POINT ( 'NONE',  ( 4.000000000000000888, -22.36774190952427688, -7.662965955988220834 ) ) ;
#12399=VERTEX_POINT ( 'NONE', #16169 ) ;
#12400=CARTESIAN_POINT ( 'NONE',  ( 4.243569643749997233, -27.09021171885596146, -10.13586168944375387 ) ) ;
#12403=CARTESIAN_POINT ( 'NONE',  ( 4.000000000000003553, -19.09940784846689610, -7.021619088400267827 ) ) ;
#12408=CIRCLE ( 'NONE', #10988, 2.000000000000001776 ) ;
#12409=CARTESIAN_POINT ( 'NONE',  ( -8.500000000000005329, 10.00000000000000000, 20.49999999999999645 ) ) ;
#12410=CARTESIAN_POINT ( 'NONE',  ( 4.730628863548789710E-15, -19.17657787239344458, -11.64849162045545583 ) ) ;
#12412=CARTESIAN_POINT ( 'NONE',  ( -3.113145992481321400, -29.13892139834124606, -12.87460258714478911 ) ) ;
#12414=CARTESIAN_POINT ( 'NONE',  ( 4.713407268011036227E-15, -21.35891669415256899, -14.27485004966103510 ) ) ;
#12415=CARTESIAN_POINT ( 'NONE',  ( 1.071796769724485454, -21.81280909414084235, -13.84422694430704226 ) ) ;
#12418=VERTEX_POINT ( 'NONE', #8079 ) ;
#12421=CARTESIAN_POINT ( 'NONE',  ( -4.243569643750000786, -19.99636183013295820, -4.276284222377527477 ) ) ;
#12424=CARTESIAN_POINT ( 'NONE',  ( 4.713407268011036227E-15, -20.52006115528422825, -13.07684018388161817 ) ) ;
#12426=EDGE_CURVE ( 'NONE', #8485, #8354, #5210, .T. ) ;
#12428=CARTESIAN_POINT ( 'NONE',  ( 4.243569643750000786, -20.41578959921466918, -4.875289154763852828 ) ) ;
#12430=ADVANCED_FACE ( 'NONE', ( #774 ), #7807, .F. ) ;
#12431=CARTESIAN_POINT ( 'NONE',  ( 1.533898589781675205E-14, -27.51564321027552040, -8.041143755076902266 ) ) ;
#12432=CARTESIAN_POINT ( 'NONE',  ( 4.243569643749997233, -26.79983864795324422, -9.721165967022450616 ) ) ;
#12434=CARTESIAN_POINT ( 'NONE',  ( 4.000000000000000888, -21.33530432409240163, -6.188492276268029890 ) ) ;
#12436=EDGE_LOOP ( 'NONE', ( #13782, #17880, #5019, #10915, #9917, #2029 ) ) ;
#12439=CARTESIAN_POINT ( 'NONE',  ( -1.071796769724486786, -18.69244293640756283, -9.387882235834636546 ) ) ;
#12445=CARTESIAN_POINT ( 'NONE',  ( -4.243569643749997233, -21.88256802303096293, -11.24155594871087338 ) ) ;
#12449=CARTESIAN_POINT ( 'NONE',  ( 4.730628863548789710E-15, -19.69279666510938043, -12.38572846031554953 ) ) ;
#12451=CARTESIAN_POINT ( 'NONE',  ( 2.319183558094505493, -24.28745349265258469, -16.12279146867029667 ) ) ;
#12452=CARTESIAN_POINT ( 'NONE',  ( 1.533898589781675205E-14, -27.25753381391755426, -7.672525335146852754 ) ) ;
#12453=CARTESIAN_POINT ( 'NONE',  ( -4.243569643749997233, -19.81769285216720888, -8.292608589270493269 ) ) ;
#12457=AXIS2_PLACEMENT_3D ( 'NONE', #18272, #6572, #1024 ) ;
#12461=VECTOR ( 'NONE', #1606, 1000.000000000000000 ) ;
#12464=EDGE_LOOP ( 'NONE', ( #2856, #7314, #9571, #104 ) ) ;
#12465=CARTESIAN_POINT ( 'NONE',  ( 2.121784821874994176, -24.24355182426693389, -3.934664979292979314 ) ) ;
#12468=DIRECTION ( 'NONE',  ( -0.000000000000000000, -0.5735764363510414965, -0.8191520442889950182 ) ) ;
#12470=CARTESIAN_POINT ( 'NONE',  ( 4.243569643750000786, -26.57815143726116602, -13.67605393059374208 ) ) ;
#12474=CARTESIAN_POINT ( 'NONE',  ( -3.999999999999997335, -20.11033631824054524, -8.465374567466390943 ) ) ;
#12476=EDGE_CURVE ( 'NONE', #17908, #12048, #1740, .T. ) ;
#12477=ORIENTED_EDGE ( 'NONE', *, *, #2424, .T. ) ;
#12478=CARTESIAN_POINT ( 'NONE',  ( 4.299564228933482956E-15, -22.89824732864832768, -15.39439339536058959 ) ) ;
#12480=ADVANCED_FACE ( 'NONE', ( #9201 ), #16541, .F. ) ;
#12483=VECTOR ( 'NONE', #6145, 1000.000000000000000 ) ;
#12487=CARTESIAN_POINT ( 'NONE',  ( -2.121784821874996396, -22.48152525766933962, -14.23270058530414950 ) ) ;
#12490=CARTESIAN_POINT ( 'NONE',  ( 4.000000000000003553, -18.84129845210892640, -6.653000668470220980 ) ) ;
#12492=DIRECTION ( 'NONE',  ( 1.000000000000000000, -0.000000000000000000, -0.000000000000000000 ) ) ;
#12498=( BOUNDED_CURVE ( )  B_SPLINE_CURVE ( 2, ( #8166, #8676, #3909, #18028, #2446, #8077, #14168, #5907, #10068 ),
 .UNSPECIFIED., .F., .T. ) 
 B_SPLINE_CURVE_WITH_KNOTS ( ( 3, 2, 2, 2, 3 ),
 ( 0.8706896551724138122, 0.8735632183908046411, 0.8793103448275861878, 0.8850574712643678454, 0.8879310344827586743 ),
 .UNSPECIFIED. ) 
 CURVE ( )  GEOMETRIC_REPRESENTATION_ITEM ( )  RATIONAL_B_SPLINE_CURVE ( ( 0.9330127018922194093, 0.9330127018922194093, 1.000000000000000000, 0.8660254037844387076, 1.000000000000000000, 0.8660254037844387076, 1.000000000000000000, 0.9330127018922180770, 0.9330127018922194093 ) ) 
 REPRESENTATION_ITEM ( '' )  );
#12499=CARTESIAN_POINT ( 'NONE',  ( -2.121784821875005722, -25.83522643514106676, -6.207811902194944054 ) ) ;
#12502=VERTEX_POINT ( 'NONE', #17671 ) ;
#12504=CARTESIAN_POINT ( 'NONE',  ( -2.000000000000005773, -27.87249825822150839, -9.485095902363450904 ) ) ;
#12506=PLANE ( 'NONE',  #10143 ) ;
#12511=CARTESIAN_POINT ( 'NONE',  ( -4.000000000000004441, -28.23867904981954879, -12.02121522353072969 ) ) ;
#12517=CARTESIAN_POINT ( 'NONE',  ( -2.000000000000005773, -27.03364271935316765, -8.287086036584028648 ) ) ;
#12518=ORIENTED_EDGE ( 'NONE', *, *, #9880, .F. ) ;
#12519=CARTESIAN_POINT ( 'NONE',  ( 3.999999999999996891, -2.343145750507611869, 16.84997118393183513 ) ) ;
#12521=CARTESIAN_POINT ( 'NONE',  ( -4.000000000000004441, -26.17380387895579830, -9.072267864090346023 ) ) ;
#12522=CARTESIAN_POINT ( 'NONE',  ( 4.243569643750003451, -20.41994811033580959, -9.152718235773933841 ) ) ;
#12525=AXIS2_PLACEMENT_3D ( 'NONE', #578, #478, #8899 ) ;
#12526=CARTESIAN_POINT ( 'NONE',  ( -5.577813053751546416E-15, -24.35380310418546657, -3.525568109927051275 ) ) ;
#12532=DIRECTION ( 'NONE',  ( 0.8191520442889951292, 0.4698463103929519935, -0.3289899283371605643 ) ) ;
#12536=CARTESIAN_POINT ( 'NONE',  ( -4.243569643750005227, -26.36965632068995191, -9.106801933805707350 ) ) ;
#12541=VECTOR ( 'NONE', #419, 1000.000000000000000 ) ;
#12542=CARTESIAN_POINT ( 'NONE',  ( 4.243569643750003451, -21.48464937031242883, -10.67326921798538386 ) ) ;
#12548=CARTESIAN_POINT ( 'NONE',  ( -2.121784821875005722, -25.28674396788038337, -5.424497759843593059 ) ) ;
#12550=CARTESIAN_POINT ( 'NONE',  ( -1.071796769724496334, -25.20418534377263953, -4.740039810362389083 ) ) ;
#12551=CARTESIAN_POINT ( 'NONE',  ( 8.500000000000019540, 0.000000000000000000, 20.49999999999998934 ) ) ;
#12554=CARTESIAN_POINT ( 'NONE',  ( -3.706921591972381904E-14, -18.96207903348436119, -9.772962490420598058 ) ) ;
#12556=DIRECTION ( 'NONE',  ( 0.000000000000000000, -0.5735764363510414965, -0.8191520442889950182 ) ) ;
#12558=CARTESIAN_POINT ( 'NONE',  ( -8.500000000000005329, -1.201721234452885367, 20.49999999999999645 ) ) ;
#12560=ORIENTED_EDGE ( 'NONE', *, *, #11082, .T. ) ;
#12561=CARTESIAN_POINT ( 'NONE',  ( 2.121784821875004390, -18.91101194138411046, -9.133479109605152857 ) ) ;
#12566=CARTESIAN_POINT ( 'NONE',  ( 4.898587196589413815E-16, 2.700915433685006750, 35.11257424290206330 ) ) ;
#12567=CARTESIAN_POINT ( 'NONE',  ( -4.243569643749997233, -23.43122440117877048, -13.45326646829115980 ) ) ;
#12568=EDGE_LOOP ( 'NONE', ( #9721, #2722, #1120, #10166 ) ) ;
#12570=CARTESIAN_POINT ( 'NONE',  ( -3.999999999999997335, -19.59411752552460584, -7.728137727606295471 ) ) ;
#12573=CARTESIAN_POINT ( 'NONE',  ( 4.000000000000000888, -25.46505466581989907, -12.08638699514879455 ) ) ;
#12579=CARTESIAN_POINT ( 'NONE',  ( 4.243569643749997233, -27.60643051157189731, -10.87309852930384935 ) ) ;
#12581=VERTEX_POINT ( 'NONE', #16817 ) ;
#12584=CARTESIAN_POINT ( 'NONE',  ( 4.299564228933482956E-15, -20.83337215778458074, -12.44544603592020771 ) ) ;
#12587=CARTESIAN_POINT ( 'NONE',  ( -8.500000000000005329, 0.000000000000000000, -20.49999999999999645 ) ) ;
#12588=CARTESIAN_POINT ( 'NONE',  ( -5.330712181944245322E-15, -27.07529864955322552, -5.843073507603255834 ) ) ;
#12591=ORIENTED_EDGE ( 'NONE', *, *, #6035, .T. ) ;
#12592=CARTESIAN_POINT ( 'NONE',  ( 4.000000000000003553, -23.29368553998883229, -13.01166841327030710 ) ) ;
#12597=CARTESIAN_POINT ( 'NONE',  ( -1.999999999999996225, -23.31572046977624169, -15.05629650786418772 ) ) ;
#12600=CARTESIAN_POINT ( 'NONE',  ( 3.999999999999996447, -25.50702127099278371, -8.120003611597617521 ) ) ;
#12602=EDGE_CURVE ( 'NONE', #13230, #13289, #14918, .T. ) ;
#12604=CARTESIAN_POINT ( 'NONE',  ( 2.769796806539087886, -22.38185710306395748, -1.928164938508226234 ) ) ;
#12607=( BOUNDED_CURVE ( )  B_SPLINE_CURVE ( 2, ( #918, #6918, #8220, #13699, #12573, #18082, #5531, #13969, #6830 ),
 .UNSPECIFIED., .F., .F. ) 
 B_SPLINE_CURVE_WITH_KNOTS ( ( 3, 2, 2, 2, 3 ),
 ( 0.1982758620689655249, 0.2011494252873563260, 0.2068965517241379282, 0.2126436781609195303, 0.2155172413793103592 ),
 .UNSPECIFIED. ) 
 CURVE ( )  GEOMETRIC_REPRESENTATION_ITEM ( )  RATIONAL_B_SPLINE_CURVE ( ( 0.9330127018922194093, 0.9330127018922194093, 1.000000000000000000, 0.8660254037844387076, 1.000000000000000000, 0.8660254037844387076, 1.000000000000000000, 0.9330127018922189652, 0.9330127018922192983 ) ) 
 REPRESENTATION_ITEM ( '' )  );
#12608=CIRCLE ( 'NONE', #4614, 6.000000000000000000 ) ;
#12609=CARTESIAN_POINT ( 'NONE',  ( -3.999999999999997335, -22.43332088546226544, -11.78294034683682057 ) ) ;
#12610=CARTESIAN_POINT ( 'NONE',  ( -5.330712181944246111E-15, -27.30114437136644767, -6.165614625042047159 ) ) ;
#12612=CARTESIAN_POINT ( 'NONE',  ( 3.999999999999996447, 6.938893903907228378E-15, 0.000000000000000000 ) ) ;
#12615=ORIENTED_EDGE ( 'NONE', *, *, #14025, .T. ) ;
#12616=ORIENTED_EDGE ( 'NONE', *, *, #3630, .T. ) ;
#12618=CARTESIAN_POINT ( 'NONE',  ( -1.071796769724477238, -25.13965799397821144, -4.647885204373104706 ) ) ;
#12619=CARTESIAN_POINT ( 'NONE',  ( -3.999999999999997335, -24.24008665996804268, -14.36326928634715649 ) ) ;
#12620=CARTESIAN_POINT ( 'NONE',  ( 4.000000000000000888, -21.07719492773443193, -5.819873856337981266 ) ) ;
#12621=CARTESIAN_POINT ( 'NONE',  ( -4.648177544792955347E-16, -30.09673717385520675, -11.72732795437737785 ) ) ;
#12624=CARTESIAN_POINT ( 'NONE',  ( 2.121784821875004390, -19.39496705955529876, -9.824638646973991030 ) ) ;
#12630=CARTESIAN_POINT ( 'NONE',  ( -4.243569643749997233, -21.91483169757570693, -11.28763325120213068 ) ) ;
#12631=AXIS2_PLACEMENT_3D ( 'NONE', #2241, #7591, #12041 ) ;
#12632=LINE ( 'NONE', #2646, #1999 ) ;
#12634=DIRECTION ( 'NONE',  ( 0.000000000000000000, 0.000000000000000000, -1.000000000000000000 ) ) ;
#12637=CARTESIAN_POINT ( 'NONE',  ( -2.121784821874996396, -17.02896425960724969, -6.445636464281891520 ) ) ;
#12640=EDGE_LOOP ( 'NONE', ( #18183, #3946, #695, #3487 ) ) ;
#12642=CARTESIAN_POINT ( 'NONE',  ( 4.299564228933482956E-15, -16.96173121241504944, -6.916169736969493442 ) ) ;
#12644=CARTESIAN_POINT ( 'NONE',  ( -10.00530551168418825, -9.915183271925439357, 7.312645477306290331 ) ) ;
#12645=ORIENTED_EDGE ( 'NONE', *, *, #947, .F. ) ;
#12646=CARTESIAN_POINT ( 'NONE',  ( -2.121784821875005722, -22.99602307520341427, -2.153009282964420290 ) ) ;
#12651=FACE_OUTER_BOUND ( 'NONE', #13262, .T. ) ;
#12654=CARTESIAN_POINT ( 'NONE',  ( 4.000000000000000888, -26.43296490145733557, -13.46870606887970645 ) ) ;
#12656=CARTESIAN_POINT ( 'NONE',  ( -4.243569643750005227, -28.69264088791166856, -12.42436771317613875 ) ) ;
#12659=CARTESIAN_POINT ( 'NONE',  ( 4.713407268011036227E-15, -18.51971333421491295, -10.22004743043051000 ) ) ;
#12668=EDGE_LOOP ( 'NONE', ( #18275, #15471, #8038, #16154 ) ) ;
#12669=CARTESIAN_POINT ( 'NONE',  ( 4.243569643749997233, -27.86453990792986701, -11.24171694923389531 ) ) ;
#12675=VECTOR ( 'NONE', #4349, 1000.000000000000000 ) ;
#12679=CARTESIAN_POINT ( 'NONE',  ( 1.071796769724495224, -17.94116814877132526, -8.314950645356326220 ) ) ;
#12681=CARTESIAN_POINT ( 'NONE',  ( 2.121784821875004390, -19.68534013045801956, -10.23933436939529606 ) ) ;
#12684=ORIENTED_EDGE ( 'NONE', *, *, #207, .T. ) ;
#12685=CARTESIAN_POINT ( 'NONE',  ( -5.279047395330986450E-15, -28.02253625933941095, -7.686213421056266704 ) ) ;
#12686=DIRECTION ( 'NONE',  ( -0.000000000000000000, -0.5735764363510414965, -0.8191520442889950182 ) ) ;
#12691=CARTESIAN_POINT ( 'NONE',  ( -5.279047395330986450E-15, -30.60363022291909729, -11.37239762035674495 ) ) ;
#12695=CARTESIAN_POINT ( 'NONE',  ( 4.000000000000003553, -21.42239241568861274, -10.33918486777069745 ) ) ;
#12697=CARTESIAN_POINT ( 'NONE',  ( 4.000000000000003553, -18.90582580190336515, -6.745155274459496475 ) ) ;
#12699=CARTESIAN_POINT ( 'NONE',  ( -6.804503976930308617, -11.93919774785484300, 12.87494948068499134 ) ) ;
#12701=CARTESIAN_POINT ( 'NONE',  ( 4.243569643749997233, -25.50929166616339927, -7.878073867372210159 ) ) ;
#12704=CARTESIAN_POINT ( 'NONE',  ( -5.577813053751546416E-15, -23.12778347219005681, -1.774630616266089866 ) ) ;
#12706=CARTESIAN_POINT ( 'NONE',  ( -1.071796769724496334, -20.04751726799184297, -11.32312894147414539 ) ) ;
#12707=VERTEX_POINT ( 'NONE', #5571 ) ;
#12708=ORIENTED_EDGE ( 'NONE', *, *, #8300, .T. ) ;
#12710=CARTESIAN_POINT ( 'NONE',  ( 3.579096709490575479E-14, -23.06325612239561451, -1.682476010276811040 ) ) ;
#12711=EDGE_CURVE ( 'NONE', #8864, #17673, #16908, .T. ) ;
#12713=CARTESIAN_POINT ( 'NONE',  ( 2.000000000000004441, -20.00331654984898577, -10.32569345209524414 ) ) ;
#12716=AXIS2_PLACEMENT_3D ( 'NONE', #6629, #12274, #5232 ) ;
#12717=ADVANCED_FACE ( 'NONE', ( #17002 ), #7351, .F. ) ;
#12718=CARTESIAN_POINT ( 'NONE',  ( 2.121784821874994176, -26.27616332058593684, -6.837535036242106123 ) ) ;
#12721=CIRCLE ( 'NONE', #9449, 2.000000000000001776 ) ;
#12727=CARTESIAN_POINT ( 'NONE',  ( -2.121784821874996396, -19.64232189773168358, -10.17789796607362618 ) ) ;
#12734=CARTESIAN_POINT ( 'NONE',  ( 2.121784821874994176, -24.21128814972218990, -3.888587676801722903 ) ) ;
#12736=DIRECTION ( 'NONE',  ( 0.000000000000000000, 0.8191520442889950182, -0.5735764363510414965 ) ) ;
#12737=ORIENTED_EDGE ( 'NONE', *, *, #8396, .T. ) ;
#12741=DIRECTION ( 'NONE',  ( 0.000000000000000000, 0.000000000000000000, -1.000000000000000000 ) ) ;
#12744=CARTESIAN_POINT ( 'NONE',  ( 4.243569643749997233, -21.92802379169658877, -2.763493290842798267 ) ) ;
#12745=AXIS2_PLACEMENT_3D ( 'NONE', #15700, #7154, #212 ) ;
#12748=CARTESIAN_POINT ( 'NONE',  ( -2.121784821875005722, -29.15838491324991466, -10.95377405879430910 ) ) ;
#12752=CARTESIAN_POINT ( 'NONE',  ( 4.243569643750003451, -22.74293267755752623, -12.47028401514436169 ) ) ;
#12754=CARTESIAN_POINT ( 'NONE',  ( -1.661723472263481630E-14, -20.51073541163217584, -11.98467301000088803 ) ) ;
#12755=CARTESIAN_POINT ( 'NONE',  ( 1.999999999999994449, -23.69972968376769273, -3.525764780161007472 ) ) ;
#12758=EDGE_LOOP ( 'NONE', ( #3376, #858, #455, #595 ) ) ;
#12759=CARTESIAN_POINT ( 'NONE',  ( 3.083285004801276763, -24.87914370749852822, -15.73138478113422778 ) ) ;
#12763=CARTESIAN_POINT ( 'NONE',  ( 2.121784821874994176, -26.82464578784662379, -7.620849178593458007 ) ) ;
#12767=CARTESIAN_POINT ( 'NONE',  ( 3.999999999999996447, 6.938893903907228378E-15, 0.000000000000000000 ) ) ;
#12770=CARTESIAN_POINT ( 'NONE',  ( 8.500000000000019540, 0.000000000000000000, 20.49999999999998934 ) ) ;
#12772=CARTESIAN_POINT ( 'NONE',  ( -1.999999999999996225, -23.25119311998180649, -14.96414190187491400 ) ) ;
#12773=CARTESIAN_POINT ( 'NONE',  ( -2.121784821875005722, -24.54467945335122536, -4.364719802544705374 ) ) ;
#12774=VERTEX_POINT ( 'NONE', #2626 ) ;
#12775=ORIENTED_EDGE ( 'NONE', *, *, #15610, .F. ) ;
#12777=FACE_OUTER_BOUND ( 'NONE', #7488, .T. ) ;
#12780=EDGE_CURVE ( 'NONE', #12103, #159, #18227, .T. ) ;
#12781=CARTESIAN_POINT ( 'NONE',  ( -4.000000000000004441, -27.72246025710361295, -11.28397838367063244 ) ) ;
#12785=CARTESIAN_POINT ( 'NONE',  ( -3.999999999999997335, -22.11068413930986054, -11.32216732091749556 ) ) ;
#12788=CARTESIAN_POINT ( 'NONE',  ( -8.500000000000005329, 10.00000000000000000, 22.50000000000000000 ) ) ;
#12791=CARTESIAN_POINT ( 'NONE',  ( -7.316869269719566304, -13.46470072737469081, 2.124349773241079653 ) ) ;
#12793=CARTESIAN_POINT ( 'NONE',  ( -2.121784821874996396, -20.12627701590287543, -10.86905750344246435 ) ) ;
#12795=CARTESIAN_POINT ( 'NONE',  ( -1.071796769724496334, -21.59617364613965762, -13.53483946105443003 ) ) ;
#12800=CARTESIAN_POINT ( 'NONE',  ( -6.428571428571424384, -11.73421655796351892, 14.25837509840160422 ) ) ;
#12802=DIRECTION ( 'NONE',  ( -0.000000000000000000, 1.000000000000000000, -0.000000000000000000 ) ) ;
#12806=CARTESIAN_POINT ( 'NONE',  ( -4.243569643750005227, -24.82099994254214437, -6.895091414225420934 ) ) ;
#12811=FACE_OUTER_BOUND ( 'NONE', #5956, .T. ) ;
#12812=CARTESIAN_POINT ( 'NONE',  ( -4.243569643749997233, -20.62428471578586553, -9.444541151551892000 ) ) ;
#12817=CARTESIAN_POINT ( 'NONE',  ( -6.428571428571426161, -14.26578344203648285, -2.827263138854404279 ) ) ;
#12820=CARTESIAN_POINT ( 'NONE',  ( -4.243569643750000786, -20.51258062284889760, -5.013521062237622949 ) ) ;
#12821=CARTESIAN_POINT ( 'NONE',  ( 0.000000000000000000, 5.977523610840987267, 32.81826849749789687 ) ) ;
#12824=CARTESIAN_POINT ( 'NONE',  ( 4.243569643750003451, -25.06591724477924288, -15.78784979451479309 ) ) ;
#12827=DIRECTION ( 'NONE',  ( -1.000000000000000000, 0.000000000000000000, -0.000000000000000000 ) ) ;
#12828=CARTESIAN_POINT ( 'NONE',  ( -2.465190328815646976E-33, -26.97786251599082519, -14.24690051095425858 ) ) ;
#12829=ORIENTED_EDGE ( 'NONE', *, *, #609, .F. ) ;
#12830=CARTESIAN_POINT ( 'NONE',  ( -4.243569643750004339, -22.53027904986517527, -3.623602937346249941 ) ) ;
#12832=CARTESIAN_POINT ( 'NONE',  ( 4.243569643750000786, -26.86852450816387972, -14.09074965301504534 ) ) ;
#12835=CARTESIAN_POINT ( 'NONE',  ( -2.121784821874996396, -22.19115218676662238, -13.81800486288284624 ) ) ;
#12838=CARTESIAN_POINT ( 'NONE',  ( -2.000000000000005773, -27.35627946550557255, -8.747859062503353655 ) ) ;
#12840=CARTESIAN_POINT ( 'NONE',  ( 2.121784821875004390, -21.97606102313498511, -13.51082284627447017 ) ) ;
#12842=CARTESIAN_POINT ( 'NONE',  ( 4.713407268011036227E-15, -16.45483816335116245, -7.271100070990128117 ) ) ;
#12846=DIRECTION ( 'NONE',  ( -0.000000000000000000, 1.000000000000000000, -0.000000000000000000 ) ) ;
#12850=CARTESIAN_POINT ( 'NONE',  ( -4.243569643749998122, -22.43105049029164277, -12.02487009106222615 ) ) ;
#12854=DIRECTION ( 'NONE',  ( 0.000000000000000000, 0.8191520442889952403, -0.5735764363510413855 ) ) ;
#12856=CARTESIAN_POINT ( 'NONE',  ( -5.577813053751546416E-15, -25.38624068961733826, -5.000041789647243107 ) ) ;
#12857=CARTESIAN_POINT ( 'NONE',  ( -1.071796769724496334, -29.07582628914216727, -10.26931610931310246 ) ) ;
#12858=CARTESIAN_POINT ( 'NONE',  ( -1.661723472263481630E-14, -20.25262601527420969, -11.61605459007084029 ) ) ;
#12859=CARTESIAN_POINT ( 'NONE',  ( 4.243569643750000786, -21.70633658100450702, -6.718381254414091508 ) ) ;
#12869=ORIENTED_EDGE ( 'NONE', *, *, #17223, .F. ) ;
#12872=CARTESIAN_POINT ( 'NONE',  ( -1.999999999999996225, -20.15388036368618074, -10.54072086271434117 ) ) ;
#12877=CARTESIAN_POINT ( 'NONE',  ( -9.890239780389581625, -9.933741096495946721, 2.532703114057662575 ) ) ;
#12878=CARTESIAN_POINT ( 'NONE',  ( 4.243569643749997233, -23.96063528801558462, -5.666363347791923744 ) ) ;
#12879=EDGE_CURVE ( 'NONE', #5337, #13588, #12974, .T. ) ;
#12881=EDGE_CURVE ( 'NONE', #12502, #18310, #16202, .T. ) ;
#12886=CARTESIAN_POINT ( 'NONE',  ( -3.999999999999997335, -21.33635595023595144, -10.21631206112735057 ) ) ;
#12891=DIRECTION ( 'NONE',  ( 0.000000000000000000, 0.8191520442889949072, -0.5735764363510414965 ) ) ;
#12892=CARTESIAN_POINT ( 'NONE',  ( 2.121784821874994176, -26.53427271694390299, -7.206153456172153859 ) ) ;
#12895=CYLINDRICAL_SURFACE ( 'NONE', #11706, 7.499999999999999112 ) ;
#12896=CARTESIAN_POINT ( 'NONE',  ( 4.000000000000003553, -25.29403336105814404, -15.86846116672141527 ) ) ;
#12898=CARTESIAN_POINT ( 'NONE',  ( -5.330712181944245322E-15, -26.30097046047931997, -4.737218247813111738 ) ) ;
#12900=FACE_OUTER_BOUND ( 'NONE', #15591, .T. ) ;
#12904=CARTESIAN_POINT ( 'NONE',  ( -2.121784821875005722, -23.73808758973257227, -3.212787240263307531 ) ) ;
#12907=VERTEX_POINT ( 'NONE', #15965 ) ;
#12910=CARTESIAN_POINT ( 'NONE',  ( 4.243569643750000786, -26.57815143726116602, -13.67605393059374208 ) ) ;
#12913=DIRECTION ( 'NONE',  ( 0.000000000000000000, 0.8191520442889952403, -0.5735764363510413855 ) ) ;
#12916=CARTESIAN_POINT ( 'NONE',  ( -4.243569643750000786, -20.02862550467770220, -4.322361524868783889 ) ) ;
#12918=CARTESIAN_POINT ( 'NONE',  ( 4.243569643749996345, -28.38075870064580286, -11.97895378909399078 ) ) ;
#12919=DIRECTION ( 'NONE',  ( 0.000000000000000000, 0.8191520442889952403, -0.5735764363510413855 ) ) ;
#12921=CARTESIAN_POINT ( 'NONE',  ( 2.121784821874994176, -28.59914788780765704, -10.15510081561253664 ) ) ;
#12922=DIRECTION ( 'NONE',  ( 0.000000000000000000, 0.8191520442889952403, -0.5735764363510413855 ) ) ;
#12923=CARTESIAN_POINT ( 'NONE',  ( -3.706921591972381904E-14, -17.99416879784692469, -8.390643416689682610 ) ) ;
#12924=CARTESIAN_POINT ( 'NONE',  ( 4.000000000000003553, -24.06801372906274139, -14.11752367306044853 ) ) ;
#12925=CARTESIAN_POINT ( 'NONE',  ( -5.330712181944245322E-15, -28.59169135315628907, -8.008706724692286727 ) ) ;
#12926=DIRECTION ( 'NONE',  ( 0.000000000000000000, 0.8191520442889952403, -0.5735764363510413855 ) ) ;
#12927=CARTESIAN_POINT ( 'NONE',  ( -1.999999999999996225, -17.89542314625890285, -7.315309689333185261 ) ) ;
#12931=CARTESIAN_POINT ( 'NONE',  ( 2.599319604203554679, -24.48737926485759431, -15.99075565718284153 ) ) ;
#12938=ORIENTED_EDGE ( 'NONE', *, *, #1516, .F. ) ;
#12939=CARTESIAN_POINT ( 'NONE',  ( -4.243569643750000786, -24.67459463912114259, -10.95749308360964136 ) ) ;
#12942=ORIENTED_EDGE ( 'NONE', *, *, #13924, .T. ) ;
#12945=CARTESIAN_POINT ( 'NONE',  ( 1.071796769724476128, -16.71514851677590485, -6.564013151695367476 ) ) ;
#12946=CARTESIAN_POINT ( 'NONE',  ( 2.121784821874994176, -29.14763035506834044, -10.93841495796388763 ) ) ;
#12947=CARTESIAN_POINT ( 'NONE',  ( 3.999999999999996447, 6.938893903907228378E-15, 0.000000000000000000 ) ) ;
#12949=FACE_OUTER_BOUND ( 'NONE', #3284, .T. ) ;
#12951=CARTESIAN_POINT ( 'NONE',  ( -5.577813053751546416E-15, -29.25788163498686245, -10.52931808859795559 ) ) ;
#12952=CARTESIAN_POINT ( 'NONE',  ( 4.243569643750000786, -21.44822718464654088, -6.349762834484042884 ) ) ;
#12953=ORIENTED_EDGE ( 'NONE', *, *, #18188, .F. ) ;
#12962=ORIENTED_EDGE ( 'NONE', *, *, #10973, .F. ) ;
#12966=CARTESIAN_POINT ( 'NONE',  ( -1.999999999999996225, -20.67009915640211659, -11.27795770257443841 ) ) ;
#12967=VERTEX_POINT ( 'NONE', #756 ) ;
#12970=CARTESIAN_POINT ( 'NONE',  ( -7.505322150676213333, -12.67849954855525496, 7.208879555002704720 ) ) ;
#12971=CARTESIAN_POINT ( 'NONE',  ( -2.121784821875005722, -23.99619698609053842, -3.581405660193354379 ) ) ;
#12974=LINE ( 'NONE', #17181, #5594 ) ;
#12977=EDGE_LOOP ( 'NONE', ( #13217, #2224, #5254, #4348 ) ) ;
#12979=LINE ( 'NONE', #17371, #405 ) ;
#12981=CARTESIAN_POINT ( 'NONE',  ( 3.999999999999996447, -22.99045465720753256, -4.525974018286417433 ) ) ;
#12982=CARTESIAN_POINT ( 'NONE',  ( 2.000000000000004441, -22.00366437091829397, -13.18248620554634698 ) ) ;
#12983=ORIENTED_EDGE ( 'NONE', *, *, #12044, .F. ) ;
#12985=CARTESIAN_POINT ( 'NONE',  ( -2.000000000000005773, -29.16304524001135334, -11.32818800201368781 ) ) ;
#12986=CARTESIAN_POINT ( 'NONE',  ( 2.121784821875004390, -20.16929524862920431, -10.93049390676413601 ) ) ;
#12988=( BOUNDED_CURVE ( )  B_SPLINE_CURVE ( 2, ( #8587, #8968, #1563, #7571, #14644, #11837, #7200, #12857, #164 ),
 .UNSPECIFIED., .F., .F. ) 
 B_SPLINE_CURVE_WITH_KNOTS ( ( 3, 2, 2, 2, 3 ),
 ( 0.1465517241379310498, 0.1494252873563218509, 0.1551724137931034531, 0.1609195402298850552, 0.1637931034482758563 ),
 .UNSPECIFIED. ) 
 CURVE ( )  GEOMETRIC_REPRESENTATION_ITEM ( )  RATIONAL_B_SPLINE_CURVE ( ( 0.9330127018922192983, 0.9330127018922196314, 1.000000000000000000, 0.8660254037844387076, 1.000000000000000000, 0.8660254037844387076, 1.000000000000000000, 0.9330127018922194093, 0.9330127018922194093 ) ) 
 REPRESENTATION_ITEM ( '' )  );
#12994=CARTESIAN_POINT ( 'NONE',  ( 4.243569643750000786, -23.25499295915232167, -8.930091773994377036 ) ) ;
#12997=CARTESIAN_POINT ( 'NONE',  ( -3.537103074283056703, -10.00000000000000178, -11.53856502750640978 ) ) ;
#12998=CARTESIAN_POINT ( 'NONE',  ( -1.071796769724496334, -23.91363836198279103, -2.896947710712150403 ) ) ;
#13001=CARTESIAN_POINT ( 'NONE',  ( -4.243569643750005227, -23.27234356439432972, -4.683380894645135406 ) ) ;
#13002=CARTESIAN_POINT ( 'NONE',  ( 4.000000000000000888, -24.69072647674599352, -10.98053173535865135 ) ) ;
#13007=CARTESIAN_POINT ( 'NONE',  ( -4.243569643749997233, -24.46366198661064573, -14.92774014801135074 ) ) ;
#13011=ADVANCED_FACE ( 'NONE', ( #12228 ), #14858, .F. ) ;
#13012=CARTESIAN_POINT ( 'NONE',  ( 8.511038526056729836, -10.00000000000000178, -5.033916384140447953 ) ) ;
#13013=VERTEX_POINT ( 'NONE', #9084 ) ;
#13014=CARTESIAN_POINT ( 'NONE',  ( 4.243569643750003451, -18.64544601037477278, -6.618466598754856101 ) ) ;
#13016=CARTESIAN_POINT ( 'NONE',  ( 2.121784821874994176, -29.92195854414224598, -12.04427021775403084 ) ) ;
#13017=VECTOR ( 'NONE', #7638, 1000.000000000000000 ) ;
#13018=CARTESIAN_POINT ( 'NONE',  ( 0.000000000000000000, 9.254131787996968228, 30.52396275209373044 ) ) ;
#13019=CARTESIAN_POINT ( 'NONE',  ( 2.121784821875004390, -21.97606102313498511, -13.51082284627447017 ) ) ;
#13023=CARTESIAN_POINT ( 'NONE',  ( -2.121784821875005722, -28.12594732781803941, -9.479300379074118155 ) ) ;
#13025=CARTESIAN_POINT ( 'NONE',  ( -4.000000000000004441, -22.04405353722830085, -3.174373145209581804 ) ) ;
#13027=EDGE_LOOP ( 'NONE', ( #1571, #8548, #15779, #13106 ) ) ;
#13035=CARTESIAN_POINT ( 'NONE',  ( -2.121784821875005722, -26.86766402057294556, -7.682285581915135886 ) ) ;
#13038=CARTESIAN_POINT ( 'NONE',  ( 1.071796769724476128, -18.19927754512928075, -8.683569065286379285 ) ) ;
#13040=CARTESIAN_POINT ( 'NONE',  ( 4.730628863548789710E-15, -21.49956243961515767, -14.96605739982588368 ) ) ;
#13044=EDGE_CURVE ( 'NONE', #3510, #13645, #3793, .T. ) ;
#13046=CARTESIAN_POINT ( 'NONE',  ( -4.243569643750005227, -23.30460723893907371, -4.729458197136391817 ) ) ;
#13047=ORIENTED_EDGE ( 'NONE', *, *, #6799, .F. ) ;
#13048=CARTESIAN_POINT ( 'NONE',  ( 1.999999999999994449, -23.89331173033122369, -3.802228594101777492 ) ) ;
#13050=CARTESIAN_POINT ( 'NONE',  ( -3.706921591972381904E-14, -19.73640722255826319, -10.87881775021074127 ) ) ;
#13052=EDGE_LOOP ( 'NONE', ( #10007, #17748, #8219, #7292 ) ) ;
#13053=CARTESIAN_POINT ( 'NONE',  ( -4.000000000000004441, -22.30216293358627055, -3.542991565139629984 ) ) ;
#13056=EDGE_CURVE ( 'NONE', #7716, #10740, #7407, .T. ) ;
#13060=ORIENTED_EDGE ( 'NONE', *, *, #10565, .T. ) ;
#13062=CARTESIAN_POINT ( 'NONE',  ( 1.999999999999994449, -25.18385871212106863, -5.645320693752015728 ) ) ;
#13066=CARTESIAN_POINT ( 'NONE',  ( 9.911039980157271501, -9.932630671411386558, 2.546919849226038313 ) ) ;
#13067=CARTESIAN_POINT ( 'NONE',  ( 4.243569643750000786, -21.15785411374382363, -5.935067112062737849 ) ) ;
#13078=CARTESIAN_POINT ( 'NONE',  ( 1.071796769724495224, -22.39355523665122405, -14.67361839015640967 ) ) ;
#13079=CARTESIAN_POINT ( 'NONE',  ( 4.243569643750003451, -19.12940112854596819, -7.309626136123695161 ) ) ;
#13085=CARTESIAN_POINT ( 'NONE',  ( 4.000000000000000888, -26.94918369417327142, -14.20594290873980192 ) ) ;
#13086=PRODUCT_DEFINITION_FORMATION_WITH_SPECIFIED_SOURCE ( 'ANY', '', #16425, .NOT_KNOWN. ) ;
#13087=CARTESIAN_POINT ( 'NONE',  ( -4.243569643750000786, -22.09350067554145625, -7.271308884309165776 ) ) ;
#13088=EDGE_CURVE ( 'NONE', #15568, #8704, #438, .T. ) ;
#13089=CARTESIAN_POINT ( 'NONE',  ( 0.000000000000000000, 9.254131787996968228, 30.52396275209373044 ) ) ;
#13094=ORIENTED_EDGE ( 'NONE', *, *, #14664, .T. ) ;
#13096=( BOUNDED_CURVE ( )  B_SPLINE_CURVE ( 2, ( #9870, #16582, #10907, #16767, #9509, #11260, #11081, #7085, #15463 ),
 .UNSPECIFIED., .F., .T. ) 
 B_SPLINE_CURVE_WITH_KNOTS ( ( 3, 2, 2, 2, 3 ),
 ( 0.6293103448275861878, 0.6321839080459770166, 0.6379310344827586743, 0.6436781609195402210, 0.6465517241379310498 ),
 .UNSPECIFIED. ) 
 CURVE ( )  GEOMETRIC_REPRESENTATION_ITEM ( )  RATIONAL_B_SPLINE_CURVE ( ( 0.9330127018922194093, 0.9330127018922194093, 1.000000000000000000, 0.8660254037844387076, 1.000000000000000000, 0.8660254037844387076, 1.000000000000000000, 0.9330127018922194093, 0.9330127018922194093 ) ) 
 REPRESENTATION_ITEM ( '' )  );
#13097=CARTESIAN_POINT ( 'NONE',  ( -4.243569643749997233, -17.75281768130346194, -5.343661229830111381 ) ) ;
#13102=CARTESIAN_POINT ( 'NONE',  ( 2.121784821875004390, -22.49227981585092095, -14.24805968613456564 ) ) ;
#13104=CARTESIAN_POINT ( 'NONE',  ( 4.898587196589413815E-16, 2.700915433685006750, 35.11257424290206330 ) ) ;
#13105=CARTESIAN_POINT ( 'NONE',  ( 2.649389826666416869, -10.00000000000053824, -4.175485738721015139 ) ) ;
#13106=ORIENTED_EDGE ( 'NONE', *, *, #1841, .T. ) ;
#13110=CARTESIAN_POINT ( 'NONE',  ( -2.121784821875005722, -29.70686738051060161, -11.73708820114566009 ) ) ;
#13111=EDGE_CURVE ( 'NONE', #15867, #9076, #9959, .T. ) ;
#13113=CARTESIAN_POINT ( 'NONE',  ( 4.243569643750003451, -23.77537026298940503, -13.94475769486455263 ) ) ;
#13119=CARTESIAN_POINT ( 'NONE',  ( 2.121784821874994176, -27.82481969873374794, -9.049245555822391651 ) ) ;
#13120=CARTESIAN_POINT ( 'NONE',  ( 1.071796769724495224, -18.52191429128169631, -9.144342091205695411 ) ) ;
#13121=CARTESIAN_POINT ( 'NONE',  ( -5.279047395330986450E-15, -23.63467652125394025, -1.419700282245455636 ) ) ;
#13126=CARTESIAN_POINT ( 'NONE',  ( 2.000000000000004441, -23.61684809886054381, -15.48635133111591067 ) ) ;
#13127=CARTESIAN_POINT ( 'NONE',  ( -5.000000000000001776, 0.000000000000000000, 5.000000000000000888 ) ) ;
#13130=CARTESIAN_POINT ( 'NONE',  ( -2.121784821874996396, -21.70719706859543408, -13.12684532551400629 ) ) ;
#13133=VECTOR ( 'NONE', #13384, 1000.000000000000000 ) ;
#13136=CARTESIAN_POINT ( 'NONE',  ( 4.243569643749996345, -27.60643051157189731, -10.87309852930384935 ) ) ;
#13140=CARTESIAN_POINT ( 'NONE',  ( -4.243569643750005227, -24.07893542801298281, -5.835313456926535025 ) ) ;
#13142=CARTESIAN_POINT ( 'NONE',  ( -4.000000000000000888, -24.81978117492496949, -11.16484094532367699 ) ) ;
#13154=CARTESIAN_POINT ( 'NONE',  ( 2.000000000000004441, -19.93878920005454347, -10.23353884610596509 ) ) ;
#13157=LINE ( 'NONE', #7589, #4122 ) ;
#13159=CARTESIAN_POINT ( 'NONE',  ( 4.000000000000003553, -23.48726758655235969, -13.28813222721107934 ) ) ;
#13160=CARTESIAN_POINT ( 'NONE',  ( 4.243569643749997233, -23.70252589165762203, -5.297744927861876896 ) ) ;
#13162=CARTESIAN_POINT ( 'NONE',  ( 4.000000000000003553, -18.06697026303501730, -5.547145408680076883 ) ) ;
#13165=DIRECTION ( 'NONE',  ( -0.000000000000000000, -0.5735764363510414965, -0.8191520442889950182 ) ) ;
#13167=CARTESIAN_POINT ( 'NONE',  ( -1.071796769724486786, -23.33841207085099612, -16.02301379457549757 ) ) ;
#13171=CARTESIAN_POINT ( 'NONE',  ( 2.121784821875004390, -17.84631068140748766, -7.612928127393706390 ) ) ;
#13176=CARTESIAN_POINT ( 'NONE',  ( 2.121784821875004390, -23.55698107582754730, -15.76861066834601210 ) ) ;
#13178=CARTESIAN_POINT ( 'NONE',  ( 4.000000000000000888, -26.43296490145733557, -13.46870606887970645 ) ) ;
#13179=CARTESIAN_POINT ( 'NONE',  ( 2.121784821875004390, -18.65290254502614431, -8.764860689675106897 ) ) ;
#13180=CARTESIAN_POINT ( 'NONE',  ( -6.938893903907228378E-15, 6.938893903907228378E-15, 30.00000000000000000 ) ) ;
#13185=ORIENTED_EDGE ( 'NONE', *, *, #1744, .T. ) ;
#13186=CARTESIAN_POINT ( 'NONE',  ( -4.243569643750005227, -21.72368718624651507, -2.471670375064849434 ) ) ;
#13190=DIRECTION ( 'NONE',  ( 0.000000000000000000, 0.000000000000000000, 1.000000000000000000 ) ) ;
#13191=CARTESIAN_POINT ( 'NONE',  ( 4.243569643750000786, -25.54571385182929077, -12.20158025087355114 ) ) ;
#13193=VECTOR ( 'NONE', #8271, 1000.000000000000000 ) ;
#13194=FACE_OUTER_BOUND ( 'NONE', #14252, .T. ) ;
#13196=CARTESIAN_POINT ( 'NONE',  ( 0.3267727178447701331, -10.00000000000000178, -5.052762561672880182 ) ) ;
#13199=CARTESIAN_POINT ( 'NONE',  ( -2.121784821874996396, -23.51396284310121487, -15.70717426502434044 ) ) ;
#13200=EDGE_CURVE ( 'NONE', #11449, #851, #6754, .T. ) ;
#13201=CARTESIAN_POINT ( 'NONE',  ( -5.330712181944246111E-15, -28.07547256044034967, -7.271469884832190367 ) ) ;
#13202=( BOUNDED_CURVE ( )  B_SPLINE_CURVE ( 2, ( #4070, #6853, #11468, #4340, #16891, #5823, #5646, #9987, #11289 ),
 .UNSPECIFIED., .F., .F. ) 
 B_SPLINE_CURVE_WITH_KNOTS ( ( 3, 2, 2, 2, 3 ),
 ( 0.1810344827586206906, 0.1839080459770114917, 0.1896551724137930939, 0.1954022988505747238, 0.1982758620689655249 ),
 .UNSPECIFIED. ) 
 CURVE ( )  GEOMETRIC_REPRESENTATION_ITEM ( )  RATIONAL_B_SPLINE_CURVE ( ( 0.9330127018922194093, 0.9330127018922194093, 1.000000000000000000, 0.8660254037844387076, 1.000000000000000000, 0.8660254037844387076, 1.000000000000000000, 0.9330127018922194093, 0.9330127018922194093 ) ) 
 REPRESENTATION_ITEM ( '' )  );
#13204=AXIS2_PLACEMENT_3D ( 'NONE', #14925, #17804, #5159 ) ;
#13205=CARTESIAN_POINT ( 'NONE',  ( 2.121784821874994176, -25.75994452787000100, -6.100298196382009763 ) ) ;
#13207=DIRECTION ( 'NONE',  ( 1.049727191973305394E-16, 0.5150380737757255245, -0.8571673013836856869 ) ) ;
#13209=DIRECTION ( 'NONE',  ( -0.000000000000000000, -0.5735764363510414965, -0.8191520442889950182 ) ) ;
#13211=CARTESIAN_POINT ( 'NONE',  ( 1.999999999999994449, -26.79704244006331493, -7.949185819321580304 ) ) ;
#13213=CARTESIAN_POINT ( 'NONE',  ( -1.999999999999996225, -22.54139228070233614, -13.95044124807404451 ) ) ;
#13214=FACE_OUTER_BOUND ( 'NONE', #16497, .T. ) ;
#13217=ORIENTED_EDGE ( 'NONE', *, *, #13512, .F. ) ;
#13218=CARTESIAN_POINT ( 'NONE',  ( -4.243569643750000786, -23.12593826097332794, -8.745782564029356720 ) ) ;
#13220=CIRCLE ( 'NONE', #11747, 4.000000000000000000 ) ;
#13225=CARTESIAN_POINT ( 'NONE',  ( -4.243569643750005227, -28.20868576974048025, -11.73320817580729880 ) ) ;
#13228=CARTESIAN_POINT ( 'NONE',  ( -4.000000000000004441, -26.88360471823526865, -10.08596851789121018 ) ) ;
#13229=CARTESIAN_POINT ( 'NONE',  ( -2.121784821874996396, -17.31933733050996338, -6.860332186703194779 ) ) ;
#13230=VERTEX_POINT ( 'NONE', #2604 ) ;
#13231=CARTESIAN_POINT ( 'NONE',  ( -8.999999999999996447, -10.00000000000000000, -3.713574246709372417 ) ) ;
#13232=CARTESIAN_POINT ( 'NONE',  ( -1.999999999999996225, -20.21840771348061949, -10.63287546870361666 ) ) ;
#13238=FACE_OUTER_BOUND ( 'NONE', #11452, .T. ) ;
#13243=ORIENTED_EDGE ( 'NONE', *, *, #15905, .F. ) ;
#13246=CARTESIAN_POINT ( 'NONE',  ( 2.000000000000004441, -19.16446101098063792, -9.127683586315821884 ) ) ;
#13251=CARTESIAN_POINT ( 'NONE',  ( 3.999999999999996447, -25.76513066735074986, -8.488622031527665257 ) ) ;
#13252=CARTESIAN_POINT ( 'NONE',  ( 2.121784821874994176, -23.95317875336422020, -3.519969256871676055 ) ) ;
#13255=CARTESIAN_POINT ( 'NONE',  ( -1.071796769724496334, -26.17209557941007603, -6.122358884093301867 ) ) ;
#13257=CARTESIAN_POINT ( 'NONE',  ( -1.287074048710188379, -10.56983422227299130, 22.11683441173179077 ) ) ;
#13262=EDGE_LOOP ( 'NONE', ( #2287, #17703, #15866 ) ) ;
#13263=VECTOR ( 'NONE', #13378, 1000.000000000000000 ) ;
#13267=CARTESIAN_POINT ( 'NONE',  ( 4.243569643750000786, -21.41596351010179333, -6.303685531992786473 ) ) ;
#13270=CARTESIAN_POINT ( 'NONE',  ( -5.330712181944246111E-15, -30.43072080220681741, -10.63511296669387818 ) ) ;
#13271=CARTESIAN_POINT ( 'NONE',  ( -3.999999999999997335, -24.17555931017360393, -14.27111468035787745 ) ) ;
#13273=CARTESIAN_POINT ( 'NONE',  ( -4.243569643750005227, -23.82082603165501666, -5.466695036996486401 ) ) ;
#13274=CARTESIAN_POINT ( 'NONE',  ( -6.774459155162589674, -14.04910063648303264, -1.424143818374616233 ) ) ;
#13277=LINE ( 'NONE', #7985, #9385 ) ;
#13282=ORIENTED_EDGE ( 'NONE', *, *, #8679, .F. ) ;
#13283=ORIENTED_EDGE ( 'NONE', *, *, #1672, .F. ) ;
#13286=CARTESIAN_POINT ( 'NONE',  ( -5.577813053751546416E-15, -24.09569370782749331, -3.156949689997003539 ) ) ;
#13289=VERTEX_POINT ( 'NONE', #15401 ) ;
#13291=CARTESIAN_POINT ( 'NONE',  ( 4.730628863548789710E-15, -21.98351755778634953, -15.65721693719472185 ) ) ;
#13296=CARTESIAN_POINT ( 'NONE',  ( -2.000000000000005773, -26.77553332299520150, -7.918467616653980024 ) ) ;
#13297=CARTESIAN_POINT ( 'NONE',  ( 2.121784821875004390, -21.75021530132177006, -13.18828172883567973 ) ) ;
#13300=CIRCLE ( 'NONE', #5611, 2.000000000000001776 ) ;
#13301=CARTESIAN_POINT ( 'NONE',  ( 4.243569643750003451, -22.22671388484159039, -11.73304717528426622 ) ) ;
#13302=DIRECTION ( 'NONE',  ( -1.000000000000000000, 0.000000000000000000, 0.000000000000000000 ) ) ;
#13304=CARTESIAN_POINT ( 'NONE',  ( -4.000000000000000888, -26.30391020327834539, -13.28439685891468613 ) ) ;
#13305=CARTESIAN_POINT ( 'NONE',  ( 4.243569643750000786, -27.09437022997710187, -14.41329077045383578 ) ) ;
#13306=CARTESIAN_POINT ( 'NONE',  ( 2.121784821875004390, -20.94362343770310986, -12.03634916655427922 ) ) ;
#13310=ORIENTED_EDGE ( 'NONE', *, *, #7729, .T. ) ;
#13312=CYLINDRICAL_SURFACE ( 'NONE', #8646, 4.000000000000000000 ) ;
#13317=CARTESIAN_POINT ( 'NONE',  ( 4.243569643749997233, -24.50911775527627157, -6.449677490143276515 ) ) ;
#13320=CIRCLE ( 'NONE', #1198, 2.999999999999999112 ) ;
#13321=( BOUNDED_CURVE ( )  B_SPLINE_CURVE ( 2, ( #4529, #8880, #14746, #11749, #1856, #4712, #16137, #7489, #17542 ),
 .UNSPECIFIED., .F., .F. ) 
 B_SPLINE_CURVE_WITH_KNOTS ( ( 3, 2, 2, 2, 3 ),
 ( 0.3706896551724138122, 0.3735632183908045856, 0.3793103448275861878, 0.3850574712643677899, 0.3879310344827586188 ),
 .UNSPECIFIED. ) 
 CURVE ( )  GEOMETRIC_REPRESENTATION_ITEM ( )  RATIONAL_B_SPLINE_CURVE ( ( 0.9330127018922194093, 0.9330127018922200755, 1.000000000000000000, 0.8660254037844387076, 1.000000000000000000, 0.8660254037844387076, 1.000000000000000000, 0.9330127018922194093, 0.9330127018922194093 ) ) 
 REPRESENTATION_ITEM ( '' )  );
#13323=DIRECTION ( 'NONE',  ( -0.000000000000000000, -0.000000000000000000, -1.000000000000000000 ) ) ;
#13325=CARTESIAN_POINT ( 'NONE',  ( -4.243569643749997233, -23.72159747208149128, -13.86796219071246306 ) ) ;
#13326=FACE_OUTER_BOUND ( 'NONE', #1994, .T. ) ;
#13328=CARTESIAN_POINT ( 'NONE',  ( 4.898587196589413815E-16, 2.700915433685006750, 35.11257424290206330 ) ) ;
#13329=CARTESIAN_POINT ( 'NONE',  ( 2.121784821874994176, -29.88969486959749844, -11.99819291526277532 ) ) ;
#13331=CARTESIAN_POINT ( 'NONE',  ( 4.898587196589409870E-16, 4.000000000000007105, -4.000000000000000000 ) ) ;
#13332=CARTESIAN_POINT ( 'NONE',  ( -2.000000000000005773, -25.80762308735776145, -6.536148542923068128 ) ) ;
#13334=CARTESIAN_POINT ( 'NONE',  ( 4.898587196589413815E-16, 2.700915433685006750, 35.11257424290206330 ) ) ;
#13336=VERTEX_POINT ( 'NONE', #5550 ) ;
#13338=LINE ( 'NONE', #271, #8953 ) ;
#13341=CARTESIAN_POINT ( 'NONE',  ( 4.299564228933482956E-15, -21.02695420434810814, -12.72190984986098172 ) ) ;
#13343=ORIENTED_EDGE ( 'NONE', *, *, #5157, .F. ) ;
#13345=CARTESIAN_POINT ( 'NONE',  ( -1.999999999999996225, -19.37955217461227875, -9.434865602924197958 ) ) ;
#13348=CARTESIAN_POINT ( 'NONE',  ( 4.400000000000002132, -26.97786251599087137, -14.24690051095422660 ) ) ;
#13351=CARTESIAN_POINT ( 'NONE',  ( -2.121784821875005722, -22.96375940065866672, -2.106931980473163879 ) ) ;
#13352=CARTESIAN_POINT ( 'NONE',  ( 4.243569643750003451, -21.48464937031242883, -10.67326921798538386 ) ) ;
#13353=ADVANCED_FACE ( 'NONE', ( #17156 ), #4430, .F. ) ;
#13354=EDGE_LOOP ( 'NONE', ( #14770, #13283 ) ) ;
#13355=CARTESIAN_POINT ( 'NONE',  ( -5.954418220269360518, -10.00000000000000178, 20.87519200589466095 ) ) ;
#13358=CARTESIAN_POINT ( 'NONE',  ( -2.121784821874996396, -23.77207223945918457, -16.07579268495438996 ) ) ;
#13362=CARTESIAN_POINT ( 'NONE',  ( -4.243569643750000786, -21.02879941556483345, -5.750757902097718421 ) ) ;
#13365=CARTESIAN_POINT ( 'NONE',  ( -4.243569643750000786, -26.48136041362692339, -13.53782202311997551 ) ) ;
#13366=CARTESIAN_POINT ( 'NONE',  ( 2.000000000000004441, -23.03610195635016922, -14.65695988526653792 ) ) ;
#13367=CARTESIAN_POINT ( 'NONE',  ( -2.121784821874996396, -18.60988431229980833, -8.703424286353433459 ) ) ;
#13378=DIRECTION ( 'NONE',  ( 0.000000000000000000, -0.5735764363510413855, -0.8191520442889951292 ) ) ;
#13379=EDGE_LOOP ( 'NONE', ( #16196, #5698 ) ) ;
#13382=CARTESIAN_POINT ( 'NONE',  ( -2.121784821875005722, -28.64216612053397526, -10.21653721893421363 ) ) ;
#13384=DIRECTION ( 'NONE',  ( -0.000000000000000000, -0.5735764363510414965, -0.8191520442889950182 ) ) ;
#13385=CARTESIAN_POINT ( 'NONE',  ( -0.8866433558321317188, -10.00000000000235545, -3.510284692361743897 ) ) ;
#13387=CARTESIAN_POINT ( 'NONE',  ( 4.243569643749996345, -27.86453990792986701, -11.24171694923389531 ) ) ;
#13389=CARTESIAN_POINT ( 'NONE',  ( -1.071796769724486786, -21.01542750362927592, -12.70544801520506972 ) ) ;
#13390=CARTESIAN_POINT ( 'NONE',  ( 4.243569643750003451, -22.74293267755752623, -12.47028401514436347 ) ) ;
#13395=CARTESIAN_POINT ( 'NONE',  ( 4.730628863548789710E-15, -19.40242359420666318, -11.97103273789424449 ) ) ;
#13406=CARTESIAN_POINT ( 'NONE',  ( -1.661723472263481630E-14, -21.09148155414255044, -12.81406445585025544 ) ) ;
#13408=ORIENTED_EDGE ( 'NONE', *, *, #7443, .T. ) ;
#13409=CARTESIAN_POINT ( 'NONE',  ( -4.243569643749998122, -20.62428471578586553, -9.444541151551893776 ) ) ;
#13411=EDGE_CURVE ( 'NONE', #14057, #15568, #9306, .T. ) ;
#13412=ORIENTED_EDGE ( 'NONE', *, *, #3031, .T. ) ;
#13417=CARTESIAN_POINT ( 'NONE',  ( 7.402533184386031806, -12.48645682432232284, 8.629691327595670813 ) ) ;
#13420=CARTESIAN_POINT ( 'NONE',  ( -2.121784821874996396, -17.57744672686793308, -7.228950606633243403 ) ) ;
#13423=CARTESIAN_POINT ( 'NONE',  ( 4.000000000000000888, -23.14207009859818243, -8.768821215778363154 ) ) ;
#13424=ORIENTED_EDGE ( 'NONE', *, *, #1627, .F. ) ;
#13425=EDGE_LOOP ( 'NONE', ( #13602, #11954, #10916, #15181 ) ) ;
#13435=CARTESIAN_POINT ( 'NONE',  ( 3.999999999999996447, -23.44214610012902966, -5.171056252157234745 ) ) ;
#13440=CARTESIAN_POINT ( 'NONE',  ( -4.243569643750000786, -20.25447122649092790, -4.644902642307576102 ) ) ;
#13441=CARTESIAN_POINT ( 'NONE',  ( -5.330712181944245322E-15, -28.36584563134306691, -7.686165607253494514 ) ) ;
#13442=CARTESIAN_POINT ( 'NONE',  ( -5.577813053751546416E-15, -26.16056887869124381, -6.105897049437384538 ) ) ;
#13443=VERTEX_POINT ( 'NONE', #11374 ) ;
#13444=CARTESIAN_POINT ( 'NONE',  ( -0.7594769011887880783, -10.00000000000000178, 23.07585096715833473 ) ) ;
#13445=DIRECTION ( 'NONE',  ( -0.000000000000000000, -0.5735764363510414965, -0.8191520442889950182 ) ) ;
#13447=CARTESIAN_POINT ( 'NONE',  ( 2.121784821874994176, -29.40573975142631014, -11.30703337789393359 ) ) ;
#13448=VERTEX_POINT ( 'NONE', #14554 ) ;
#13450=EDGE_CURVE ( 'NONE', #12141, #15771, #17063, .T. ) ;
#13453=CARTESIAN_POINT ( 'NONE',  ( 2.121784821874994176, -24.72750694243812219, -4.625824516661818819 ) ) ;
#13456=CARTESIAN_POINT ( 'NONE',  ( -4.243569643749998122, -23.97970686843945742, -14.23658061064251257 ) ) ;
#13457=CARTESIAN_POINT ( 'NONE',  ( 1.999999999999994449, -29.05549965749059638, -11.17459699270273354 ) ) ;
#13459=CARTESIAN_POINT ( 'NONE',  ( -2.121784821875005722, -24.02846066063528596, -3.627482962684610346 ) ) ;
#13462=CARTESIAN_POINT ( 'NONE',  ( -2.000000000000005773, -28.32418970114301260, -10.13017813623426733 ) ) ;
#13463=CARTESIAN_POINT ( 'NONE',  ( 2.000000000000004441, -17.35769523647485713, -6.547354646805487732 ) ) ;
#13464=DIRECTION ( 'NONE',  ( 0.000000000000000000, 0.8191520442889952403, -0.5735764363510413855 ) ) ;
#13465=ORIENTED_EDGE ( 'NONE', *, *, #12044, .T. ) ;
#13469=CARTESIAN_POINT ( 'NONE',  ( 1.071796769724485232, -29.24635493426803379, -10.51285625394204182 ) ) ;
#13470=ORIENTED_EDGE ( 'NONE', *, *, #15904, .T. ) ;
#13472=CARTESIAN_POINT ( 'NONE',  ( -4.243569643750000786, -25.41665915365029704, -12.01727104090852905 ) ) ;
#13475=CARTESIAN_POINT ( 'NONE',  ( -3.999999999999997335, -22.11068413930986054, -11.32216732091749556 ) ) ;
#13476=CARTESIAN_POINT ( 'NONE',  ( 4.243569643750000786, -25.83608692273200802, -12.61627597329485440 ) ) ;
#13479=CARTESIAN_POINT ( 'NONE',  ( -3.999999999999997335, -24.43366870653157363, -14.63973310028792518 ) ) ;
#13481=CARTESIAN_POINT ( 'NONE',  ( -4.243569643749997233, -21.88256802303096293, -11.24155594871087338 ) ) ;
#13482=VERTEX_POINT ( 'NONE', #11558 ) ;
#13490=DIRECTION ( 'NONE',  ( -0.3258630558627223506, -2.733395053862362198E-16, -0.9454169814551716122 ) ) ;
#13492=CARTESIAN_POINT ( 'NONE',  ( -2.121784821874996396, -19.12610310501574418, -9.440661126213528931 ) ) ;
#13495=VECTOR ( 'NONE', #9664, 1000.000000000000000 ) ;
#13496=DIRECTION ( 'NONE',  ( 0.000000000000000000, 0.000000000000000000, 1.000000000000000000 ) ) ;
#13499=CARTESIAN_POINT ( 'NONE',  ( -2.511069452714361550, -24.47646004445711299, -16.25126521642124189 ) ) ;
#13502=CARTESIAN_POINT ( 'NONE',  ( 4.243569643750003451, -18.38733661401680308, -6.249848178824808365 ) ) ;
#13506=CARTESIAN_POINT ( 'NONE',  ( -4.000000000000000888, -22.49679660770325285, -7.847275165953248255 ) ) ;
#13509=EDGE_LOOP ( 'NONE', ( #8777, #12, #15510, #2634 ) ) ;
#13510=ORIENTED_EDGE ( 'NONE', *, *, #8996, .T. ) ;
#13511=CARTESIAN_POINT ( 'NONE',  ( 0.000000000000000000, 10.00000000000000000, 4.000000000000000000 ) ) ;
#13512=EDGE_CURVE ( 'NONE', #6584, #17470, #11745, .T. ) ;
#13520=CARTESIAN_POINT ( 'NONE',  ( -2.000000000000005773, -23.67822056669957576, -3.495046577493408968 ) ) ;
#13526=VECTOR ( 'NONE', #16263, 1000.000000000000000 ) ;
#13527=CARTESIAN_POINT ( 'NONE',  ( -4.243569643749997233, -22.17294109393367307, -11.65625167113217664 ) ) ;
#13529=CARTESIAN_POINT ( 'NONE',  ( 1.342650718860975534, -30.09701863977672431, -12.10727608660696752 ) ) ;
#13531=CARTESIAN_POINT ( 'NONE',  ( -3.999999999999997335, -17.98093379758235955, -5.424272602036731783 ) ) ;
#13533=CARTESIAN_POINT ( 'NONE',  ( 2.121784821875004390, -23.55698107582754730, -15.76861066834601210 ) ) ;
#13537=CARTESIAN_POINT ( 'NONE',  ( -2.121784821874996396, -17.54518305232318554, -7.182873304141986992 ) ) ;
#13539=AXIS2_PLACEMENT_3D ( 'NONE', #11047, #9831, #18217 ) ;
#13542=CARTESIAN_POINT ( 'NONE',  ( 4.000000000000003553, -23.74537698291033294, -13.65675064714112885 ) ) ;
#13544=CARTESIAN_POINT ( 'NONE',  ( 2.121784821875004390, -18.39479314866817461, -8.396242269745057385 ) ) ;
#13547=CIRCLE ( 'NONE', #7321, 2.000000000000001776 ) ;
#13550=AXIS2_PLACEMENT_3D ( 'NONE', #2739, #8452, #4116 ) ;
#13551=VERTEX_POINT ( 'NONE', #10456 ) ;
#13554=CYLINDRICAL_SURFACE ( 'NONE', #9121, 4.000000000000000000 ) ;
#13557=DIRECTION ( 'NONE',  ( 0.000000000000000000, 0.000000000000000000, 1.000000000000000000 ) ) ;
#13558=CARTESIAN_POINT ( 'NONE',  ( -2.121784821874996396, -21.15871460133474713, -12.34353118316265707 ) ) ;
#13561=CARTESIAN_POINT ( 'NONE',  ( 0.000000000000000000, 9.254131787996968228, 30.52396275209373044 ) ) ;
#13562=CARTESIAN_POINT ( 'NONE',  ( -1.071796769724486564, -27.20453316484195483, -7.596832563813487482 ) ) ;
#13564=CARTESIAN_POINT ( 'NONE',  ( -4.243569643750000786, -25.96514162091098399, -12.80058518325988182 ) ) ;
#13566=CARTESIAN_POINT ( 'NONE',  ( 4.074955379826664448, -26.45924826029166965, -14.98212748481132905 ) ) ;
#13569=CARTESIAN_POINT ( 'NONE',  ( 2.121784821875004390, -20.68551404134514016, -11.66773074662423149 ) ) ;
#13571=CARTESIAN_POINT ( 'NONE',  ( 0.000000000000000000, 5.977523610840987267, 32.81826849749789687 ) ) ;
#13583=( BOUNDED_CURVE ( )  B_SPLINE_CURVE ( 2, ( #12202, #9331, #5068, #10909, #9420, #15279, #3954, #4980, #8031 ),
 .UNSPECIFIED., .F., .T. ) 
 B_SPLINE_CURVE_WITH_KNOTS ( ( 3, 2, 2, 2, 3 ),
 ( 0.8362068965517241992, 0.8390804597701149170, 0.8448275862068965747, 0.8505747126436781214, 0.8534482758620689502 ),
 .UNSPECIFIED. ) 
 CURVE ( )  GEOMETRIC_REPRESENTATION_ITEM ( )  RATIONAL_B_SPLINE_CURVE ( ( 0.9330127018922194093, 0.9330127018922206306, 1.000000000000000000, 0.8660254037844387076, 1.000000000000000000, 0.8660254037844387076, 1.000000000000000000, 0.9330127018922194093, 0.9330127018922194093 ) ) 
 REPRESENTATION_ITEM ( '' )  );
#13584=ORIENTED_EDGE ( 'NONE', *, *, #7337, .F. ) ;
#13585=CARTESIAN_POINT ( 'NONE',  ( -5.330712181944246111E-15, -26.81718925319525937, -5.474455087673208986 ) ) ;
#13588=VERTEX_POINT ( 'NONE', #17873 ) ;
#13594=CARTESIAN_POINT ( 'NONE',  ( 4.551717183842061587, -10.00000000000000178, -2.180355508048899882 ) ) ;
#13595=CARTESIAN_POINT ( 'NONE',  ( 1.071796769724494780, -27.95580795247818173, -8.669764154291803138 ) ) ;
#13596=CARTESIAN_POINT ( 'NONE',  ( -4.243569643750005227, -28.95075028426964181, -12.79298613310618471 ) ) ;
#13599=CARTESIAN_POINT ( 'NONE',  ( 3.999999999999996447, -25.57154862078722246, -8.212158217586894793 ) ) ;
#13602=ORIENTED_EDGE ( 'NONE', *, *, #9430, .F. ) ;
#13603=ORIENTED_EDGE ( 'NONE', *, *, #2647, .T. ) ;
#13604=CARTESIAN_POINT ( 'NONE',  ( 4.000000000000003553, -20.45448218005117624, -8.956865794039783779 ) ) ;
#13605=AXIS2_PLACEMENT_3D ( 'NONE', #10067, #5995, #10255 ) ;
#13609=ORIENTED_EDGE ( 'NONE', *, *, #10968, .F. ) ;
#13611=CARTESIAN_POINT ( 'NONE',  ( 4.000000000000003553, -19.35751724482486580, -7.390237508330316452 ) ) ;
#13613=EDGE_CURVE ( 'NONE', #15568, #14065, #12275, .T. ) ;
#13614=CARTESIAN_POINT ( 'NONE',  ( -3.999999999999997335, -19.78769957208813679, -8.004601541547065935 ) ) ;
#13617=CARTESIAN_POINT ( 'NONE',  ( 4.299564228933482956E-15, -17.41342265533655009, -7.561251970840314307 ) ) ;
#13620=CARTESIAN_POINT ( 'NONE',  ( -2.121784821874996396, -20.93286887952152497, -12.02099006572386486 ) ) ;
#13622=CARTESIAN_POINT ( 'NONE',  ( -4.000000000000004441, -24.81872954737152170, -7.137021158450828295 ) ) ;
#13624=CYLINDRICAL_SURFACE ( 'NONE', #16357, 4.000000000000000000 ) ;
#13626=CARTESIAN_POINT ( 'NONE',  ( -4.000000000000004441, -24.56062015101355911, -6.768402738520781448 ) ) ;
#13627=CARTESIAN_POINT ( 'NONE',  ( -1.071796769724496334, -25.97851353284654152, -5.845895070152532291 ) ) ;
#13631=CARTESIAN_POINT ( 'NONE',  ( -4.243569643750000786, -20.25447122649092790, -4.644902642307576102 ) ) ;
#13635=CARTESIAN_POINT ( 'NONE',  ( 3.999999999999996447, -27.31378704549856096, -10.70033255110795167 ) ) ;
#13637=CARTESIAN_POINT ( 'NONE',  ( -4.243569643750000786, -20.02862550467770220, -4.322361524868783889 ) ) ;
#13640=CARTESIAN_POINT ( 'NONE',  ( -1.071796769724491671, -22.30597448541912087, -14.54854011485530840 ) ) ;
#13642=CARTESIAN_POINT ( 'NONE',  ( 1.999999999999994449, -27.24873388298481558, -8.594268053192397616 ) ) ;
#13644=ORIENTED_EDGE ( 'NONE', *, *, #12780, .T. ) ;
#13645=VERTEX_POINT ( 'NONE', #8195 ) ;
#13648=CARTESIAN_POINT ( 'NONE',  ( 7.491798610157291982, -13.11847650086634509, 4.256480280831525853 ) ) ;
#13651=CARTESIAN_POINT ( 'NONE',  ( -5.330712181944245322E-15, -28.33358195679831937, -7.640088304762238103 ) ) ;
#13656=CARTESIAN_POINT ( 'NONE',  ( -2.343145750507620750, 4.000000000000007994, -4.000000000000000888 ) ) ;
#13658=CARTESIAN_POINT ( 'NONE',  ( -2.121784821874996396, -21.96530646495340378, -13.49546374544405403 ) ) ;
#13662=CARTESIAN_POINT ( 'NONE',  ( 4.898587196589413815E-16, 2.700915433685006750, 35.11257424290206330 ) ) ;
#13663=CARTESIAN_POINT ( 'NONE',  ( 2.121784821874994176, -25.50183513151203130, -5.731679776451962915 ) ) ;
#13664=CARTESIAN_POINT ( 'NONE',  ( -3.999999999999997335, -20.11033631824054524, -8.465374567466390943 ) ) ;
#13675=CARTESIAN_POINT ( 'NONE',  ( -2.121784821875005722, -24.28657005699325921, -3.996101382614658970 ) ) ;
#13678=AXIS2_PLACEMENT_3D ( 'NONE', #11137, #16823, #5120 ) ;
#13679=ORIENTED_EDGE ( 'NONE', *, *, #12711, .F. ) ;
#13680=ADVANCED_FACE ( 'NONE', ( #2381 ), #836, .T. ) ;
#13681=VERTEX_POINT ( 'NONE', #3383 ) ;
#13682=CARTESIAN_POINT ( 'NONE',  ( 4.000000000000003553, -19.87373603754079809, -8.127474348190411035 ) ) ;
#13683=EDGE_CURVE ( 'NONE', #11829, #17908, #14742, .T. ) ;
#13684=FACE_OUTER_BOUND ( 'NONE', #17166, .T. ) ;
#13685=CARTESIAN_POINT ( 'NONE',  ( 2.658838382460517735, -24.55987625702158539, -16.27480033055179476 ) ) ;
#13686=CARTESIAN_POINT ( 'NONE',  ( 7.638598542356191956, -10.30911785226841282, 7.201745306969625560 ) ) ;
#13687=EDGE_CURVE ( 'NONE', #17470, #1591, #3637, .T. ) ;
#13689=CARTESIAN_POINT ( 'NONE',  ( -4.243569643750000786, -25.67476855000827030, -12.38588946083857856 ) ) ;
#13693=CARTESIAN_POINT ( 'NONE',  ( 2.000000000000004441, -19.22898836077508022, -9.219838192305099156 ) ) ;
#13696=ORIENTED_EDGE ( 'NONE', *, *, #2090, .F. ) ;
#13698=( BOUNDED_CURVE ( )  B_SPLINE_CURVE ( 2, ( #9852, #1069, #15261, #2557, #8189, #9668, #10304, #12998, #11413 ),
 .UNSPECIFIED., .F., .T. ) 
 B_SPLINE_CURVE_WITH_KNOTS ( ( 3, 2, 2, 2, 3 ),
 ( 0.8362068965517241992, 0.8390804597701149170, 0.8448275862068965747, 0.8505747126436781214, 0.8534482758620689502 ),
 .UNSPECIFIED. ) 
 CURVE ( )  GEOMETRIC_REPRESENTATION_ITEM ( )  RATIONAL_B_SPLINE_CURVE ( ( 0.9330127018922194093, 0.9330127018922206306, 1.000000000000000000, 0.8660254037844387076, 1.000000000000000000, 0.8660254037844387076, 1.000000000000000000, 0.9330127018922194093, 0.9330127018922194093 ) ) 
 REPRESENTATION_ITEM ( '' )  );
#13699=CARTESIAN_POINT ( 'NONE',  ( 3.999999999999996447, -27.37831439529299615, -10.79248715709722717 ) ) ;
#13706=CARTESIAN_POINT ( 'NONE',  ( 2.000000000000004441, -18.13202342554876267, -7.653209906595630940 ) ) ;
#13712=LINE ( 'NONE', #6664, #16178 ) ;
#13713=CARTESIAN_POINT ( 'NONE',  ( -5.330712181944246111E-15, -24.72005040778675777, -2.479430425741570243 ) ) ;
#13714=CARTESIAN_POINT ( 'NONE',  ( 4.730628863548789710E-15, -20.46712485418328242, -13.49158372010569273 ) ) ;
#13724=CARTESIAN_POINT ( 'NONE',  ( -4.243569643750000786, -19.73825243377498850, -3.907665802447479297 ) ) ;
#13728=( BOUNDED_CURVE ( )  B_SPLINE_CURVE ( 2, ( #16751, #2380, #8012, #13664, #4025, #9672, #1259, #12550, #18237 ),
 .UNSPECIFIED., .F., .T. ) 
 B_SPLINE_CURVE_WITH_KNOTS ( ( 3, 2, 2, 2, 3 ),
 ( 0.6637931034482759118, 0.6666666666666666297, 0.6724137931034482873, 0.6781609195402298340, 0.6810344827586206629 ),
 .UNSPECIFIED. ) 
 CURVE ( )  GEOMETRIC_REPRESENTATION_ITEM ( )  RATIONAL_B_SPLINE_CURVE ( ( 0.9330127018922194093, 0.9330127018922206306, 1.000000000000000000, 0.8660254037844387076, 1.000000000000000000, 0.8660254037844387076, 1.000000000000000000, 0.9330127018922194093, 0.9330127018922194093 ) ) 
 REPRESENTATION_ITEM ( '' )  );
#13729=CARTESIAN_POINT ( 'NONE',  ( -3.999999999999997335, -23.65934051745766808, -13.53387784049778197 ) ) ;
#13731=CARTESIAN_POINT ( 'NONE',  ( 2.121784821874994176, -23.46922363519303190, -2.828809719502837439 ) ) ;
#13733=CARTESIAN_POINT ( 'NONE',  ( -4.000000000000000888, -24.30356238220903364, -10.42760410546358152 ) ) ;
#13734=AXIS2_PLACEMENT_3D ( 'NONE', #12264, #15256, #10970 ) ;
#13735=CARTESIAN_POINT ( 'NONE',  ( 2.121784821875004390, -20.68551404134514016, -11.66773074662423149 ) ) ;
#13736=AXIS2_PLACEMENT_3D ( 'NONE', #4768, #4492, #10420 ) ;
#13740=EDGE_LOOP ( 'NONE', ( #13679, #10555, #10688, #10611, #17647, #12128 ) ) ;
#13745=CYLINDRICAL_SURFACE ( 'NONE', #3316, 4.000000000000000000 ) ;
#13746=CARTESIAN_POINT ( 'NONE',  ( 4.000000000000003553, -22.19672060476252184, -11.44504012756083888 ) ) ;
#13750=CARTESIAN_POINT ( 'NONE',  ( -2.121784821875005722, -27.60972853510210001, -8.742063539214022683 ) ) ;
#13756=CARTESIAN_POINT ( 'NONE',  ( -4.243569643749997233, -22.43105049029164277, -12.02487009106222615 ) ) ;
#13760=CARTESIAN_POINT ( 'NONE',  ( 0.000000000000000000, 9.254131787996968228, 30.52396275209373044 ) ) ;
#13761=CARTESIAN_POINT ( 'NONE',  ( 2.121784821874994176, -24.46939754608015605, -4.257206096731771083 ) ) ;
#13762=FACE_OUTER_BOUND ( 'NONE', #12568, .T. ) ;
#13763=CARTESIAN_POINT ( 'NONE',  ( 1.071796769724500109, -21.87733644393529531, -13.93638155029631420 ) ) ;
#13771=CARTESIAN_POINT ( 'NONE',  ( -2.121784821875005722, -25.06089824606716476, -5.101956642404802622 ) ) ;
#13776=CARTESIAN_POINT ( 'NONE',  ( 4.000000000000000888, -21.78699576701389873, -6.833574510138848090 ) ) ;
#13777=CARTESIAN_POINT ( 'NONE',  ( -2.121784821875005722, -29.67460370596585406, -11.69101089865440457 ) ) ;
#13778=CARTESIAN_POINT ( 'NONE',  ( -3.291771655530798757, -28.93493258167780269, -13.02337503524261386 ) ) ;
#13779=DIRECTION ( 'NONE',  ( -1.000000000000000000, 0.000000000000000000, 0.000000000000000000 ) ) ;
#13781=CARTESIAN_POINT ( 'NONE',  ( 4.243569643750003451, -23.51726086663143533, -13.57613927493450667 ) ) ;
#13782=ORIENTED_EDGE ( 'NONE', *, *, #726, .F. ) ;
#13784=CARTESIAN_POINT ( 'NONE',  ( -1.999999999999996225, -18.41164193897483869, -8.052546529193282510 ) ) ;
#13791=UNCERTAINTY_MEASURE_WITH_UNIT (LENGTH_MEASURE( 1.000000000000000082E-05 ), #15992, 'distance_accuracy_value', 'NONE');
#13792=CARTESIAN_POINT ( 'NONE',  ( -4.000000000000004441, -22.23763558379183181, -3.450836959150351824 ) ) ;
#13795=EDGE_CURVE ( 'NONE', #9873, #8773, #13547, .T. ) ;
#13796=ORIENTED_EDGE ( 'NONE', *, *, #5017, .F. ) ;
#13797=CARTESIAN_POINT ( 'NONE',  ( -4.243569643750004339, -27.69246697702454441, -10.99597133594720333 ) ) ;
#13799=CARTESIAN_POINT ( 'NONE',  ( 1.999999999999994449, -24.15142112668919339, -4.170847014031824784 ) ) ;
#13801=DIRECTION ( 'NONE',  ( -0.000000000000000000, -0.5735764363510414965, -0.8191520442889950182 ) ) ;
#13803=DIRECTION ( 'NONE',  ( 0.000000000000000000, 0.000000000000000000, 1.000000000000000000 ) ) ;
#13805=( BOUNDED_CURVE ( )  B_SPLINE_CURVE ( 2, ( #4125, #5511, #2746, #7323, #11157, #10100, #3268, #13078, #3080 ),
 .UNSPECIFIED., .F., .T. ) 
 B_SPLINE_CURVE_WITH_KNOTS ( ( 3, 2, 2, 2, 3 ),
 ( 0.1637931034482758563, 0.1666666666666666574, 0.1724137931034482873, 0.1781609195402298895, 0.1810344827586206906 ),
 .UNSPECIFIED. ) 
 CURVE ( )  GEOMETRIC_REPRESENTATION_ITEM ( )  RATIONAL_B_SPLINE_CURVE ( ( 0.9330127018922194093, 0.9330127018922194093, 1.000000000000000000, 0.8660254037844387076, 1.000000000000000000, 0.8660254037844387076, 1.000000000000000000, 0.9330127018922194093, 0.9330127018922194093 ) ) 
 REPRESENTATION_ITEM ( '' )  );
#13806=CARTESIAN_POINT ( 'NONE',  ( -4.243569643749997233, -21.14050350850180138, -10.18177799141198747 ) ) ;
#13809=ORIENTED_EDGE ( 'NONE', *, *, #10323, .F. ) ;
#13811=CARTESIAN_POINT ( 'NONE',  ( 4.000000000000003553, -22.51935735091492674, -11.90581315348016567 ) ) ;
#13812=CARTESIAN_POINT ( 'NONE',  ( 4.000000000000003553, -23.22915819019439709, -12.91951380728103160 ) ) ;
#13817=ADVANCED_FACE ( 'NONE', ( #4119, #9768 ), #14037, .T. ) ;
#13818=CARTESIAN_POINT ( 'NONE',  ( 4.000000000000000888, -27.01371104396771017, -14.29809751472907919 ) ) ;
#13822=CARTESIAN_POINT ( 'NONE',  ( 3.999999999999996447, -27.05567764914059481, -10.33171413117790394 ) ) ;
#13824=CARTESIAN_POINT ( 'NONE',  ( 2.121784821874994176, -22.69489544611912279, -1.722954459712693787 ) ) ;
#13828=CARTESIAN_POINT ( 'NONE',  ( -2.121784821875005722, -27.86783793146007326, -9.110681959144070419 ) ) ;
#13833=ORIENTED_EDGE ( 'NONE', *, *, #4057, .T. ) ;
#13835=PLANE ( 'NONE',  #3142 ) ;
#13836=CARTESIAN_POINT ( 'NONE',  ( -1.071796769724496334, -21.27353689998724562, -13.07406643513510858 ) ) ;
#13837=ORIENTED_EDGE ( 'NONE', *, *, #13411, .F. ) ;
#13839=CARTESIAN_POINT ( 'NONE',  ( -2.121784821874996396, -20.90060520497677743, -11.97491276323260756 ) ) ;
#13844=CARTESIAN_POINT ( 'NONE',  ( 4.243569643750000786, -24.28743054458419692, -10.40456545371456620 ) ) ;
#13851=CARTESIAN_POINT ( 'NONE',  ( -0.9009826423167719422, -10.00000000000000178, -12.54001985818077181 ) ) ;
#13852=EDGE_CURVE ( 'NONE', #3584, #269, #15502, .T. ) ;
#13855=CARTESIAN_POINT ( 'NONE',  ( 2.121784821875004390, -18.87874826683935936, -9.087401807113897334 ) ) ;
#13856=CARTESIAN_POINT ( 'NONE',  ( -3.999999999999997335, -24.94988749924751303, -15.37696994014802065 ) ) ;
#13858=EDGE_CURVE ( 'NONE', #12967, #9005, #11188, .T. ) ;
#13860=CARTESIAN_POINT ( 'NONE',  ( 3.999999999999996447, -25.31343922442924921, -7.843539797656847057 ) ) ;
#13862=CARTESIAN_POINT ( 'NONE',  ( -2.000000000000005773, -28.06608030478504290, -9.761559716304219592 ) ) ;
#13868=CARTESIAN_POINT ( 'NONE',  ( 4.243569643750000786, -20.93200839193060148, -5.612525994623947412 ) ) ;
#13871=CARTESIAN_POINT ( 'NONE',  ( 0.000000000000000000, 5.977523610840987267, 32.81826849749789687 ) ) ;
#13872=CARTESIAN_POINT ( 'NONE',  ( 2.121784821874994176, -29.37347607688156259, -11.26095607540267807 ) ) ;
#13873=CARTESIAN_POINT ( 'NONE',  ( 4.898587196589412829E-16, -10.00099999999999767, -4.000000000000000000 ) ) ;
#13877=CARTESIAN_POINT ( 'NONE',  ( -4.243569643749997233, -24.20555259025267603, -14.55912172808130656 ) ) ;
#13878=ORIENTED_EDGE ( 'NONE', *, *, #15856, .F. ) ;
#13879=CARTESIAN_POINT ( 'NONE',  ( -4.000000000000004441, -25.59305773644542370, -8.242876418240973280 ) ) ;
#13880=CARTESIAN_POINT ( 'NONE',  ( 4.000000000000000888, -21.85152311680833748, -6.925729116128124474 ) ) ;
#13883=CARTESIAN_POINT ( 'NONE',  ( 3.999999999999996447, -24.28100163899738106, -6.369066117936657889 ) ) ;
#13890=CARTESIAN_POINT ( 'NONE',  ( 4.730628863548789710E-15, -22.01578123233109707, -15.70329423968597915 ) ) ;
#13892=CARTESIAN_POINT ( 'NONE',  ( -1.999999999999996225, -17.57278640010649795, -6.854536663413863806 ) ) ;
#13898=VECTOR ( 'NONE', #4383, 1000.000000000000000 ) ;
#13899=CARTESIAN_POINT ( 'NONE',  ( 4.243569643749996345, -25.28344594435018067, -7.555532749933418835 ) ) ;
#13901=MANIFOLD_SOLID_BREP ( 'Cavity1', #5841 ) ;
#13903=AXIS2_PLACEMENT_3D ( 'NONE', #15395, #9625, #6930 ) ;
#13906=CARTESIAN_POINT ( 'NONE',  ( 4.000000000000003553, -22.26124795455695704, -11.53719473355011793 ) ) ;
#13912=CARTESIAN_POINT ( 'NONE',  ( -5.330712181944245322E-15, -23.94572221871285578, -1.373575165951426369 ) ) ;
#13915=CARTESIAN_POINT ( 'NONE',  ( 4.000000000000003553, -22.97104879383642384, -12.55089538735098387 ) ) ;
#13917=TOROIDAL_SURFACE ( 'NONE', #10657, 4.400000000000002132, 0.4000000000000000222 ) ;
#13918=CARTESIAN_POINT ( 'NONE',  ( 4.243569643750000786, -19.89957080649872623, -4.138052314903757356 ) ) ;
#13921=( BOUNDED_CURVE ( )  B_SPLINE_CURVE ( 2, ( #2713, #5565, #10854, #16532, #1228, #8071, #2620, #16632, #7983 ),
 .UNSPECIFIED., .F., .F. ) 
 B_SPLINE_CURVE_WITH_KNOTS ( ( 3, 2, 2, 2, 3 ),
 ( 0.1810344827586206906, 0.1839080459770114917, 0.1896551724137930939, 0.1954022988505747238, 0.1982758620689655249 ),
 .UNSPECIFIED. ) 
 CURVE ( )  GEOMETRIC_REPRESENTATION_ITEM ( )  RATIONAL_B_SPLINE_CURVE ( ( 0.9330127018922194093, 0.9330127018922194093, 1.000000000000000000, 0.8660254037844387076, 1.000000000000000000, 0.8660254037844387076, 1.000000000000000000, 0.9330127018922194093, 0.9330127018922194093 ) ) 
 REPRESENTATION_ITEM ( '' )  );
#13922=CARTESIAN_POINT ( 'NONE',  ( -1.661723472263481630E-14, -21.09148155414254688, -12.81406445585025544 ) ) ;
#13923=CARTESIAN_POINT ( 'NONE',  ( 4.243569643750000786, -22.96461988824960443, -8.515396051573073777 ) ) ;
#13924=EDGE_CURVE ( 'NONE', #15144, #13588, #11775, .T. ) ;
#13931=CYLINDRICAL_SURFACE ( 'NONE', #6683, 4.000000000000000000 ) ;
#13936=CARTESIAN_POINT ( 'NONE',  ( 4.243569643749996345, -26.79983864795324422, -9.721165967022450616 ) ) ;
#13939=CARTESIAN_POINT ( 'NONE',  ( 0.000000000000000000, 9.254131787996968228, 30.52396275209373044 ) ) ;
#13941=CARTESIAN_POINT ( 'NONE',  ( 4.243569643749996345, -25.54155534070815392, -7.924151169863466571 ) ) ;
#13942=CARTESIAN_POINT ( 'NONE',  ( 0.8866433558360066192, -9.999999999998044231, -3.510284692354058045 ) ) ;
#13944=CARTESIAN_POINT ( 'NONE',  ( -3.706921591972381904E-14, -18.96207903348436119, -9.772962490420598058 ) ) ;
#13945=CARTESIAN_POINT ( 'NONE',  ( -4.243569643750000786, -21.54501820828076930, -6.487994741957813005 ) ) ;
#13946=LINE ( 'NONE', #5506, #6789 ) ;
#13951=DIRECTION ( 'NONE',  ( -0.000000000000000000, -0.5735764363510414965, -0.8191520442889950182 ) ) ;
#13953=DIRECTION ( 'NONE',  ( 0.8191520442889951292, 0.4698463103929519935, -0.3289899283371605643 ) ) ;
#13954=ORIENTED_EDGE ( 'NONE', *, *, #8396, .F. ) ;
#13955=B_SPLINE_CURVE_WITH_KNOTS ( 'NONE', 3,
 ( #780, #6612, #2271, #5310, #10962, #16645, #13648, #3648, #14885, #967, #17942, #4939, #5214, #17677 ),
 .UNSPECIFIED., .F., .F.,
 ( 4, 2, 2, 2, 2, 2, 4 ),
 ( 0.000000000000000000, 0.002175243210657258879, 0.004350486421314517758, 0.008700972842629035517, 0.01087621605328629310, 0.01305145926394355588, 0.01740194568525808144 ),
 .UNSPECIFIED. ) ;
#13956=CARTESIAN_POINT ( 'NONE',  ( -5.330712181944246111E-15, -26.04286106412135027, -4.368599827883064890 ) ) ;
#13963=CARTESIAN_POINT ( 'NONE',  ( 2.121784821875004390, -23.26660800492483006, -15.35391494592470885 ) ) ;
#13966=CARTESIAN_POINT ( 'NONE',  ( -4.000000000000004441, -23.85081931173408165, -5.754702084719914623 ) ) ;
#13968=VERTEX_POINT ( 'NONE', #1709 ) ;
#13969=CARTESIAN_POINT ( 'NONE',  ( 1.071796769724490339, -22.13544584029325435, -14.30499997022636727 ) ) ;
#13971=EDGE_CURVE ( 'NONE', #16888, #17673, #3380, .T. ) ;
#13979=CARTESIAN_POINT ( 'NONE',  ( -2.121784821875005722, -28.15821100236278696, -9.525377681565375454 ) ) ;
#13985=DIRECTION ( 'NONE',  ( -0.000000000000000000, 1.000000000000000000, -0.000000000000000000 ) ) ;
#13986=LINE ( 'NONE', #8326, #589 ) ;
#13988=CARTESIAN_POINT ( 'NONE',  ( -4.243569643749997233, -20.36617531942789228, -9.075922731621842487 ) ) ;
#13990=CARTESIAN_POINT ( 'NONE',  ( -2.451037035742412051, -29.65081295030892505, -12.49886881493011437 ) ) ;
#13992=CARTESIAN_POINT ( 'NONE',  ( 4.000000000000003553, -22.77746674727289289, -12.27443157341021163 ) ) ;
#13993=CARTESIAN_POINT ( 'NONE',  ( 2.000000000000004441, -22.26177376727626367, -13.55110462547639472 ) ) ;
#13997=CARTESIAN_POINT ( 'NONE',  ( 3.999999999999996447, -28.66886137708284110, -12.63557925674746762 ) ) ;
#14003=CARTESIAN_POINT ( 'NONE',  ( -4.000000000000000888, -23.20659744698271965, -8.860975819754113303 ) ) ;
#14007=CARTESIAN_POINT ( 'NONE',  ( -1.071796769724486564, -27.52716991099435973, -8.057605589732816043 ) ) ;
#14008=CARTESIAN_POINT ( 'NONE',  ( 2.121784821874994176, -26.53427271694390299, -7.206153456172153859 ) ) ;
#14009=VECTOR ( 'NONE', #14249, 1000.000000000000000 ) ;
#14010=CARTESIAN_POINT ( 'NONE',  ( 2.000000000000004441, -21.48744557820235457, -12.44524936568625151 ) ) ;
#14014=CARTESIAN_POINT ( 'NONE',  ( -4.000000000000000888, -23.27112479677715839, -8.953130425743392351 ) ) ;
#14015=ORIENTED_EDGE ( 'NONE', *, *, #1047, .T. ) ;
#14016=ORIENTED_EDGE ( 'NONE', *, *, #14431, .T. ) ;
#14018=CARTESIAN_POINT ( 'NONE',  ( -3.999999999999997335, -20.04580896844610649, -8.373219961477113671 ) ) ;
#14021=ORIENTED_EDGE ( 'NONE', *, *, #15325, .T. ) ;
#14023=CARTESIAN_POINT ( 'NONE',  ( 2.121784821875004390, -20.42740464498717401, -11.29911232669418197 ) ) ;
#14025=EDGE_CURVE ( 'NONE', #18076, #17255, #18118, .T. ) ;
#14027=CARTESIAN_POINT ( 'NONE',  ( -3.706921591972381904E-14, -17.99416879784692469, -8.390643416689682610 ) ) ;
#14028=EDGE_CURVE ( 'NONE', #6628, #7899, #9474, .T. ) ;
#14029=CYLINDRICAL_SURFACE ( 'NONE', #1375, 7.499999999999999112 ) ;
#14031=CARTESIAN_POINT ( 'NONE',  ( 4.730628863548789710E-15, -20.20901545782531628, -13.12296530017564500 ) ) ;
#14034=DIRECTION ( 'NONE',  ( 0.000000000000000000, 0.000000000000000000, 1.000000000000000000 ) ) ;
#14035=CARTESIAN_POINT ( 'NONE',  ( -5.330712181944245322E-15, -25.49437859686066332, -3.585285685531713451 ) ) ;
#14036=CARTESIAN_POINT ( 'NONE',  ( -1.999999999999996225, -24.02552130905571204, -16.06999716166505721 ) ) ;
#14037=PLANE ( 'NONE',  #8819 ) ;
#14039=DIRECTION ( 'NONE',  ( -0.000000000000000000, -0.5735764363510414965, -0.8191520442889950182 ) ) ;
#14040=LINE ( 'NONE', #11251, #61 ) ;
#14042=CARTESIAN_POINT ( 'NONE',  ( -9.831267214419536771, -9.942687138680838643, 1.765148412673711142 ) ) ;
#14043=EDGE_CURVE ( 'NONE', #7315, #14839, #17524, .T. ) ;
#14045=CARTESIAN_POINT ( 'NONE',  ( 2.121784821875004390, -18.39479314866817461, -8.396242269745057385 ) ) ;
#14049=DIRECTION ( 'NONE',  ( 0.000000000000000000, 0.000000000000000000, 1.000000000000000000 ) ) ;
#14050=CARTESIAN_POINT ( 'NONE',  ( 3.999999999999996447, -28.34622463093043621, -12.17480623082814262 ) ) ;
#14051=CARTESIAN_POINT ( 'NONE',  ( 15.00000000000000355, -10.00000000000000000, 30.00000000000000000 ) ) ;
#14052=CARTESIAN_POINT ( 'NONE',  ( -4.243569643749997233, -24.72177138296861898, -15.29635856794139848 ) ) ;
#14054=CARTESIAN_POINT ( 'NONE',  ( -1.071796769724486564, -26.94642376848398158, -7.228214143883440634 ) ) ;
#14055=CARTESIAN_POINT ( 'NONE',  ( 4.000000000000003553, -20.19637278369320299, -8.588247374109736043 ) ) ;
#14057=VERTEX_POINT ( 'NONE', #9382 ) ;
#14063=CARTESIAN_POINT ( 'NONE',  ( -5.330712181944246111E-15, -29.14017382041697957, -8.792020867043637722 ) ) ;
#14065=VERTEX_POINT ( 'NONE', #3732 ) ;
#14068=( BOUNDED_CURVE ( )  B_SPLINE_CURVE ( 3, ( #17482, #11504, #4649, #8818 ),
 .UNSPECIFIED., .F., .T. ) 
 B_SPLINE_CURVE_WITH_KNOTS ( ( 4, 4 ),
 ( 4.712388980384689674, 6.283185307179586232 ),
 .UNSPECIFIED. ) 
 CURVE ( )  GEOMETRIC_REPRESENTATION_ITEM ( )  RATIONAL_B_SPLINE_CURVE ( ( 1.000000000000000000, 0.8047378541243649375, 0.8047378541243649375, 1.000000000000000000 ) ) 
 REPRESENTATION_ITEM ( '' )  );
#14072=EDGE_CURVE ( 'NONE', #2835, #10774, #13955, .T. ) ;
#14073=CARTESIAN_POINT ( 'NONE',  ( 4.243569643750000786, -22.99688356279435197, -8.561473354064329300 ) ) ;
#14075=EDGE_CURVE ( 'NONE', #9076, #5876, #7935, .T. ) ;
#14078=CARTESIAN_POINT ( 'NONE',  ( 2.000000000000004441, -22.32630111707070242, -13.64325923146567199 ) ) ;
#14080=CARTESIAN_POINT ( 'NONE',  ( 3.579096709490575479E-14, -23.64400226490599266, -2.511867456126184894 ) ) ;
#14081=DIRECTION ( 'NONE',  ( -0.000000000000000000, -0.000000000000000000, -1.000000000000000000 ) ) ;
#14083=ADVANCED_FACE ( 'NONE', ( #15150 ), #13554, .F. ) ;
#14086=CARTESIAN_POINT ( 'NONE',  ( -5.279047395330986450E-15, -30.34552082656112759, -11.00377920042669722 ) ) ;
#14090=CARTESIAN_POINT ( 'NONE',  ( 3.999999999999996447, -26.02324006370871601, -8.857240451457712993 ) ) ;
#14091=ORIENTED_EDGE ( 'NONE', *, *, #10523, .F. ) ;
#14093=CARTESIAN_POINT ( 'NONE',  ( 2.000000000000004441, -17.93844137898523527, -7.376746092654861364 ) ) ;
#14098=CARTESIAN_POINT ( 'NONE',  ( -4.243569643750000786, -22.83556519007061425, -8.331086841608051685 ) ) ;
#14104=ORIENTED_EDGE ( 'NONE', *, *, #10144, .F. ) ;
#14109=CARTESIAN_POINT ( 'NONE',  ( 1.071796769724495224, -17.74758610220779431, -8.038486831415553979 ) ) ;
#14110=CARTESIAN_POINT ( 'NONE',  ( -3.999999999999997335, -25.01441484904194823, -15.46912454613729793 ) ) ;
#14113=CARTESIAN_POINT ( 'NONE',  ( 2.121784821874994176, -25.75994452787000100, -6.100298196382009763 ) ) ;
#14116=CARTESIAN_POINT ( 'NONE',  ( 7.056670106005041632, -10.00000000000000178, -9.351700598554229416 ) ) ;
#14119=CARTESIAN_POINT ( 'NONE',  ( 2.121784821875004390, -21.49210590496380036, -12.81966330890563022 ) ) ;
#14122=CARTESIAN_POINT ( 'NONE',  ( 8.500000000000019540, 0.000000000000000000, -20.49999999999998934 ) ) ;
#14123=VECTOR ( 'NONE', #8371, 1000.000000000000000 ) ;
#14124=CARTESIAN_POINT ( 'NONE',  ( 4.243569643750003451, -19.12940112854596819, -7.309626136123695161 ) ) ;
#14129=CARTESIAN_POINT ( 'NONE',  ( -2.121784821874996396, -23.48169916855646733, -15.66109696253308314 ) ) ;
#14131=FACE_BOUND ( 'NONE', #3645, .T. ) ;
#14139=CARTESIAN_POINT ( 'NONE',  ( -5.330712181944246111E-15, -30.14034773130410372, -10.22041724427257137 ) ) ;
#14144=CARTESIAN_POINT ( 'NONE',  ( -4.243569643750005227, -26.62776571704792161, -9.475420353735755086 ) ) ;
#14145=ORIENTED_EDGE ( 'NONE', *, *, #15907, .T. ) ;
#14147=CARTESIAN_POINT ( 'NONE',  ( 4.000000000000000888, -20.30286673866052283, -4.714018596547838946 ) ) ;
#14151=AXIS2_PLACEMENT_3D ( 'NONE', #11168, #16860, #4136 ) ;
#14157=EDGE_LOOP ( 'NONE', ( #9650, #12257, #14170, #8024 ) ) ;
#14158=CARTESIAN_POINT ( 'NONE',  ( 4.243569643750000786, -24.54553994094216307, -10.77318387364461572 ) ) ;
#14165=LINE ( 'NONE', #1206, #6773 ) ;
#14168=CARTESIAN_POINT ( 'NONE',  ( -2.000000000000005773, -23.42011117034160605, -3.126428157563360344 ) ) ;
#14169=CARTESIAN_POINT ( 'NONE',  ( -2.121784821875005722, -24.80278884970919506, -4.733338222474753998 ) ) ;
#14170=ORIENTED_EDGE ( 'NONE', *, *, #5783, .T. ) ;
#14173=CARTESIAN_POINT ( 'NONE',  ( -4.000000000000004441, -26.94813206802970740, -10.17812312388048746 ) ) ;
#14174=CARTESIAN_POINT ( 'NONE',  ( 4.898587196589413815E-16, 2.700915433685006750, 35.11257424290206330 ) ) ;
#14179=CARTESIAN_POINT ( 'NONE',  ( -3.999999999999997335, -23.98197726361007298, -13.99465086641710698 ) ) ;
#14181=EDGE_CURVE ( 'NONE', #6360, #3748, #4824, .T. ) ;
#14184=EDGE_CURVE ( 'NONE', #17065, #17116, #4110, .T. ) ;
#14185=CARTESIAN_POINT ( 'NONE',  ( -4.000000000000004441, -25.85116713280339695, -8.611494838171019239 ) ) ;
#14186=( BOUNDED_CURVE ( )  B_SPLINE_CURVE ( 2, ( #12754, #8393, #8475, #4313, #18077, #13879, #11264, #14054, #16953 ),
 .UNSPECIFIED., .F., .T. ) 
 B_SPLINE_CURVE_WITH_KNOTS ( ( 3, 2, 2, 2, 3 ),
 ( 0.4568965517241379559, 0.4597701149425287293, 0.4655172413793103314, 0.4712643678160919336, 0.4741379310344827624 ),
 .UNSPECIFIED. ) 
 CURVE ( )  GEOMETRIC_REPRESENTATION_ITEM ( )  RATIONAL_B_SPLINE_CURVE ( ( 0.9330127018922194093, 0.9330127018922200755, 1.000000000000000000, 0.8660254037844387076, 1.000000000000000000, 0.8660254037844387076, 1.000000000000000000, 0.9330127018922187432, 0.9330127018922194093 ) ) 
 REPRESENTATION_ITEM ( '' )  );
#14188=DIRECTION ( 'NONE',  ( 0.000000000000000000, 0.8191520442889952403, -0.5735764363510413855 ) ) ;
#14190=CARTESIAN_POINT ( 'NONE',  ( 9.852650557354193595, -9.939667866509505956, 9.673467103803176315 ) ) ;
#14192=CARTESIAN_POINT ( 'NONE',  ( -4.243569643750004339, -25.07910933890011052, -7.263709834155468670 ) ) ;
#14194=CARTESIAN_POINT ( 'NONE',  ( -3.999999999999997335, -18.04546114737679829, -5.516427208026009943 ) ) ;
#14199=CARTESIAN_POINT ( 'NONE',  ( -8.999999999999994671, -10.00000000000000178, 15.14468620625657103 ) ) ;
#14202=CARTESIAN_POINT ( 'NONE',  ( -5.577813053751546416E-15, -26.22509622848567545, -6.198051655426662698 ) ) ;
#14203=ORIENTED_EDGE ( 'NONE', *, *, #6152, .F. ) ;
#14205=CARTESIAN_POINT ( 'NONE',  ( -2.121784821874996396, -19.61005822318693248, -10.13182066358236888 ) ) ;
#14212=CARTESIAN_POINT ( 'NONE',  ( 4.000000000000000888, -24.94883587310395967, -11.34915015528869731 ) ) ;
#14213=CARTESIAN_POINT ( 'NONE',  ( -4.243569643750005227, -24.59515422072892221, -6.572550296786629609 ) ) ;
#14215=CIRCLE ( 'NONE', #10954, 4.000000000000000000 ) ;
#14219=CARTESIAN_POINT ( 'NONE',  ( -1.999999999999996225, -18.15353254261686899, -7.683928109263233885 ) ) ;
#14220=CARTESIAN_POINT ( 'NONE',  ( 4.243569643749996345, -22.67008830622574322, -3.823271248141685508 ) ) ;
#14228=DIRECTION ( 'NONE',  ( 0.000000000000000000, 0.000000000000000000, -1.000000000000000000 ) ) ;
#14231=CARTESIAN_POINT ( 'NONE',  ( -4.243569643749998122, -18.30130014856414533, -6.126975372181462376 ) ) ;
#14234=CARTESIAN_POINT ( 'NONE',  ( 1.999999999999994449, -22.60276474854137874, -1.959136494451539035 ) ) ;
#14235=APPLICATION_CONTEXT ( 'automotive_design' ) ;
#14236=CARTESIAN_POINT ( 'NONE',  ( -5.330712181944246111E-15, -29.10791014587222847, -8.745943564552382199 ) ) ;
#14240=CARTESIAN_POINT ( 'NONE',  ( 2.121784821875004390, -21.71795162677701896, -13.14220442634442243 ) ) ;
#14242=CARTESIAN_POINT ( 'NONE',  ( -1.999999999999996225, -16.86298556082702760, -5.840836009612994317 ) ) ;
#14247=CARTESIAN_POINT ( 'NONE',  ( 2.856226148085021954, -24.67072674863668169, -15.86966854801251081 ) ) ;
#14249=DIRECTION ( 'NONE',  ( -0.000000000000000000, -0.5735764363510414965, -0.8191520442889950182 ) ) ;
#14251=ADVANCED_FACE ( 'NONE', ( #4011 ), #9654, .F. ) ;
#14252=EDGE_LOOP ( 'NONE', ( #5895, #6513, #2697, #17240, #13185, #13470 ) ) ;
#14253=CARTESIAN_POINT ( 'NONE',  ( 4.730628863548789710E-15, -19.69279666510938043, -12.38572846031554953 ) ) ;
#14256=VERTEX_POINT ( 'NONE', #1331 ) ;
#14259=CARTESIAN_POINT ( 'NONE',  ( 4.299564228933482956E-15, -19.28471577963676964, -10.23373551633992307 ) ) ;
#14260=CARTESIAN_POINT ( 'NONE',  ( -8.500000000000005329, 10.00000000000000000, 20.49999999999999645 ) ) ;
#14262=CARTESIAN_POINT ( 'NONE',  ( -1.661723472263481630E-14, -21.28506360070608139, -13.09052826979102946 ) ) ;
#14263=CARTESIAN_POINT ( 'NONE',  ( -4.243569643750000786, -20.80295369375161130, -5.428216784658927985 ) ) ;
#14266=VERTEX_POINT ( 'NONE', #8617 ) ;
#14267=EDGE_LOOP ( 'NONE', ( #9356, #16631, #5467, #11054 ) ) ;
#14268=CARTESIAN_POINT ( 'NONE',  ( -2.000000000000005773, -23.22652912377807510, -2.849964343622590324 ) ) ;
#14277=CARTESIAN_POINT ( 'NONE',  ( 2.000000000000004441, -20.19689859641251317, -10.60215726603601283 ) ) ;
#14278=EDGE_LOOP ( 'NONE', ( #17352, #10098, #8146, #13696 ) ) ;
#14285=CARTESIAN_POINT ( 'NONE',  ( 4.243569643750000786, -22.44840109553366858, -7.778159211712977417 ) ) ;
#14291=EDGE_CURVE ( 'NONE', #11559, #6787, #16100, .T. ) ;
#14293=AXIS2_PLACEMENT_3D ( 'NONE', #14340, #11540, #15640 ) ;
#14294=CARTESIAN_POINT ( 'NONE',  ( -1.071796769724505882, -18.24075149348606573, -8.742800001963811241 ) ) ;
#14296=ORIENTED_EDGE ( 'NONE', *, *, #18289, .T. ) ;
#14298=CARTESIAN_POINT ( 'NONE',  ( 2.121784821874994176, -25.24372573515406515, -5.363061356521914291 ) ) ;
#14300=( BOUNDED_CURVE ( )  B_SPLINE_CURVE ( 2, ( #3593, #13595, #9243, #12111, #17982, #10723, #16400, #3685, #15008 ),
 .UNSPECIFIED., .F., .T. ) 
 B_SPLINE_CURVE_WITH_KNOTS ( ( 3, 2, 2, 2, 3 ),
 ( 0.3362068965517241437, 0.3390804597701149170, 0.3448275862068965747, 0.3505747126436781769, 0.3534482758620690057 ),
 .UNSPECIFIED. ) 
 CURVE ( )  GEOMETRIC_REPRESENTATION_ITEM ( )  RATIONAL_B_SPLINE_CURVE ( ( 0.9330127018922194093, 0.9330127018922200755, 1.000000000000000000, 0.8660254037844387076, 1.000000000000000000, 0.8660254037844387076, 1.000000000000000000, 0.9330127018922187432, 0.9330127018922194093 ) ) 
 REPRESENTATION_ITEM ( '' )  );
#14303=CARTESIAN_POINT ( 'NONE',  ( 0.000000000000000000, 5.977523610840987267, 32.81826849749789687 ) ) ;
#14304=CARTESIAN_POINT ( 'NONE',  ( -2.121784821875005722, -26.35144522785700616, -6.945048742055040414 ) ) ;
#14308=CARTESIAN_POINT ( 'NONE',  ( 0.5553297335976642435, -10.00000000000086686, -4.810349131761211261 ) ) ;
#14309=EDGE_CURVE ( 'NONE', #14256, #13681, #1625, .T. ) ;
#14312=CARTESIAN_POINT ( 'NONE',  ( -4.000000000000000888, -24.75525382513053430, -11.07268633933439972 ) ) ;
#14313=CARTESIAN_POINT ( 'NONE',  ( -2.121784821875005722, -23.22186879701663642, -2.475550400403212503 ) ) ;
#14319=CARTESIAN_POINT ( 'NONE',  ( 4.243569643750000786, -26.83626083361913217, -14.04467235052378804 ) ) ;
#14323=FACE_OUTER_BOUND ( 'NONE', #7645, .T. ) ;
#14325=CARTESIAN_POINT ( 'NONE',  ( -4.243569643749998122, -18.04319075220617563, -5.758356952251413752 ) ) ;
#14327=CARTESIAN_POINT ( 'NONE',  ( -4.243569643750000786, -26.48136041362692339, -13.53782202311997551 ) ) ;
#14329=CARTESIAN_POINT ( 'NONE',  ( -5.330712181944246111E-15, -29.88223833494613402, -9.851798824342527183 ) ) ;
#14331=VECTOR ( 'NONE', #7629, 1000.000000000000000 ) ;
#14334=CARTESIAN_POINT ( 'NONE',  ( -4.243569643749997233, -22.65689621210486138, -12.34741120850101836 ) ) ;
#14335=CARTESIAN_POINT ( 'NONE',  ( 0.000000000000000000, 5.977523610840987267, 32.81826849749789687 ) ) ;
#14336=CARTESIAN_POINT ( 'NONE',  ( 4.000000000000003553, -19.16393519826133485, -7.113773694389545099 ) ) ;
#14338=EDGE_LOOP ( 'NONE', ( #12283, #762, #7542, #4357, #12333, #16417, #14104, #7302, #14726 ) ) ;
#14340=CARTESIAN_POINT ( 'NONE',  ( 0.000000000000000000, 5.977523610840987267, 32.81826849749789687 ) ) ;
#14342=CARTESIAN_POINT ( 'NONE',  ( 4.000000000000003553, -21.42239241568860564, -10.33918486777069745 ) ) ;
#14345=CARTESIAN_POINT ( 'NONE',  ( 4.243569643750003451, -22.25897755938633793, -11.77912447777552174 ) ) ;
#14349=CARTESIAN_POINT ( 'NONE',  ( 3.999999999999996447, -24.73269308191887461, -7.014148351807473425 ) ) ;
#14350=CARTESIAN_POINT ( 'NONE',  ( 2.121784821875004390, -22.26643409403770590, -13.92551856869577342 ) ) ;
#14354=CARTESIAN_POINT ( 'NONE',  ( 2.121784821874994176, -23.72733303155099804, -3.197428139432884286 ) ) ;
#14355=EDGE_CURVE ( 'NONE', #17116, #17908, #1040, .T. ) ;
#14356=ORIENTED_EDGE ( 'NONE', *, *, #13200, .T. ) ;
#14357=CARTESIAN_POINT ( 'NONE',  ( 2.000000000000004441, -20.19689859641251317, -10.60215726603601283 ) ) ;
#14361=ADVANCED_FACE ( 'NONE', ( #850 ), #12394, .T. ) ;
#14362=CARTESIAN_POINT ( 'NONE',  ( 8.500000000000019540, 10.00000000000000000, -20.49999999999998934 ) ) ;
#14369=CARTESIAN_POINT ( 'NONE',  ( 1.999999999999994449, -26.73251509026887618, -7.857031213332303921 ) ) ;
#14373=CARTESIAN_POINT ( 'NONE',  ( 3.999999999999996447, 6.938893903907228378E-15, 24.28148006742132026 ) ) ;
#14374=CARTESIAN_POINT ( 'NONE',  ( 2.121784821875004390, -18.36252947412342351, -8.350164967253801862 ) ) ;
#14377=EDGE_CURVE ( 'NONE', #1806, #15033, #9204, .T. ) ;
#14387=CARTESIAN_POINT ( 'NONE',  ( 4.243569643750003451, -21.19427629940971869, -10.25857349556407527 ) ) ;
#14391=CARTESIAN_POINT ( 'NONE',  ( -1.999999999999996225, -24.28363070541367819, -16.43861558159510494 ) ) ;
#14393=CARTESIAN_POINT ( 'NONE',  ( -4.243569643750005227, -24.33704482437095251, -6.203931876856584537 ) ) ;
#14396=CARTESIAN_POINT ( 'NONE',  ( -5.940121053391560935, -10.00000000000000178, -9.400027718825146650 ) ) ;
#14399=( BOUNDED_CURVE ( )  B_SPLINE_CURVE ( 2, ( #2221, #14929, #7848, #16675, #12292, #12387, #816, #17713, #6553 ),
 .UNSPECIFIED., .F., .T. ) 
 B_SPLINE_CURVE_WITH_KNOTS ( ( 3, 2, 2, 2, 3 ),
 ( 0.6982758620689655249, 0.7011494252873563537, 0.7068965517241379004, 0.7126436781609195581, 0.7155172413793103869 ),
 .UNSPECIFIED. ) 
 CURVE ( )  GEOMETRIC_REPRESENTATION_ITEM ( )  RATIONAL_B_SPLINE_CURVE ( ( 0.9330127018922194093, 0.9330127018922194093, 1.000000000000000000, 0.8660254037844387076, 1.000000000000000000, 0.8660254037844387076, 1.000000000000000000, 0.9330127018922180770, 0.9330127018922194093 ) ) 
 REPRESENTATION_ITEM ( '' )  );
#14400=CARTESIAN_POINT ( 'NONE',  ( -2.121784821875005722, -23.47997819337460257, -2.844168820333258907 ) ) ;
#14406=CARTESIAN_POINT ( 'NONE',  ( -2.121784821874996396, -23.73980856491443703, -16.02971538246313443 ) ) ;
#14413=CARTESIAN_POINT ( 'NONE',  ( 4.730628863548789710E-15, -16.07926511609781883, -7.225070581294880334 ) ) ;
#14415=CARTESIAN_POINT ( 'NONE',  ( -2.121784821875005722, -29.44875798415262835, -11.36846978121561236 ) ) ;
#14420=CARTESIAN_POINT ( 'NONE',  ( 2.121784821875004390, -23.00849860856686036, -14.98529652599465933 ) ) ;
#14421=CARTESIAN_POINT ( 'NONE',  ( -3.706921591972381904E-14, -16.70362181605707619, -6.547551317039444818 ) ) ;
#14425=CARTESIAN_POINT ( 'NONE',  ( 2.121784821875004390, -21.20173283406107956, -12.40496758648432518 ) ) ;
#14427=CARTESIAN_POINT ( 'NONE',  ( -2.000000000000005773, -23.22652912377807510, -2.849964343622590324 ) ) ;
#14431=EDGE_CURVE ( 'NONE', #317, #16065, #16268, .T. ) ;
#14435=CARTESIAN_POINT ( 'NONE',  ( 1.999999999999994449, -26.21629629755294033, -7.119794373472207560 ) ) ;
#14438=( BOUNDED_CURVE ( )  B_SPLINE_CURVE ( 2, ( #5333, #2384, #2656, #13860, #1349, #6632, #10890, #9495, #11071 ),
 .UNSPECIFIED., .F., .F. ) 
 B_SPLINE_CURVE_WITH_KNOTS ( ( 3, 2, 2, 2, 3 ),
 ( 0.4741379310344827624, 0.4770114942528735358, 0.4827586206896551935, 0.4885057471264367956, 0.4913793103448276245 ),
 .UNSPECIFIED. ) 
 CURVE ( )  GEOMETRIC_REPRESENTATION_ITEM ( )  RATIONAL_B_SPLINE_CURVE ( ( 0.9330127018922194093, 0.9330127018922200755, 1.000000000000000000, 0.8660254037844387076, 1.000000000000000000, 0.8660254037844387076, 1.000000000000000000, 0.9330127018922187432, 0.9330127018922194093 ) ) 
 REPRESENTATION_ITEM ( '' )  );
#14439=EDGE_LOOP ( 'NONE', ( #281, #17429, #10822, #1390, #6565, #1364, #4986 ) ) ;
#14440=CARTESIAN_POINT ( 'NONE',  ( 4.243569643749997233, -26.05777413342408622, -8.661388009723561154 ) ) ;
#14443=CARTESIAN_POINT ( 'NONE',  ( 15.00000000000000355, -10.00000000000000000, -30.00000000000000000 ) ) ;
#14445=AXIS2_PLACEMENT_3D ( 'NONE', #4825, #841, #6482 ) ;
#14446=CARTESIAN_POINT ( 'NONE',  ( -2.121784821875005722, -28.93253919143669251, -10.63123294135551689 ) ) ;
#14447=DIRECTION ( 'NONE',  ( -0.000000000000000000, 1.000000000000000000, -0.000000000000000000 ) ) ;
#14448=CIRCLE ( 'NONE', #14445, 3.000000000000001776 ) ;
#14454=CARTESIAN_POINT ( 'NONE',  ( 4.243569643750000786, -21.96444597736247673, -7.086999674344137468 ) ) ;
#14459=EDGE_LOOP ( 'NONE', ( #9313, #1558, #180, #749 ) ) ;
#14468=EDGE_LOOP ( 'NONE', ( #9343, #10189, #6217, #11887 ) ) ;
#14472=CARTESIAN_POINT ( 'NONE',  ( 4.000000000000003553, -20.64806422661470720, -9.233329607980554243 ) ) ;
#14474=CARTESIAN_POINT ( 'NONE',  ( 1.071796769724485232, -24.14869435690309984, -3.232642461330365702 ) ) ;
#14476=CARTESIAN_POINT ( 'NONE',  ( -5.993188111103413540, -10.31462179351540875, 0.09365451271231550745 ) ) ;
#14477=CARTESIAN_POINT ( 'NONE',  ( 4.243569643750003451, -20.16183871397783633, -8.784099815843886105 ) ) ;
#14485=FACE_OUTER_BOUND ( 'NONE', #4820, .T. ) ;
#14486=CARTESIAN_POINT ( 'NONE',  ( 3.999999999999996891, -2.343145750507611424, 25.02027108472329786 ) ) ;
#14487=CARTESIAN_POINT ( 'NONE',  ( 3.999999999999996447, -26.79756825278262511, -9.963095711247856201 ) ) ;
#14490=CARTESIAN_POINT ( 'NONE',  ( -4.648177544792955347E-16, -29.58051838113927090, -10.99009111451728415 ) ) ;
#14491=CARTESIAN_POINT ( 'NONE',  ( -5.330712181944245322E-15, -25.49437859686066332, -3.585285685531713451 ) ) ;
#14495=CARTESIAN_POINT ( 'NONE',  ( -4.243569643750004339, -28.98301395881438580, -12.83906343559744201 ) ) ;
#14498=CARTESIAN_POINT ( 'NONE',  ( -2.121784821874996396, -19.12610310501574418, -9.440661126213528931 ) ) ;
#14502=CARTESIAN_POINT ( 'NONE',  ( -3.706921591972381904E-14, -18.76849698692083379, -9.496498676479825818 ) ) ;
#14507=CARTESIAN_POINT ( 'NONE',  ( -6.938893903907228378E-15, 6.938893903907228378E-15, 30.00000000000000000 ) ) ;
#14508=CARTESIAN_POINT ( 'NONE',  ( 4.000000000000003553, -18.64771640554539545, -6.376536854529449627 ) ) ;
#14509=ORIENTED_EDGE ( 'NONE', *, *, #5024, .F. ) ;
#14511=CARTESIAN_POINT ( 'NONE',  ( -4.243569643750000786, -26.70720613544014199, -13.86036314055876772 ) ) ;
#14513=CARTESIAN_POINT ( 'NONE',  ( 4.299564228933482956E-15, -22.89824732864832768, -15.39439339536058959 ) ) ;
#14514=CARTESIAN_POINT ( 'NONE',  ( 6.079313232897375130, -14.44302855110184680, -4.023496914807076941 ) ) ;
#14517=CARTESIAN_POINT ( 'NONE',  ( -4.243569643750005227, -28.46679516609844995, -12.10182659573734476 ) ) ;
#14518=VECTOR ( 'NONE', #5708, 999.9999999999998863 ) ;
#14520=CARTESIAN_POINT ( 'NONE',  ( -2.121784821875005722, -28.38405672417600911, -9.847918799004165891 ) ) ;
#14521=( BOUNDED_CURVE ( )  B_SPLINE_CURVE ( 2, ( #5272, #2327, #16418, #13614, #6662, #6570, #4056, #9348, #9708 ),
 .UNSPECIFIED., .F., .T. ) 
 B_SPLINE_CURVE_WITH_KNOTS ( ( 3, 2, 2, 2, 3 ),
 ( 0.7327586206896552490, 0.7356321839080459668, 0.7413793103448276245, 0.7471264367816091712, 0.7500000000000000000 ),
 .UNSPECIFIED. ) 
 CURVE ( )  GEOMETRIC_REPRESENTATION_ITEM ( )  RATIONAL_B_SPLINE_CURVE ( ( 0.9330127018922194093, 0.9330127018922206306, 1.000000000000000000, 0.8660254037844387076, 1.000000000000000000, 0.8660254037844387076, 1.000000000000000000, 0.9330127018922194093, 0.9330127018922194093 ) ) 
 REPRESENTATION_ITEM ( '' )  );
#14522=LINE ( 'NONE', #10136, #1391 ) ;
#14524=CARTESIAN_POINT ( 'NONE',  ( 1.533898589781675205E-14, -28.22544404955499786, -9.054844408877768203 ) ) ;
#14525=CARTESIAN_POINT ( 'NONE',  ( 4.243569643750003451, -23.25915147027346563, -13.20752085500445894 ) ) ;
#14527=CARTESIAN_POINT ( 'NONE',  ( 0.000000000000000000, -15.45745613286697839, -10.86990606519494129 ) ) ;
#14528=CARTESIAN_POINT ( 'NONE',  ( 2.000000000000004441, -17.68033198262726913, -7.008127672724814516 ) ) ;
#14530=ORIENTED_EDGE ( 'NONE', *, *, #5783, .F. ) ;
#14535=CARTESIAN_POINT ( 'NONE',  ( 4.000000000000000888, -26.75560164760974047, -13.92947909479903146 ) ) ;
#14539=CARTESIAN_POINT ( 'NONE',  ( -2.121784821874996396, -20.93286887952152497, -12.02099006572386486 ) ) ;
#14542=CARTESIAN_POINT ( 'NONE',  ( 3.999999999999996447, -21.95801707177565731, -3.051500338566227377 ) ) ;
#14543=CARTESIAN_POINT ( 'NONE',  ( 2.121784821874994176, -28.88952095871037429, -10.56979653803383989 ) ) ;
#14544=CARTESIAN_POINT ( 'NONE',  ( -4.000000000000000888, -25.33599996764090534, -11.90207778518377246 ) ) ;
#14548=CARTESIAN_POINT ( 'NONE',  ( 2.121784821875004390, -18.91101194138411046, -9.133479109605152857 ) ) ;
#14554=CARTESIAN_POINT ( 'NONE',  ( 4.898587196589409870E-16, 4.000000000000007105, -4.000000000000000000 ) ) ;
#14557=VERTEX_POINT ( 'NONE', #15027 ) ;
#14558=CYLINDRICAL_SURFACE ( 'NONE', #8358, 4.000000000000000000 ) ;
#14559=CARTESIAN_POINT ( 'NONE',  ( 0.000000000000000000, 0.000000000000000000, 0.000000000000000000 ) ) ;
#14564=MECHANICAL_DESIGN_GEOMETRIC_PRESENTATION_REPRESENTATION('',(#7725),#3591);
#14566=CARTESIAN_POINT ( 'NONE',  ( -3.999999999999997335, -20.04580896844610649, -8.373219961477115447 ) ) ;
#14567=EDGE_LOOP ( 'NONE', ( #14814, #10128, #11340, #9053 ) ) ;
#14570=CARTESIAN_POINT ( 'NONE',  ( -7.076011672040958267, -12.11284110773042144, 11.47761944861337469 ) ) ;
#14571=CARTESIAN_POINT ( 'NONE',  ( -2.121784821875005722, -24.77052517516444752, -4.687260919983497587 ) ) ;
#14579=CARTESIAN_POINT ( 'NONE',  ( 4.000000000000000888, -24.88430852330952447, -11.25699554929942003 ) ) ;
#14583=CARTESIAN_POINT ( 'NONE',  ( 2.121784821874994176, -24.46939754608015605, -4.257206096731771083 ) ) ;
#14585=VECTOR ( 'NONE', #1122, 1000.000000000000000 ) ;
#14588=CARTESIAN_POINT ( 'NONE',  ( 4.243569643750003451, -25.09818091932399398, -15.83392709700605039 ) ) ;
#14589=CARTESIAN_POINT ( 'NONE',  ( -4.000000000000004441, -28.69037049274105300, -12.66629745740154434 ) ) ;
#14591=CARTESIAN_POINT ( 'NONE',  ( 4.730628863548789710E-15, -16.59548390881375468, -7.962307421154977582 ) ) ;
#14593=CARTESIAN_POINT ( 'NONE',  ( 0.2979626678773949489, -10.00000000000000178, -4.943697222988730822 ) ) ;
#14596=AXIS2_PLACEMENT_3D ( 'NONE', #14559, #11848, #11660 ) ;
#14603=AXIS2_PLACEMENT_3D ( 'NONE', #9802, #8672, #5812 ) ;
#14606=CARTESIAN_POINT ( 'NONE',  ( -4.243569643750005227, -28.17642209519573271, -11.68713087331604150 ) ) ;
#14610=LINE ( 'NONE', #6154, #17684 ) ;
#14615=CARTESIAN_POINT ( 'NONE',  ( 2.610817815249942608, -22.30731692868453564, -2.152029956302548008 ) ) ;
#14617=CARTESIAN_POINT ( 'NONE',  ( -4.243569643749998122, -22.14067741938892908, -11.61017436864092112 ) ) ;
#14618=DIRECTION ( 'NONE',  ( -0.000000000000000000, -0.5735764363510414965, -0.8191520442889950182 ) ) ;
#14622=CARTESIAN_POINT ( 'NONE',  ( -5.330712181944245322E-15, -26.78492557865051538, -5.428377785181952575 ) ) ;
#14625=DIRECTION ( 'NONE',  ( -0.000000000000000000, -0.5735764363510414965, -0.8191520442889950182 ) ) ;
#14627=EDGE_CURVE ( 'NONE', #4281, #16392, #11687, .T. ) ;
#14628=CARTESIAN_POINT ( 'NONE',  ( 0.000000000000000000, 5.977523610840987267, 32.81826849749789687 ) ) ;
#14630=CARTESIAN_POINT ( 'NONE',  ( 1.533898589781675205E-14, -27.77375260663349366, -8.409762175006950002 ) ) ;
#14631=CARTESIAN_POINT ( 'NONE',  ( -3.999999999999997335, -24.49819605632600883, -14.73188770627720245 ) ) ;
#14635=CARTESIAN_POINT ( 'NONE',  ( -4.243569643750004339, -25.11137301344485451, -7.309787136646725081 ) ) ;
#14637=( BOUNDED_CURVE ( )  B_SPLINE_CURVE ( 2, ( #9031, #2007, #1723, #7545, #4673, #11622, #16004, #4581, #10227 ),
 .UNSPECIFIED., .F., .T. ) 
 B_SPLINE_CURVE_WITH_KNOTS ( ( 3, 2, 2, 2, 3 ),
 ( 0.2500000000000000000, 0.2528735632183908288, 0.2586206896551724310, 0.2643678160919540332, 0.2672413793103448620 ),
 .UNSPECIFIED. ) 
 CURVE ( )  GEOMETRIC_REPRESENTATION_ITEM ( )  RATIONAL_B_SPLINE_CURVE ( ( 0.9330127018922194093, 0.9330127018922190762, 1.000000000000000000, 0.8660254037844387076, 1.000000000000000000, 0.8660254037844387076, 1.000000000000000000, 0.9330127018922187432, 0.9330127018922194093 ) ) 
 REPRESENTATION_ITEM ( '' )  );
#14642=CARTESIAN_POINT ( 'NONE',  ( -2.121784821874996396, -22.48152525766933962, -14.23270058530414950 ) ) ;
#14643=CARTESIAN_POINT ( 'NONE',  ( 4.000000000000003553, -24.77781456834220464, -15.13122432686131802 ) ) ;
#14644=CARTESIAN_POINT ( 'NONE',  ( -4.000000000000000888, -25.85221876035684474, -12.63931462504386793 ) ) ;
#14645=CARTESIAN_POINT ( 'NONE',  ( -2.000000000000005773, -27.80797090842707320, -9.392941296374171856 ) ) ;
#14646=CARTESIAN_POINT ( 'NONE',  ( -4.243569643749997233, -17.78508135584820948, -5.389738532321366904 ) ) ;
#14648=CARTESIAN_POINT ( 'NONE',  ( 0.000000000000000000, -27.20729309053124112, -14.57456132866985321 ) ) ;
#14649=CARTESIAN_POINT ( 'NONE',  ( 3.999999999999996447, -25.05532982807127951, -7.474921377726800209 ) ) ;
#14660=VERTEX_POINT ( 'NONE', #8490 ) ;
#14662=CARTESIAN_POINT ( 'NONE',  ( 4.000000000000003553, -20.90617362297267690, -9.601948027910603756 ) ) ;
#14663=ORIENTED_EDGE ( 'NONE', *, *, #9829, .F. ) ;
#14664=EDGE_CURVE ( 'NONE', #13443, #4345, #15212, .T. ) ;
#14665=CARTESIAN_POINT ( 'NONE',  ( -1.661723472263481630E-14, -21.34959095050052014, -13.18268287578030318 ) ) ;
#14670=CARTESIAN_POINT ( 'NONE',  ( 2.121784821874994176, -24.98561633879609545, -4.994442936591867443 ) ) ;
#14672=EDGE_CURVE ( 'NONE', #8639, #1548, #14165, .T. ) ;
#14683=CARTESIAN_POINT ( 'NONE',  ( -4.243569643750005227, -23.27234356439432972, -4.683380894645135406 ) ) ;
#14687=CARTESIAN_POINT ( 'NONE',  ( -4.243569643750004339, -28.72490456245641255, -12.47044501566739427 ) ) ;
#14688=CARTESIAN_POINT ( 'NONE',  ( -4.000000000000000888, -25.78769141056240954, -12.54716001905459066 ) ) ;
#14689=CARTESIAN_POINT ( 'NONE',  ( -4.243569643750000786, -21.31917248646755070, -6.165453624519022569 ) ) ;
#14692=CARTESIAN_POINT ( 'NONE',  ( 1.533898589781675205E-14, -27.70922525683905846, -8.317607569017670954 ) ) ;
#14697=DIRECTION ( 'NONE',  ( -1.000000000000000000, 0.000000000000000000, 0.000000000000000000 ) ) ;
#14698=CARTESIAN_POINT ( 'NONE',  ( 1.071796769724485232, -23.89058496054513370, -2.864024041400317078 ) ) ;
#14702=CARTESIAN_POINT ( 'NONE',  ( 4.243569643750000786, -25.02949505911335137, -11.46434341101345389 ) ) ;
#14707=CARTESIAN_POINT ( 'NONE',  ( -2.797762022055394482E-14, -10.00000000000000178, -12.59063537424807677 ) ) ;
#14708=CARTESIAN_POINT ( 'NONE',  ( 2.121784821875004390, -22.52454349039567205, -14.29413698862582294 ) ) ;
#14710=CARTESIAN_POINT ( 'NONE',  ( 4.730628863548789710E-15, -19.66053299056463288, -12.33965115782429400 ) ) ;
#14711=DIRECTION ( 'NONE',  ( -0.000000000000000000, -0.5735764363510414965, -0.8191520442889950182 ) ) ;
#14715=CARTESIAN_POINT ( 'NONE',  ( -2.121784821874996396, -20.90060520497677743, -11.97491276323260756 ) ) ;
#14717=CARTESIAN_POINT ( 'NONE',  ( -4.000000000000004441, -21.52783474451236145, -2.437136305349486332 ) ) ;
#14721=CARTESIAN_POINT ( 'NONE',  ( 1.071796769724485454, -20.58678946214543970, -12.09328945064608085 ) ) ;
#14723=CARTESIAN_POINT ( 'NONE',  ( 4.713407268011036227E-15, -21.61702609051053514, -14.64346846959108284 ) ) ;
#14726=ORIENTED_EDGE ( 'NONE', *, *, #16603, .T. ) ;
#14727=CARTESIAN_POINT ( 'NONE',  ( 4.730628863548789710E-15, -18.66035907967750163, -10.91125478059535858 ) ) ;
#14732=EDGE_CURVE ( 'NONE', #8704, #13968, #11195, .T. ) ;
#14734=CARTESIAN_POINT ( 'NONE',  ( -2.121784821875005722, -28.15821100236278696, -9.525377681565375454 ) ) ;
#14736=CARTESIAN_POINT ( 'NONE',  ( 9.320906609362770823, -9.992678237866394753, -2.177225805445022644 ) ) ;
#14737=LINE ( 'NONE', #13328, #2883 ) ;
#14738=CARTESIAN_POINT ( 'NONE',  ( 4.243569643750000786, -19.89957080649872623, -4.138052314903757356 ) ) ;
#14740=CARTESIAN_POINT ( 'NONE',  ( -1.661723472263481630E-14, -20.76884480799014554, -12.35329142993093576 ) ) ;
#14741=CARTESIAN_POINT ( 'NONE',  ( 3.999999999999996447, -24.79722043171331336, -7.106302957796752473 ) ) ;
#14742=LINE ( 'NONE', #13334, #11174 ) ;
#14746=CARTESIAN_POINT ( 'NONE',  ( 1.999999999999994449, -27.05515183642128108, -8.317804239251627152 ) ) ;
#14747=CARTESIAN_POINT ( 'NONE',  ( -8.999999999999992895, -13.00000000000000000, -3.713574246709377746 ) ) ;
#14754=CARTESIAN_POINT ( 'NONE',  ( 4.000000000000000888, -21.78699576701389873, -6.833574510138848090 ) ) ;
#14761=CARTESIAN_POINT ( 'NONE',  ( -4.243569643750004339, -23.53045296075229942, -5.051999314575183142 ) ) ;
#14762=CARTESIAN_POINT ( 'NONE',  ( 4.243569643749996345, -25.54155534070815392, -7.924151169863466571 ) ) ;
#14765=CARTESIAN_POINT ( 'NONE',  ( -4.950315044628286643, -10.00000000000096811, 20.01801554166341646 ) ) ;
#14768=CARTESIAN_POINT ( 'NONE',  ( 3.999999999999996447, -24.02289224263940426, -6.000447698006609265 ) ) ;
#14769=CARTESIAN_POINT ( 'NONE',  ( -4.243569643749997233, -25.01214445387132912, -15.71105429036270351 ) ) ;
#14770=ORIENTED_EDGE ( 'NONE', *, *, #8744, .F. ) ;
#14771=STYLED_ITEM('',(#18389),#13901);
#14775=CARTESIAN_POINT ( 'NONE',  ( 2.121784821875004390, -18.36252947412342351, -8.350164967253801862 ) ) ;
#14778=CARTESIAN_POINT ( 'NONE',  ( -4.243569643749998122, -24.75403505751336297, -15.34243587043265400 ) ) ;
#14779=CARTESIAN_POINT ( 'NONE',  ( 4.000000000000003553, -24.77781456834220464, -15.13122432686131802 ) ) ;
#14780=CARTESIAN_POINT ( 'NONE',  ( 4.243569643750003451, -18.90355540673274248, -6.987085018684902948 ) ) ;
#14784=DIRECTION ( 'NONE',  ( -0.000000000000000000, -0.000000000000000000, -1.000000000000000000 ) ) ;
#14788=EDGE_LOOP ( 'NONE', ( #3375, #11332, #2703, #18095 ) ) ;
#14790=CARTESIAN_POINT ( 'NONE',  ( -2.121784821875005722, -22.70565000430070057, -1.738313560543115477 ) ) ;
#14795=EDGE_CURVE ( 'NONE', #2069, #9984, #9893, .T. ) ;
#14796=CARTESIAN_POINT ( 'NONE',  ( -2.121784821875005722, -28.12594732781803941, -9.479300379074118155 ) ) ;
#14799=DIRECTION ( 'NONE',  ( 0.000000000000000000, 0.000000000000000000, -1.000000000000000000 ) ) ;
#14800=CARTESIAN_POINT ( 'NONE',  ( 3.537103074283489246, -10.00000000000000178, -11.53856502750720203 ) ) ;
#14801=CARTESIAN_POINT ( 'NONE',  ( -4.243569643750000786, -24.93270403547910874, -11.32611150353969087 ) ) ;
#14802=LINE ( 'NONE', #13018, #8133 ) ;
#14803=CARTESIAN_POINT ( 'NONE',  ( 4.243569643750000786, -24.25516687003944938, -10.35848815122331068 ) ) ;
#14809=CARTESIAN_POINT ( 'NONE',  ( 4.730628863548789710E-15, -19.66053299056463288, -12.33965115782429400 ) ) ;
#14812=DIRECTION ( 'NONE',  ( 0.000000000000000000, 0.8191520442889952403, -0.5735764363510413855 ) ) ;
#14814=ORIENTED_EDGE ( 'NONE', *, *, #11357, .F. ) ;
#14816=CARTESIAN_POINT ( 'NONE',  ( -1.071796769724487675, -23.40293942064543486, -16.11516840056477662 ) ) ;
#14821=CARTESIAN_POINT ( 'NONE',  ( -4.243569643750000786, -22.60971946825739209, -8.008545724169261248 ) ) ;
#14831=CARTESIAN_POINT ( 'NONE',  ( 8.500000000000019540, 0.000000000000000000, -22.49999999999999289 ) ) ;
#14832=CARTESIAN_POINT ( 'NONE',  ( 4.243569643750000786, -20.41578959921466918, -4.875289154763852828 ) ) ;
#14834=CARTESIAN_POINT ( 'NONE',  ( 1.071796769724495224, -19.81246127307154836, -10.98743419085593409 ) ) ;
#14836=CARTESIAN_POINT ( 'NONE',  ( -2.000000000000005773, -26.32384188007369730, -7.273385382783162711 ) ) ;
#14839=VERTEX_POINT ( 'NONE', #17057 ) ;
#14842=EDGE_CURVE ( 'NONE', #12048, #2315, #4222, .T. ) ;
#14847=EDGE_CURVE ( 'NONE', #17808, #7377, #11646, .T. ) ;
#14851=CARTESIAN_POINT ( 'NONE',  ( 3.999999999999996447, -24.21647428920293876, -6.276911511947378841 ) ) ;
#14853=DIRECTION ( 'NONE',  ( -0.000000000000000000, -0.5735764363510414965, -0.8191520442889950182 ) ) ;
#14855=CARTESIAN_POINT ( 'NONE',  ( 1.475796370471763337E-14, -22.05939178977998694, -14.19638352958117267 ) ) ;
#14856=CARTESIAN_POINT ( 'NONE',  ( 4.243569643749997233, -22.41197890986777352, -3.454652828211637772 ) ) ;
#14857=CARTESIAN_POINT ( 'NONE',  ( -2.121784821875005722, -26.60955462421497586, -7.313667161985088150 ) ) ;
#14858=CYLINDRICAL_SURFACE ( 'NONE', #4060, 4.000000000000000000 ) ;
#14859=VERTEX_POINT ( 'NONE', #17431 ) ;
#14861=CARTESIAN_POINT ( 'NONE',  ( 3.132887738848207260, -10.75727755901226779, 20.85177242120515473 ) ) ;
#14862=LINE ( 'NONE', #7788, #4537 ) ;
#14863=CARTESIAN_POINT ( 'NONE',  ( 4.000000000000000888, -22.10963251316630362, -7.294347536058173098 ) ) ;
#14864=CARTESIAN_POINT ( 'NONE',  ( -4.243569643750005227, -28.98301395881438580, -12.83906343559744201 ) ) ;
#14866=AXIS2_PLACEMENT_3D ( 'NONE', #13571, #7827, #4870 ) ;
#14868=CARTESIAN_POINT ( 'NONE',  ( 3.276967058447619152, -25.10900663730464188, -15.57833582608148326 ) ) ;
#14870=CARTESIAN_POINT ( 'NONE',  ( 4.243569643750003451, -19.90372931761987019, -8.415481395913838369 ) ) ;
#14873=CARTESIAN_POINT ( 'NONE',  ( 4.243569643750000786, -25.83608692273200802, -12.61627597329485440 ) ) ;
#14874=CARTESIAN_POINT ( 'NONE',  ( -3.999999999999997335, -23.91744991381563779, -13.90249626042782793 ) ) ;
#14875=CARTESIAN_POINT ( 'NONE',  ( 4.730628863548789710E-15, -16.85359330517172083, -8.330925841085024430 ) ) ;
#14878=CARTESIAN_POINT ( 'NONE',  ( -6.428571428571425272, -14.26578344203648285, -2.827263138854410496 ) ) ;
#14880=EDGE_LOOP ( 'NONE', ( #10188, #12615, #9633, #8885 ) ) ;
#14881=ORIENTED_EDGE ( 'NONE', *, *, #2441, .F. ) ;
#14882=CARTESIAN_POINT ( 'NONE',  ( 2.121784821875004390, -16.81387309597561242, -6.138454447673516334 ) ) ;
#14884=CARTESIAN_POINT ( 'NONE',  ( -6.158835246850665095E-15, -22.31750118613795664, -14.56500194951122218 ) ) ;
#14885=CARTESIAN_POINT ( 'NONE',  ( 7.485948097525552569, -12.69170840778861731, 7.144968677233840104 ) ) ;
#14886=ORIENTED_EDGE ( 'NONE', *, *, #11691, .T. ) ;
#14890=CARTESIAN_POINT ( 'NONE',  ( -4.243569643750005227, -27.66020330247980041, -10.94989403345594425 ) ) ;
#14893=CARTESIAN_POINT ( 'NONE',  ( -5.577813053751546416E-15, -23.57947491511155036, -2.419712850136908511 ) ) ;
#14894=CARTESIAN_POINT ( 'NONE',  ( 1.598251304517956273, -15.40332308709066211, -10.50456014341326849 ) ) ;
#14896=CARTESIAN_POINT ( 'NONE',  ( -4.243569643749997233, -23.97970686843945742, -14.23658061064251257 ) ) ;
#14898=AXIS2_PLACEMENT_3D ( 'NONE', #151, #8480, #15472 ) ;
#14902=CARTESIAN_POINT ( 'NONE',  ( -2.000000000000005773, -29.09851789021691815, -11.23603339602441054 ) ) ;
#14904=CARTESIAN_POINT ( 'NONE',  ( 4.243569643750000786, -23.99705747368147968, -9.989869731293264721 ) ) ;
#14905=VERTEX_POINT ( 'NONE', #2301 ) ;
#14906=FACE_OUTER_BOUND ( 'NONE', #9409, .T. ) ;
#14910=ORIENTED_EDGE ( 'NONE', *, *, #15287, .F. ) ;
#14914=AXIS2_PLACEMENT_3D ( 'NONE', #10668, #16436, #7795 ) ;
#14918=( BOUNDED_CURVE ( )  B_SPLINE_CURVE ( 2, ( #9742, #12706, #5303, #5394, #14014, #10955, #11306, #16639, #4273 ),
 .UNSPECIFIED., .F., .F. ) 
 B_SPLINE_CURVE_WITH_KNOTS ( ( 3, 2, 2, 2, 3 ),
 ( 0.4913793103448276245, 0.4942528735632183978, 0.5000000000000000000, 0.5057471264367816577, 0.5086206896551724865 ),
 .UNSPECIFIED. ) 
 CURVE ( )  GEOMETRIC_REPRESENTATION_ITEM ( )  RATIONAL_B_SPLINE_CURVE ( ( 0.9330127018922194093, 0.9330127018922200755, 1.000000000000000000, 0.8660254037844387076, 1.000000000000000000, 0.8660254037844387076, 1.000000000000000000, 0.9330127018922180770, 0.9330127018922194093 ) ) 
 REPRESENTATION_ITEM ( '' )  );
#14920=CARTESIAN_POINT ( 'NONE',  ( 4.243569643750000786, -22.22255537372044998, -7.455618094274186092 ) ) ;
#14925=CARTESIAN_POINT ( 'NONE',  ( -14.99999999999999645, -10.00000000000000000, 30.00000000000000000 ) ) ;
#14927=CARTESIAN_POINT ( 'NONE',  ( 9.985555166373632829, -9.918630114099121542, 7.321306590882093346 ) ) ;
#14929=CARTESIAN_POINT ( 'NONE',  ( -1.071796769724486786, -18.49886088984402832, -9.111418421893864306 ) ) ;
#14930=CARTESIAN_POINT ( 'NONE',  ( -2.121784821874996396, -23.99791796127240318, -16.39833380239318217 ) ) ;
#14932=CYLINDRICAL_SURFACE ( 'NONE', #12157, 4.000000000000000000 ) ;
#14933=CARTESIAN_POINT ( 'NONE',  ( -3.999999999999997335, -21.65899269638835278, -10.67708508704667913 ) ) ;
#14935=EDGE_LOOP ( 'NONE', ( #810, #4667 ) ) ;
#14936=CARTESIAN_POINT ( 'NONE',  ( 8.500000000000019540, 10.00000000000000000, 20.49999999999998934 ) ) ;
#14944=CARTESIAN_POINT ( 'NONE',  ( -5.279047395330986450E-15, -24.86069615324935356, -3.170637775906417488 ) ) ;
#14950=CARTESIAN_POINT ( 'NONE',  ( 2.121784821875004390, -21.75021530132177006, -13.18828172883567973 ) ) ;
#14952=CARTESIAN_POINT ( 'NONE',  ( 3.082316921986471225, -29.06618978543598786, -12.78463801463987437 ) ) ;
#14954=CARTESIAN_POINT ( 'NONE',  ( -5.526342620816817153, -10.00000000000000178, 19.09106094340727111 ) ) ;
#14956=CARTESIAN_POINT ( 'NONE',  ( 2.121784821875004390, -23.81509047218551700, -16.13722908827605806 ) ) ;
#14960=CARTESIAN_POINT ( 'NONE',  ( -4.243569643750005227, -21.72368718624651507, -2.471670375064849434 ) ) ;
#14963=CARTESIAN_POINT ( 'NONE',  ( 4.000000000000003553, -24.00348637926829909, -14.02536906707117659 ) ) ;
#14964=ORIENTED_EDGE ( 'NONE', *, *, #2817, .F. ) ;
#14965=CARTESIAN_POINT ( 'NONE',  ( -5.330712181944245322E-15, -25.01042347868947857, -2.894126148162874834 ) ) ;
#14968=CARTESIAN_POINT ( 'NONE',  ( 0.000000000000000000, 9.254131787996968228, 30.52396275209373044 ) ) ;
#14974=CARTESIAN_POINT ( 'NONE',  ( 0.000000000000000000, 5.977523610840987267, 32.81826849749789687 ) ) ;
#14975=ORIENTED_EDGE ( 'NONE', *, *, #4953, .F. ) ;
#14977=CARTESIAN_POINT ( 'NONE',  ( 4.243569643750000786, -23.99705747368147968, -9.989869731293264721 ) ) ;
#14979=CARTESIAN_POINT ( 'NONE',  ( 0.9009826423167504039, -10.00000000000000178, -12.54001985818112352 ) ) ;
#14980=CARTESIAN_POINT ( 'NONE',  ( -5.330712181944245322E-15, -28.88206442405900631, -8.423402447113588210 ) ) ;
#14983=CARTESIAN_POINT ( 'NONE',  ( -5.577813053751546416E-15, -29.51599103134483570, -10.89793650852800511 ) ) ;
#14985=CARTESIAN_POINT ( 'NONE',  ( -4.243569643749997233, -21.62445862667299323, -10.87293752878082742 ) ) ;
#14998=CARTESIAN_POINT ( 'NONE',  ( 4.243569643749997233, -25.02533654799221452, -7.186914330003371099 ) ) ;
#15003=FACE_OUTER_BOUND ( 'NONE', #15022, .T. ) ;
#15004=AXIS2_PLACEMENT_3D ( 'NONE', #8236, #11102, #16790 ) ;
#15006=CARTESIAN_POINT ( 'NONE',  ( -3.792279431941310452, -28.18008910945223278, -13.57208143547394918 ) ) ;
#15007=CARTESIAN_POINT ( 'NONE',  ( 4.299564228933482956E-15, -19.02660638327879994, -9.865117096409875330 ) ) ;
#15008=CARTESIAN_POINT ( 'NONE',  ( -1.661723472263481630E-14, -21.28506360070608139, -13.09052826979102946 ) ) ;
#15009=CARTESIAN_POINT ( 'NONE',  ( 2.121784821874994176, -22.69489544611912279, -1.722954459712693787 ) ) ;
#15010=ORIENTED_EDGE ( 'NONE', *, *, #14355, .T. ) ;
#15012=CARTESIAN_POINT ( 'NONE',  ( 3.999999999999996447, -24.53911103535534366, -6.737684537866704737 ) ) ;
#15015=ORIENTED_EDGE ( 'NONE', *, *, #4450, .T. ) ;
#15016=( BOUNDED_CURVE ( )  B_SPLINE_CURVE ( 2, ( #15443, #18234, #14219, #2911, #8287, #9939, #16931, #15528, #5686 ),
 .UNSPECIFIED., .F., .T. ) 
 B_SPLINE_CURVE_WITH_KNOTS ( ( 3, 2, 2, 2, 3 ),
 ( 0.8017241379310344751, 0.8045977011494253039, 0.8103448275862068506, 0.8160919540229885083, 0.8189655172413793371 ),
 .UNSPECIFIED. ) 
 CURVE ( )  GEOMETRIC_REPRESENTATION_ITEM ( )  RATIONAL_B_SPLINE_CURVE ( ( 0.9330127018922194093, 0.9330127018922194093, 1.000000000000000000, 0.8660254037844387076, 1.000000000000000000, 0.8660254037844387076, 1.000000000000000000, 0.9330127018922194093, 0.9330127018922194093 ) ) 
 REPRESENTATION_ITEM ( '' )  );
#15017=CARTESIAN_POINT ( 'NONE',  ( -4.648177544792955347E-16, -29.58051838113927090, -10.99009111451728415 ) ) ;
#15022=EDGE_LOOP ( 'NONE', ( #12983, #2761, #7373, #10828 ) ) ;
#15024=CARTESIAN_POINT ( 'NONE',  ( 3.999999999999996447, -23.18403670377106351, -4.802437832227187897 ) ) ;
#15027=CARTESIAN_POINT ( 'NONE',  ( 3.064183985264992582, -21.85725672082847382, -2.451266466499125052 ) ) ;
#15028=CARTESIAN_POINT ( 'NONE',  ( 4.243569643749997233, -22.15386951350980382, -3.086034408281590480 ) ) ;
#15030=CARTESIAN_POINT ( 'NONE',  ( 2.121784821874994176, -26.82464578784662379, -7.620849178593458007 ) ) ;
#15033=VERTEX_POINT ( 'NONE', #9241 ) ;
#15034=CARTESIAN_POINT ( 'NONE',  ( -3.544496300715703541, -10.00000000000000178, 23.01862375599376875 ) ) ;
#15035=CARTESIAN_POINT ( 'NONE',  ( 8.500000000000019540, 10.00000000000000000, 22.49999999999999289 ) ) ;
#15037=CARTESIAN_POINT ( 'NONE',  ( -2.000000000000005773, -25.54951369099979175, -6.167530122993019503 ) ) ;
#15041=CARTESIAN_POINT ( 'NONE',  ( 2.769796424106844235, -22.34959361326263760, -1.882087514909482229 ) ) ;
#15045=CARTESIAN_POINT ( 'NONE',  ( -4.000000000000004441, -27.14171411459323835, -10.45458693782125792 ) ) ;
#15046=ORIENTED_EDGE ( 'NONE', *, *, #10144, .T. ) ;
#15047=CARTESIAN_POINT ( 'NONE',  ( -5.330712181944245322E-15, -24.23609528961556947, -1.788270888372730960 ) ) ;
#15050=CARTESIAN_POINT ( 'NONE',  ( -5.577813053751546416E-15, -28.74166284227092305, -9.792081248737861898 ) ) ;
#15051=CARTESIAN_POINT ( 'NONE',  ( 1.071796769724495224, -21.03848090506694390, -12.73837168451689550 ) ) ;
#15059=FACE_OUTER_BOUND ( 'NONE', #13509, .T. ) ;
#15063=CARTESIAN_POINT ( 'NONE',  ( 2.121784821875004390, -20.68551404134514016, -11.66773074662423149 ) ) ;
#15069=CARTESIAN_POINT ( 'NONE',  ( 4.730628863548789710E-15, -21.24145304325719152, -14.59743897989583594 ) ) ;
#15072=CARTESIAN_POINT ( 'NONE',  ( -2.000000000000005773, -22.96841972742010540, -2.481345923692543920 ) ) ;
#15074=CARTESIAN_POINT ( 'NONE',  ( -2.121784821875005722, -25.54485336423835307, -5.793116179773641683 ) ) ;
#15083=DIRECTION ( 'NONE',  ( -0.000000000000000000, -0.5735764363510414965, -0.8191520442889950182 ) ) ;
#15084=EDGE_LOOP ( 'NONE', ( #3483, #14356, #5061, #15842 ) ) ;
#15085=CARTESIAN_POINT ( 'NONE',  ( -4.243569643750004339, -23.30460723893907371, -4.729458197136390929 ) ) ;
#15090=VECTOR ( 'NONE', #7379, 1000.000000000000000 ) ;
#15093=CARTESIAN_POINT ( 'NONE',  ( 4.243569643749997233, -28.86471381881699116, -12.67011332646283073 ) ) ;
#15095=CARTESIAN_POINT ( 'NONE',  ( 7.035635943437157813, -13.82009150476320869, -0.02313312325170999509 ) ) ;
#15097=CARTESIAN_POINT ( 'NONE',  ( 4.730628863548789710E-15, -21.98351755778634953, -15.65721693719472185 ) ) ;
#15100=CARTESIAN_POINT ( 'NONE',  ( 3.999999999999996447, -24.02289224263940781, -6.000447698006609265 ) ) ;
#15104=CARTESIAN_POINT ( 'NONE',  ( 2.000000000000004441, -19.48709775713304637, -9.588456612235146892 ) ) ;
#15111=CARTESIAN_POINT ( 'NONE',  ( -3.999999999999997335, -18.23904319394032569, -5.792891021966779519 ) ) ;
#15118=CARTESIAN_POINT ( 'NONE',  ( -2.121784821875005722, -23.73808758973257227, -3.212787240263307531 ) ) ;
#15120=ADVANCED_FACE ( 'NONE', ( #13684 ), #8385, .F. ) ;
#15121=( BOUNDED_CURVE ( )  B_SPLINE_CURVE ( 2, ( #9878, #11269, #9792, #16957, #11178, #8399, #4505, #2768, #7369 ),
 .UNSPECIFIED., .F., .T. ) 
 B_SPLINE_CURVE_WITH_KNOTS ( ( 3, 2, 2, 2, 3 ),
 ( 0.6293103448275861878, 0.6321839080459770166, 0.6379310344827586743, 0.6436781609195402210, 0.6465517241379310498 ),
 .UNSPECIFIED. ) 
 CURVE ( )  GEOMETRIC_REPRESENTATION_ITEM ( )  RATIONAL_B_SPLINE_CURVE ( ( 0.9330127018922194093, 0.9330127018922194093, 1.000000000000000000, 0.8660254037844387076, 1.000000000000000000, 0.8660254037844387076, 1.000000000000000000, 0.9330127018922194093, 0.9330127018922194093 ) ) 
 REPRESENTATION_ITEM ( '' )  );
#15122=CARTESIAN_POINT ( 'NONE',  ( 4.243569643749996345, -26.05777413342408622, -8.661388009723561154 ) ) ;
#15125=CARTESIAN_POINT ( 'NONE',  ( 4.299564228933482956E-15, -18.51038759056286054, -9.127880256549779858 ) ) ;
#15131=CARTESIAN_POINT ( 'NONE',  ( 4.000000000000003553, -25.10045131449460598, -15.59199735278064125 ) ) ;
#15135=CARTESIAN_POINT ( 'NONE',  ( 3.999999999999996447, -26.28134946006668571, -9.225858871387760729 ) ) ;
#15137=CARTESIAN_POINT ( 'NONE',  ( -2.121784821874996396, -17.57744672686793308, -7.228950606633243403 ) ) ;
#15139=CARTESIAN_POINT ( 'NONE',  ( 4.243569643749997233, -25.76740106252136542, -8.246692287302257895 ) ) ;
#15140=CARTESIAN_POINT ( 'NONE',  ( -1.071796769724496334, -29.26940833570569822, -10.54577992325387292 ) ) ;
#15143=CARTESIAN_POINT ( 'NONE',  ( 4.299564228933482956E-15, -19.28471577963676964, -10.23373551633992307 ) ) ;
#15144=VERTEX_POINT ( 'NONE', #6906 ) ;
#15145=ORIENTED_EDGE ( 'NONE', *, *, #14184, .T. ) ;
#15150=FACE_OUTER_BOUND ( 'NONE', #1688, .T. ) ;
#15153=CARTESIAN_POINT ( 'NONE',  ( -5.330712181944245322E-15, -27.55925376772441382, -6.534233044972094895 ) ) ;
#15159=CARTESIAN_POINT ( 'NONE',  ( -2.121784821874996396, -21.19097827587949467, -12.38960848565391260 ) ) ;
#15165=CARTESIAN_POINT ( 'NONE',  ( -4.243569643749997233, -19.30147405945127304, -7.555371749410396021 ) ) ;
#15167=ADVANCED_FACE ( 'NONE', ( #12651 ), #15980, .F. ) ;
#15168=CARTESIAN_POINT ( 'NONE',  ( -4.000000000000004441, -28.69037049274104945, -12.66629745740154611 ) ) ;
#15175=CYLINDRICAL_SURFACE ( 'NONE', #6011, 4.000000000000000000 ) ;
#15176=ORIENTED_EDGE ( 'NONE', *, *, #1744, .F. ) ;
#15178=CARTESIAN_POINT ( 'NONE',  ( -2.121784821875005722, -24.02846066063528596, -3.627482962684610346 ) ) ;
#15181=ORIENTED_EDGE ( 'NONE', *, *, #10960, .F. ) ;
#15183=FACE_OUTER_BOUND ( 'NONE', #17814, .T. ) ;
#15184=CARTESIAN_POINT ( 'NONE',  ( -4.243569643750004339, -28.69264088791166856, -12.42436771317613875 ) ) ;
#15186=CARTESIAN_POINT ( 'NONE',  ( 3.375445829055900404, -25.20600189401019264, -15.83707978931157534 ) ) ;
#15188=EDGE_CURVE ( 'NONE', #12907, #12502, #2351, .T. ) ;
#15190=CARTESIAN_POINT ( 'NONE',  ( 4.243569643749996345, -28.34849502610105176, -11.93287648660273703 ) ) ;
#15192=DIRECTION ( 'NONE',  ( -0.000000000000000000, -0.000000000000000000, -1.000000000000000000 ) ) ;
#15194=CARTESIAN_POINT ( 'NONE',  ( 2.000000000000004441, -18.45466017170117112, -8.113982932514955948 ) ) ;
#15199=CARTESIAN_POINT ( 'NONE',  ( 2.000000000000004441, -23.35873870250257767, -15.11773291118586293 ) ) ;
#15203=CARTESIAN_POINT ( 'NONE',  ( -1.999999999999996225, -17.57278640010649795, -6.854536663413863806 ) ) ;
#15205=ORIENTED_EDGE ( 'NONE', *, *, #15672, .T. ) ;
#15206=CARTESIAN_POINT ( 'NONE',  ( -4.243569643749998122, -23.46348807572352158, -13.49934377078241710 ) ) ;
#15208=CARTESIAN_POINT ( 'NONE',  ( 4.000000000000003553, -18.32507965939299055, -5.915763828610126396 ) ) ;
#15212=LINE ( 'NONE', #2692, #4120 ) ;
#15214=CARTESIAN_POINT ( 'NONE',  ( 4.730628863548789710E-15, -16.56322023426900714, -7.916230118663721171 ) ) ;
#15215=CARTESIAN_POINT ( 'NONE',  ( -2.121784821874996396, -19.90043129408965328, -10.54651638600367214 ) ) ;
#15218=CARTESIAN_POINT ( 'NONE',  ( 1.999999999999994449, -27.05515183642128108, -8.317804239251627152 ) ) ;
#15219=CARTESIAN_POINT ( 'NONE',  ( -1.661723472263481630E-14, -21.80128239342201724, -13.82776510965112671 ) ) ;
#15221=CARTESIAN_POINT ( 'NONE',  ( 9.000000000000003553, -4.000000000000000000, -30.00000000000000000 ) ) ;
#15225=CARTESIAN_POINT ( 'NONE',  ( 4.243569643750000786, -19.86730713195397868, -4.091975012412500945 ) ) ;
#15230=CARTESIAN_POINT ( 'NONE',  ( 2.000000000000004441, -21.74555497456032427, -12.81386778561629924 ) ) ;
#15233=CARTESIAN_POINT ( 'NONE',  ( -5.330712181944245322E-15, -24.49420468597353562, -2.156889308302778030 ) ) ;
#15235=( BOUNDED_CURVE ( )  B_SPLINE_CURVE ( 2, ( #6655, #17901, #12302, #6563, #3780, #18264, #16501, #15476, #9522 ),
 .UNSPECIFIED., .F., .F. ) 
 B_SPLINE_CURVE_WITH_KNOTS ( ( 3, 2, 2, 2, 3 ),
 ( 0.4741379310344827624, 0.4770114942528735358, 0.4827586206896551935, 0.4885057471264367956, 0.4913793103448276245 ),
 .UNSPECIFIED. ) 
 CURVE ( )  GEOMETRIC_REPRESENTATION_ITEM ( )  RATIONAL_B_SPLINE_CURVE ( ( 0.9330127018922194093, 0.9330127018922200755, 1.000000000000000000, 0.8660254037844387076, 1.000000000000000000, 0.8660254037844387076, 1.000000000000000000, 0.9330127018922187432, 0.9330127018922194093 ) ) 
 REPRESENTATION_ITEM ( '' )  );
#15236=FACE_OUTER_BOUND ( 'NONE', #2299, .T. ) ;
#15239=CARTESIAN_POINT ( 'NONE',  ( -4.243569643750000786, -24.90044036093436119, -11.28003420104843357 ) ) ;
#15240=CARTESIAN_POINT ( 'NONE',  ( 1.071796769724490339, -22.84524667957272470, -15.31870062402723320 ) ) ;
#15247=LINE ( 'NONE', #15513, #13193 ) ;
#15248=DIRECTION ( 'NONE',  ( -0.000000000000000000, -0.5735764363510414965, -0.8191520442889950182 ) ) ;
#15249=CARTESIAN_POINT ( 'NONE',  ( 0.000000000000000000, 5.977523610840987267, 32.81826849749789687 ) ) ;
#15252=CARTESIAN_POINT ( 'NONE',  ( 4.243569643750003451, -21.96860448848362779, -11.36442875535422026 ) ) ;
#15256=DIRECTION ( 'NONE',  ( -0.000000000000000000, -0.5735764363510414965, -0.8191520442889950182 ) ) ;
#15258=CARTESIAN_POINT ( 'NONE',  ( -4.243569643750005227, -26.40191999523469946, -9.152879236296964649 ) ) ;
#15259=CARTESIAN_POINT ( 'NONE',  ( 0.000000000000000000, -10.00000000000000178, -12.59063537424807677 ) ) ;
#15261=CARTESIAN_POINT ( 'NONE',  ( -1.999999999999996225, -17.89542314625890285, -7.315309689333185261 ) ) ;
#15262=DIRECTION ( 'NONE',  ( -0.000000000000000000, 1.000000000000000000, -0.000000000000000000 ) ) ;
#15263=CARTESIAN_POINT ( 'NONE',  ( 4.243569643750000786, -21.67407290645975948, -6.672303951922835097 ) ) ;
#15265=DIRECTION ( 'NONE',  ( -0.000000000000000000, -0.5735764363510414965, -0.8191520442889950182 ) ) ;
#15266=DIRECTION ( 'NONE',  ( -0.000000000000000000, -0.5735764363510414965, -0.8191520442889950182 ) ) ;
#15273=CARTESIAN_POINT ( 'NONE',  ( 4.730628863548789710E-15, -17.36981209788766023, -9.068162680945121679 ) ) ;
#15275=CARTESIAN_POINT ( 'NONE',  ( -4.243569643750000786, -26.44909673908217584, -13.49174472062871999 ) ) ;
#15278=LINE ( 'NONE', #6821, #4418 ) ;
#15279=CARTESIAN_POINT ( 'NONE',  ( -4.000000000000004441, -22.75385437650777476, -4.188073799010446407 ) ) ;
#15280=CARTESIAN_POINT ( 'NONE',  ( -2.121784821874996396, -23.48169916855646733, -15.66109696253308314 ) ) ;
#15282=DIRECTION ( 'NONE',  ( 1.000000000000000000, 0.000000000000000000, 0.000000000000000000 ) ) ;
#15283=CARTESIAN_POINT ( 'NONE',  ( -4.000000000000000888, -21.98057781498731345, -7.110038326093152783 ) ) ;
#15286=LINE ( 'NONE', #2586, #1562 ) ;
#15287=EDGE_CURVE ( 'NONE', #14859, #10059, #12721, .T. ) ;
#15293=CARTESIAN_POINT ( 'NONE',  ( -2.121784821875005722, -28.41632039872075666, -9.893996101495421414 ) ) ;
#15295=ADVANCED_FACE ( 'NONE', ( #15301 ), #5897, .F. ) ;
#15297=CARTESIAN_POINT ( 'NONE',  ( -2.000000000000005773, -22.90389237762567021, -2.389191317703265316 ) ) ;
#15298=ORIENTED_EDGE ( 'NONE', *, *, #560, .T. ) ;
#15300=LINE ( 'NONE', #8049, #3467 ) ;
#15301=FACE_OUTER_BOUND ( 'NONE', #12034, .T. ) ;
#15302=CARTESIAN_POINT ( 'NONE',  ( -2.121784821874996396, -19.64232189773168358, -10.17789796607362618 ) ) ;
#15307=CARTESIAN_POINT ( 'NONE',  ( -1.999999999999996225, -22.02517348798640029, -13.21320440821394904 ) ) ;
#15314=CARTESIAN_POINT ( 'NONE',  ( -4.243569643750005227, -21.98179658260448832, -2.840288794994898058 ) ) ;
#15316=EDGE_CURVE ( 'NONE', #8682, #17004, #6505, .T. ) ;
#15318=CARTESIAN_POINT ( 'NONE',  ( -4.000000000000000888, -24.23903503241459845, -10.33544949947430425 ) ) ;
#15322=CARTESIAN_POINT ( 'NONE',  ( 1.743066579297358403E-15, -23.60804816792780159, -16.40809404916146264 ) ) ;
#15323=CARTESIAN_POINT ( 'NONE',  ( 4.243569643750003451, -20.67805750669377929, -9.521336655703983354 ) ) ;
#15325=EDGE_CURVE ( 'NONE', #6382, #3333, #13986, .T. ) ;
#15337=CARTESIAN_POINT ( 'NONE',  ( 2.121784821875004390, -21.71795162677701896, -13.14220442634442243 ) ) ;
#15342=CARTESIAN_POINT ( 'NONE',  ( -4.243569643750005227, -25.62759180616079746, -8.047023976506819665 ) ) ;
#15352=CARTESIAN_POINT ( 'NONE',  ( 4.243569643750003451, -20.16183871397784344, -8.784099815843886105 ) ) ;
#15353=CARTESIAN_POINT ( 'NONE',  ( 1.743066579297358403E-15, -23.60804816792780159, -16.40809404916146264 ) ) ;
#15359=CARTESIAN_POINT ( 'NONE',  ( -1.071796769724486564, -28.49508014663179623, -9.439924663463729715 ) ) ;
#15363=AXIS2_PLACEMENT_3D ( 'NONE', #1051, #12065, #10680 ) ;
#15365=CARTESIAN_POINT ( 'NONE',  ( -2.121784821875005722, -24.80278884970919506, -4.733338222474753998 ) ) ;
#15368=CARTESIAN_POINT ( 'NONE',  ( -2.121784821874996396, -23.48169916855646733, -15.66109696253308314 ) ) ;
#15369=CARTESIAN_POINT ( 'NONE',  ( -5.577813053751546416E-15, -24.87002189690140241, -4.262804949787145858 ) ) ;
#15373=CARTESIAN_POINT ( 'NONE',  ( 4.243569643749996345, -27.57416683702714622, -10.82702122681259205 ) ) ;
#15376=CARTESIAN_POINT ( 'NONE',  ( 3.999999999999996447, -23.50667344992347196, -5.263210858146513793 ) ) ;
#15379=CARTESIAN_POINT ( 'NONE',  ( -2.343145750507622527, 4.000000000000006217, 3.999999999999999112 ) ) ;
#15387=CARTESIAN_POINT ( 'NONE',  ( -4.243569643750000786, -25.19081343183707844, -11.69472992346973861 ) ) ;
#15389=CARTESIAN_POINT ( 'NONE',  ( -3.999999999999997335, -17.98093379758235955, -5.424272602036731783 ) ) ;
#15390=ORIENTED_EDGE ( 'NONE', *, *, #6928, .T. ) ;
#15393=CARTESIAN_POINT ( 'NONE',  ( -2.000000000000005773, -26.84006067278963670, -8.010622222643258183 ) ) ;
#15395=CARTESIAN_POINT ( 'NONE',  ( -8.500000000000005329, 0.000000000000000000, 20.49999999999999645 ) ) ;
#15397=CARTESIAN_POINT ( 'NONE',  ( 4.730628863548789710E-15, -19.43468726875141073, -12.01711004038550001 ) ) ;
#15401=CARTESIAN_POINT ( 'NONE',  ( 3.579096709490575479E-14, -26.48320562484364871, -6.566670075356708658 ) ) ;
#15403=ORIENTED_EDGE ( 'NONE', *, *, #6483, .F. ) ;
#15404=CARTESIAN_POINT ( 'NONE',  ( 4.000000000000000888, -24.94883587310395967, -11.34915015528869731 ) ) ;
#15405=CARTESIAN_POINT ( 'NONE',  ( 0.000000000000000000, 5.977523610840987267, 32.81826849749789687 ) ) ;
#15407=CARTESIAN_POINT ( 'NONE',  ( 0.000000000000000000, 10.00000000000000000, 0.000000000000000000 ) ) ;
#15408=ORIENTED_EDGE ( 'NONE', *, *, #10323, .T. ) ;
#15411=CARTESIAN_POINT ( 'NONE',  ( 3.999999999999996447, -27.37831439529299615, -10.79248715709723072 ) ) ;
#15414=CARTESIAN_POINT ( 'NONE',  ( -1.999999999999996225, -22.47686493090789739, -13.85828664208477079 ) ) ;
#15417=CARTESIAN_POINT ( 'NONE',  ( -4.243569643750005227, -22.01406025714923231, -2.886366097486154469 ) ) ;
#15420=CARTESIAN_POINT ( 'NONE',  ( -4.243569643750000786, -23.35178398278655010, -9.068323681468148934 ) ) ;
#15425=ORIENTED_EDGE ( 'NONE', *, *, #1321, .T. ) ;
#15426=EDGE_LOOP ( 'NONE', ( #6840, #962, #17856, #16956 ) ) ;
#15433=CARTESIAN_POINT ( 'NONE',  ( -4.243569643750000786, -23.35178398278655010, -9.068323681468148934 ) ) ;
#15438=B_SPLINE_CURVE_WITH_KNOTS ( 'NONE', 3,
 ( #16184, #7911, #3480, #3661, #9393, #13566, #9126, #4952 ),
 .UNSPECIFIED., .F., .F.,
 ( 4, 2, 2, 4 ),
 ( 0.02025600316476611554, 0.02089043502514349032, 0.02152486688552086164, 0.02279373060627560774 ),
 .UNSPECIFIED. ) ;
#15439=CARTESIAN_POINT ( 'NONE',  ( -4.243569643750000786, -23.38404765733129764, -9.114400983959404456 ) ) ;
#15443=CARTESIAN_POINT ( 'NONE',  ( 4.299564228933482956E-15, -17.73605940148895854, -8.022024996759636650 ) ) ;
#15444=CARTESIAN_POINT ( 'NONE',  ( 4.730628863548789710E-15, -18.36998600877478438, -10.49655905817405355 ) ) ;
#15445=FACE_BOUND ( 'NONE', #1142, .T. ) ;
#15448=CYLINDRICAL_SURFACE ( 'NONE', #12382, 4.000000000000000000 ) ;
#15452=CARTESIAN_POINT ( 'NONE',  ( -8.999999999999996447, -4.000000000000000000, 30.00000000000000000 ) ) ;
#15455=CARTESIAN_POINT ( 'NONE',  ( -2.121784821874996396, -18.86799370865777803, -9.072042706283481195 ) ) ;
#15460=CARTESIAN_POINT ( 'NONE',  ( -4.243569643749998122, -24.97988077932658157, -15.66497698787144799 ) ) ;
#15463=CARTESIAN_POINT ( 'NONE',  ( -5.577813053751546416E-15, -25.64435008597530796, -5.368660209577289955 ) ) ;
#15465=CARTESIAN_POINT ( 'NONE',  ( -5.577813053751546416E-15, -29.32240898478130120, -10.62147269458723464 ) ) ;
#15466=CARTESIAN_POINT ( 'NONE',  ( 4.730628863548789710E-15, -22.75784574686025152, -16.76307219698486506 ) ) ;
#15468=CARTESIAN_POINT ( 'NONE',  ( -1.999999999999996225, -20.67009915640211659, -11.27795770257443841 ) ) ;
#15469=CARTESIAN_POINT ( 'NONE',  ( -2.000000000000005773, -24.25896670920994680, -4.324438023342780824 ) ) ;
#15471=ORIENTED_EDGE ( 'NONE', *, *, #14075, .T. ) ;
#15472=DIRECTION ( 'NONE',  ( 0.000000000000000000, 0.8191520442889952403, -0.5735764363510413855 ) ) ;
#15473=VECTOR ( 'NONE', #5959, 1000.000000000000000 ) ;
#15476=CARTESIAN_POINT ( 'NONE',  ( 1.071796769724485454, -20.26415271599303836, -11.63251642472675229 ) ) ;
#15479=CARTESIAN_POINT ( 'NONE',  ( -2.121784821875005722, -27.90010160600482081, -9.156759261635325942 ) ) ;
#15484=DIRECTION ( 'NONE',  ( 0.000000000000000000, 0.000000000000000000, 1.000000000000000000 ) ) ;
#15487=CARTESIAN_POINT ( 'NONE',  ( -2.121784821874996396, -19.12610310501574418, -9.440661126213528931 ) ) ;
#15488=ORIENTED_EDGE ( 'NONE', *, *, #14795, .T. ) ;
#15491=CARTESIAN_POINT ( 'NONE',  ( -3.999999999999997335, -22.43332088546226188, -11.78294034683682057 ) ) ;
#15493=DIRECTION ( 'NONE',  ( 0.000000000000000000, 0.000000000000000000, 1.000000000000000000 ) ) ;
#15496=CARTESIAN_POINT ( 'NONE',  ( 1.999999999999994449, -29.63624580000097097, -12.00398843855210629 ) ) ;
#15501=CARTESIAN_POINT ( 'NONE',  ( 3.999999999999996447, -25.24891187463481046, -7.751385191667569785 ) ) ;
#15502=( BOUNDED_CURVE ( )  B_SPLINE_CURVE ( 2, ( #10120, #14698, #17491, #7439, #17394, #14508, #217, #10503, #4660 ),
 .UNSPECIFIED., .F., .T. ) 
 B_SPLINE_CURVE_WITH_KNOTS ( ( 3, 2, 2, 2, 3 ),
 ( 0.8534482758620689502, 0.8563218390804597790, 0.8620689655172413257, 0.8678160919540229834, 0.8706896551724138122 ),
 .UNSPECIFIED. ) 
 CURVE ( )  GEOMETRIC_REPRESENTATION_ITEM ( )  RATIONAL_B_SPLINE_CURVE ( ( 0.9330127018922194093, 0.9330127018922194093, 1.000000000000000000, 0.8660254037844387076, 1.000000000000000000, 0.8660254037844387076, 1.000000000000000000, 0.9330127018922194093, 0.9330127018922194093 ) ) 
 REPRESENTATION_ITEM ( '' )  );
#15506=CARTESIAN_POINT ( 'NONE',  ( -2.121784821874996396, -19.86816761954490573, -10.50043908351241662 ) ) ;
#15507=DIRECTION ( 'NONE',  ( 0.8191520442889960174, 0.4698463103929512164, -0.3289899283371594541 ) ) ;
#15508=CARTESIAN_POINT ( 'NONE',  ( 4.000000000000000888, -21.01266757793999318, -5.727719250348704882 ) ) ;
#15510=ORIENTED_EDGE ( 'NONE', *, *, #16558, .F. ) ;
#15513=CARTESIAN_POINT ( 'NONE',  ( 4.898587196589413815E-16, 2.700915433685006750, 35.11257424290206330 ) ) ;
#15516=ORIENTED_EDGE ( 'NONE', *, *, #10205, .T. ) ;
#15518=CARTESIAN_POINT ( 'NONE',  ( 4.243569643750003451, -20.41994811033581314, -9.152718235773933841 ) ) ;
#15522=CARTESIAN_POINT ( 'NONE',  ( 0.000000000000000000, -15.45745613286697839, -10.86990606519494129 ) ) ;
#15524=CARTESIAN_POINT ( 'NONE',  ( -4.243569643750000786, -23.64215705368926379, -9.483019403889452192 ) ) ;
#15526=CARTESIAN_POINT ( 'NONE',  ( -1.598251304517731564, -15.40332308709088061, -10.50456014341368416 ) ) ;
#15528=CARTESIAN_POINT ( 'NONE',  ( -1.071796769724496334, -24.17174775834076073, -3.265566130642198139 ) ) ;
#15529=CARTESIAN_POINT ( 'NONE',  ( 4.243569643750000786, -20.38352592466991808, -4.829211852272596417 ) ) ;
#15535=DIRECTION ( 'NONE',  ( -0.000000000000000000, -0.5735764363510414965, -0.8191520442889950182 ) ) ;
#15538=CARTESIAN_POINT ( 'NONE',  ( 4.730628863548789710E-15, -16.59548390881375468, -7.962307421154977582 ) ) ;
#15542=CARTESIAN_POINT ( 'NONE',  ( 4.243569643749997233, -27.83227623338511236, -11.19563964674263978 ) ) ;
#15545=DIRECTION ( 'NONE',  ( -0.000000000000000000, 1.000000000000000000, -0.000000000000000000 ) ) ;
#15546=CARTESIAN_POINT ( 'NONE',  ( 4.243569643749996345, -26.54172925159527452, -9.352547547092401103 ) ) ;
#15547=EDGE_CURVE ( 'NONE', #451, #11984, #4604, .T. ) ;
#15550=CARTESIAN_POINT ( 'NONE',  ( 4.000000000000000888, -19.78664794594458698, -3.976781756687743918 ) ) ;
#15552=EDGE_CURVE ( 'NONE', #7377, #2690, #1754, .T. ) ;
#15554=CARTESIAN_POINT ( 'NONE',  ( -1.661723472263481630E-14, -20.57526276142661459, -12.07682761599016175 ) ) ;
#15555=CARTESIAN_POINT ( 'NONE',  ( 2.000000000000004441, -20.45500799277048287, -10.97077568596606056 ) ) ;
#15558=CARTESIAN_POINT ( 'NONE',  ( 4.730628863548789710E-15, -20.72523425054125212, -13.86020214003574047 ) ) ;
#15562=CYLINDRICAL_SURFACE ( 'NONE', #4620, 2.000000000000001776 ) ;
#15564=CARTESIAN_POINT ( 'NONE',  ( -4.243569643749997233, -20.62428471578586553, -9.444541151551892000 ) ) ;
#15567=ADVANCED_FACE ( 'NONE', ( #12949 ), #6188, .T. ) ;
#15568=VERTEX_POINT ( 'NONE', #5815 ) ;
#15569=CARTESIAN_POINT ( 'NONE',  ( 2.000000000000004441, -21.55197292799679687, -12.53740397167552878 ) ) ;
#15575=CARTESIAN_POINT ( 'NONE',  ( -5.279047395330986450E-15, -30.08741143020316144, -10.63516078049664948 ) ) ;
#15579=CARTESIAN_POINT ( 'NONE',  ( 4.713407268011036227E-15, -20.26195175892625855, -12.70822176395157044 ) ) ;
#15583=CARTESIAN_POINT ( 'NONE',  ( -6.428571428571427937, -11.73421655796351892, 14.25837509840160067 ) ) ;
#15584=CARTESIAN_POINT ( 'NONE',  ( -5.330712181944246111E-15, -27.04303497500847797, -5.796996205112000311 ) ) ;
#15585=ADVANCED_FACE ( 'NONE', ( #7288 ), #259, .F. ) ;
#15586=CONICAL_SURFACE ( 'NONE', #794, 2.000000000000001776, 1.029744260000000189 ) ;
#15588=CARTESIAN_POINT ( 'NONE',  ( -1.071796769724496334, -20.30562666434980912, -11.69174736140419135 ) ) ;
#15591=EDGE_LOOP ( 'NONE', ( #352, #16266, #13809, #7142, #4230 ) ) ;
#15598=CARTESIAN_POINT ( 'NONE',  ( 2.121784821874994176, -26.01805392422797070, -6.468916616312057499 ) ) ;
#15600=( BOUNDED_CURVE ( )  B_SPLINE_CURVE ( 2, ( #8916, #3281, #1899, #16080, #7806, #17670, #13463, #9105, #10679 ),
 .UNSPECIFIED., .F., .T. ) 
 B_SPLINE_CURVE_WITH_KNOTS ( ( 3, 2, 2, 2, 3 ),
 ( 0.9224137931034482873, 0.9252873563218391162, 0.9310344827586206629, 0.9367816091954023205, 0.9396551724137931494 ),
 .UNSPECIFIED. ) 
 CURVE ( )  GEOMETRIC_REPRESENTATION_ITEM ( )  RATIONAL_B_SPLINE_CURVE ( ( 0.9330127018922194093, 0.9330127018922194093, 1.000000000000000000, 0.8660254037844387076, 1.000000000000000000, 0.8660254037844387076, 1.000000000000000000, 0.9330127018922180770, 0.9330127018922194093 ) ) 
 REPRESENTATION_ITEM ( '' )  );
#15604=CARTESIAN_POINT ( 'NONE',  ( 4.730628863548789710E-15, -18.40224968331953548, -10.54263636066531085 ) ) ;
#15605=DIRECTION ( 'NONE',  ( 1.000000000000000000, 0.000000000000000000, 0.000000000000000000 ) ) ;
#15609=CARTESIAN_POINT ( 'NONE',  ( 4.243569643750000786, -20.12541652831194838, -4.460593432342547793 ) ) ;
#15610=EDGE_CURVE ( 'NONE', #10059, #3027, #3322, .T. ) ;
#15611=CARTESIAN_POINT ( 'NONE',  ( -1.661723472263481630E-14, -21.34959095050052014, -13.18268287578030318 ) ) ;
#15613=EDGE_LOOP ( 'NONE', ( #8308, #13603, #10081 ) ) ;
#15616=CARTESIAN_POINT ( 'NONE',  ( -2.121784821875005722, -29.93271310232382021, -12.05962931858445231 ) ) ;
#15619=FACE_OUTER_BOUND ( 'NONE', #12436, .T. ) ;
#15620=CARTESIAN_POINT ( 'NONE',  ( 9.000000000000005329, -10.00000000000000000, -30.00000000000000000 ) ) ;
#15621=ORIENTED_EDGE ( 'NONE', *, *, #337, .T. ) ;
#15622=CARTESIAN_POINT ( 'NONE',  ( -2.121784821875005722, -23.25413247156138397, -2.521627702894468470 ) ) ;
#15624=AXIS2_PLACEMENT_3D ( 'NONE', #8680, #17350, #8499 ) ;
#15625=CIRCLE ( 'NONE', #7618, 2.000000000000001776 ) ;
#15626=( BOUNDED_CURVE ( )  B_SPLINE_CURVE ( 2, ( #3846, #6711, #12363, #5330, #13002, #2827, #1708, #123, #15611 ),
 .UNSPECIFIED., .F., .F. ) 
 B_SPLINE_CURVE_WITH_KNOTS ( ( 3, 2, 2, 2, 3 ),
 ( 0.3017241379310345306, 0.3045977011494253039, 0.3103448275862069061, 0.3160919540229885083, 0.3189655172413793371 ),
 .UNSPECIFIED. ) 
 CURVE ( )  GEOMETRIC_REPRESENTATION_ITEM ( )  RATIONAL_B_SPLINE_CURVE ( ( 0.9330127018922194093, 0.9330127018922200755, 1.000000000000000000, 0.8660254037844387076, 1.000000000000000000, 0.8660254037844387076, 1.000000000000000000, 0.9330127018922187432, 0.9330127018922194093 ) ) 
 REPRESENTATION_ITEM ( '' )  );
#15628=CARTESIAN_POINT ( 'NONE',  ( 4.730628863548789710E-15, -21.72540816142837983, -15.28859851726467589 ) ) ;
#15633=CARTESIAN_POINT ( 'NONE',  ( 4.243569643750000786, -24.25516687003944938, -10.35848815122331068 ) ) ;
#15635=CARTESIAN_POINT ( 'NONE',  ( 3.999999999999996447, -21.69990767541768761, -2.682881918636178753 ) ) ;
#15640=DIRECTION ( 'NONE',  ( 0.000000000000000000, 0.8191520442889952403, -0.5735764363510413855 ) ) ;
#15645=CARTESIAN_POINT ( 'NONE',  ( 4.730628863548789710E-15, -20.46712485418328242, -13.49158372010569096 ) ) ;
#15651=EDGE_CURVE ( 'NONE', #2970, #3053, #15934, .T. ) ;
#15653=CARTESIAN_POINT ( 'NONE',  ( 0.000000000000000000, 5.977523610840987267, 32.81826849749789687 ) ) ;
#15655=CARTESIAN_POINT ( 'NONE',  ( -5.330712181944245322E-15, -25.01042347868947857, -2.894126148162874834 ) ) ;
#15659=ORIENTED_EDGE ( 'NONE', *, *, #14847, .F. ) ;
#15660=CARTESIAN_POINT ( 'NONE',  ( -1.999999999999996225, -17.63731374990092959, -6.946691269403138413 ) ) ;
#15667=ORIENTED_EDGE ( 'NONE', *, *, #3201, .T. ) ;
#15668=B_SPLINE_CURVE_WITH_KNOTS ( 'NONE', 3,
 ( #1463, #12759, #14247, #12931 ),
 .UNSPECIFIED., .F., .F.,
 ( 4, 4 ),
 ( 0.002451451260336424184, 0.003462474391252139301 ),
 .UNSPECIFIED. ) ;
#15670=CARTESIAN_POINT ( 'NONE',  ( 4.000000000000003553, -21.16428301933063949, -9.970566447840647939 ) ) ;
#15672=EDGE_CURVE ( 'NONE', #10774, #8639, #10499, .T. ) ;
#15674=CARTESIAN_POINT ( 'NONE',  ( 4.000000000000000888, -20.81908553137646578, -5.451255436407934418 ) ) ;
#15676=EDGE_CURVE ( 'NONE', #18119, #12399, #12988, .T. ) ;
#15679=ADVANCED_FACE ( 'NONE', ( #17149 ), #16809, .F. ) ;
#15681=CARTESIAN_POINT ( 'NONE',  ( -2.121784821875005722, -26.31918155331226217, -6.898971439563784003 ) ) ;
#15683=CARTESIAN_POINT ( 'NONE',  ( -5.577813053751546416E-15, -23.32136551875358776, -2.051094430206859887 ) ) ;
#15685=ORIENTED_EDGE ( 'NONE', *, *, #3781, .T. ) ;
#15691=CARTESIAN_POINT ( 'NONE',  ( -4.243569643750005227, -25.07910933890011407, -7.263709834155468670 ) ) ;
#15697=CARTESIAN_POINT ( 'NONE',  ( 4.243569643750003451, -21.22653997395446623, -10.30465079805533435 ) ) ;
#15698=CARTESIAN_POINT ( 'NONE',  ( -6.079313232897520791, -14.44302855110153594, -4.023496914806315772 ) ) ;
#15699=AXIS2_PLACEMENT_3D ( 'NONE', #10454, #10356, #7484 ) ;
#15700=CARTESIAN_POINT ( 'NONE',  ( 0.000000000000000000, 5.977523610840987267, 32.81826849749789687 ) ) ;
#15702=( BOUNDED_CURVE ( )  B_SPLINE_CURVE ( 2, ( #6018, #14474, #2799, #8429, #15674, #12697, #14093, #5655, #9999 ),
 .UNSPECIFIED., .F., .T. ) 
 B_SPLINE_CURVE_WITH_KNOTS ( ( 3, 2, 2, 2, 3 ),
 ( 0.8189655172413793371, 0.8218390804597701660, 0.8275862068965517127, 0.8333333333333333703, 0.8362068965517241992 ),
 .UNSPECIFIED. ) 
 CURVE ( )  GEOMETRIC_REPRESENTATION_ITEM ( )  RATIONAL_B_SPLINE_CURVE ( ( 0.9330127018922194093, 0.9330127018922194093, 1.000000000000000000, 0.8660254037844387076, 1.000000000000000000, 0.8660254037844387076, 1.000000000000000000, 0.9330127018922180770, 0.9330127018922194093 ) ) 
 REPRESENTATION_ITEM ( '' )  );
#15703=CARTESIAN_POINT ( 'NONE',  ( -2.121784821874996396, -17.28707365596521939, -6.814254884211938368 ) ) ;
#15704=CARTESIAN_POINT ( 'NONE',  ( 8.500000000000019540, 0.000000000000000000, -18.49999999999998934 ) ) ;
#15706=ORIENTED_EDGE ( 'NONE', *, *, #7265, .T. ) ;
#15708=CARTESIAN_POINT ( 'NONE',  ( -4.000000000000004441, -24.04440135829761616, -6.031165898660685976 ) ) ;
#15711=DIRECTION ( 'NONE',  ( -0.000000000000000000, -0.5735764363510414965, -0.8191520442889950182 ) ) ;
#15713=CARTESIAN_POINT ( 'NONE',  ( -4.243569643750004339, -22.01406025714923587, -2.886366097486154469 ) ) ;
#15716=CARTESIAN_POINT ( 'NONE',  ( 4.243569643750000786, -26.61041511180591357, -13.72213123308499760 ) ) ;
#15719=CARTESIAN_POINT ( 'NONE',  ( 4.243569643750000786, -25.02949505911335137, -11.46434341101345389 ) ) ;
#15720=CARTESIAN_POINT ( 'NONE',  ( 8.500000000000019540, 0.000000000000000000, 22.49999999999999289 ) ) ;
#15722=CARTESIAN_POINT ( 'NONE',  ( 1.533898589781675205E-14, -27.77375260663349366, -8.409762175006950002 ) ) ;
#15724=CARTESIAN_POINT ( 'NONE',  ( 4.243569643750003451, -23.00104207391549593, -12.83890243507441120 ) ) ;
#15726=CARTESIAN_POINT ( 'NONE',  ( 4.000000000000003553, -18.64771640554539545, -6.376536854529448739 ) ) ;
#15727=VECTOR ( 'NONE', #3749, 1000.000000000000000 ) ;
#15733=CARTESIAN_POINT ( 'NONE',  ( 0.000000000000000000, 9.254131787996968228, 30.52396275209373044 ) ) ;
#15735=( BOUNDED_CURVE ( )  B_SPLINE_CURVE ( 2, ( #869, #18222, #17941, #11052, #9294, #6691, #6516, #3917, #10777 ),
 .UNSPECIFIED., .F., .F. ) 
 B_SPLINE_CURVE_WITH_KNOTS ( ( 3, 2, 2, 2, 3 ),
 ( 0.7155172413793103869, 0.7183908045977011048, 0.7241379310344827624, 0.7298850574712644201, 0.7327586206896552490 ),
 .UNSPECIFIED. ) 
 CURVE ( )  GEOMETRIC_REPRESENTATION_ITEM ( )  RATIONAL_B_SPLINE_CURVE ( ( 0.9330127018922194093, 0.9330127018922206306, 1.000000000000000000, 0.8660254037844387076, 1.000000000000000000, 0.8660254037844387076, 1.000000000000000000, 0.9330127018922180770, 0.9330127018922194093 ) ) 
 REPRESENTATION_ITEM ( '' )  );
#15737=CARTESIAN_POINT ( 'NONE',  ( 2.121784821875004390, -21.49210590496380036, -12.81966330890563022 ) ) ;
#15743=CARTESIAN_POINT ( 'NONE',  ( 4.299564228933482956E-15, -19.47829782620029704, -10.51019933028069708 ) ) ;
#15744=DIRECTION ( 'NONE',  ( 0.000000000000000000, 0.000000000000000000, 1.000000000000000000 ) ) ;
#15747=CARTESIAN_POINT ( 'NONE',  ( -2.121784821875005722, -24.28657005699325921, -3.996101382614658970 ) ) ;
#15748=ORIENTED_EDGE ( 'NONE', *, *, #3864, .T. ) ;
#15750=CARTESIAN_POINT ( 'NONE',  ( 3.999999999999996447, -24.99080247827684431, -7.382766771737522049 ) ) ;
#15752=ORIENTED_EDGE ( 'NONE', *, *, #3565, .T. ) ;
#15753=LINE ( 'NONE', #14174, #10758 ) ;
#15754=CARTESIAN_POINT ( 'NONE',  ( -3.706921591972381904E-14, -17.67153205169451624, -7.929870390770359379 ) ) ;
#15761=CARTESIAN_POINT ( 'NONE',  ( 4.000000000000000888, -23.07754274880374368, -8.676666609789087659 ) ) ;
#15764=CYLINDRICAL_SURFACE ( 'NONE', #11475, 4.000000000000000000 ) ;
#15767=CARTESIAN_POINT ( 'NONE',  ( -6.616789018075169615, -14.16315581186571571, -2.134625489590734837 ) ) ;
#15768=CARTESIAN_POINT ( 'NONE',  ( -2.121784821874996396, -18.57762063775506078, -8.657346983862177936 ) ) ;
#15771=VERTEX_POINT ( 'NONE', #15007 ) ;
#15772=ORIENTED_EDGE ( 'NONE', *, *, #14377, .T. ) ;
#15774=CARTESIAN_POINT ( 'NONE',  ( -4.000000000000004441, -25.07683894372948785, -7.505639578380876031 ) ) ;
#15778=CARTESIAN_POINT ( 'NONE',  ( 1.999999999999994449, -23.95783908012565888, -3.894383200091054320 ) ) ;
#15779=ORIENTED_EDGE ( 'NONE', *, *, #16928, .F. ) ;
#15782=EDGE_CURVE ( 'NONE', #94, #5846, #13096, .T. ) ;
#15784=CARTESIAN_POINT ( 'NONE',  ( 4.243569643749996345, -25.25118226980542602, -7.509455447442161535 ) ) ;
#15787=EDGE_CURVE ( 'NONE', #8354, #8879, #18252, .T. ) ;
#15792=CARTESIAN_POINT ( 'NONE',  ( 4.243569643749996345, -24.50911775527627157, -6.449677490143276515 ) ) ;
#15793=DIRECTION ( 'NONE',  ( -0.000000000000000000, -0.000000000000000000, -1.000000000000000000 ) ) ;
#15800=CARTESIAN_POINT ( 'NONE',  ( 4.243569643750003451, -18.87129173218799849, -6.941007716193646537 ) ) ;
#15804=CARTESIAN_POINT ( 'NONE',  ( 4.730628863548789710E-15, -23.01595514321822122, -17.13169061691491279 ) ) ;
#15808=CARTESIAN_POINT ( 'NONE',  ( -9.974462289245280999, -9.920488278021490913, 4.137459934542836670 ) ) ;
#15810=EDGE_LOOP ( 'NONE', ( #11523, #1570, #17819, #83 ) ) ;
#15811=CARTESIAN_POINT ( 'NONE',  ( 2.121784821874994176, -22.69489544611912279, -1.722954459712693787 ) ) ;
#15813=CARTESIAN_POINT ( 'NONE',  ( 4.713407268011036227E-15, -16.13220141719875400, -6.810327045070806662 ) ) ;
#15814=DIRECTION ( 'NONE',  ( -0.000000000000000000, -0.5735764363510414965, -0.8191520442889950182 ) ) ;
#15815=CARTESIAN_POINT ( 'NONE',  ( 4.243569643750003451, -23.00104207391549593, -12.83890243507440942 ) ) ;
#15816=( BOUNDED_CURVE ( )  B_SPLINE_CURVE ( 2, ( #8815, #5769, #17016, #1515, #14212, #4468, #7148, #7331, #2995 ),
 .UNSPECIFIED., .F., .F. ) 
 B_SPLINE_CURVE_WITH_KNOTS ( ( 3, 2, 2, 2, 3 ),
 ( 0.2672413793103448620, 0.2701149425287356354, 0.2758620689655172376, 0.2816091954022988397, 0.2844827586206896686 ),
 .UNSPECIFIED. ) 
 CURVE ( )  GEOMETRIC_REPRESENTATION_ITEM ( )  RATIONAL_B_SPLINE_CURVE ( ( 0.9330127018922194093, 0.9330127018922200755, 1.000000000000000000, 0.8660254037844387076, 1.000000000000000000, 0.8660254037844387076, 1.000000000000000000, 0.9330127018922187432, 0.9330127018922194093 ) ) 
 REPRESENTATION_ITEM ( '' )  );
#15817=CYLINDRICAL_SURFACE ( 'NONE', #11733, 4.000000000000000000 ) ;
#15821=CARTESIAN_POINT ( 'NONE',  ( -4.243569643750000786, -24.38422156821842535, -10.54279736118833988 ) ) ;
#15822=CARTESIAN_POINT ( 'NONE',  ( 0.000000000000000000, 9.254131787996968228, 30.52396275209373044 ) ) ;
#15823=CARTESIAN_POINT ( 'NONE',  ( 3.999999999999996447, -22.47423586449159671, -3.788737178426322849 ) ) ;
#15829=CARTESIAN_POINT ( 'NONE',  ( 3.375445829055900404, -25.20600189401019264, -15.83707978931157534 ) ) ;
#15832=CARTESIAN_POINT ( 'NONE',  ( -4.243569643750004339, -25.62759180616079746, -8.047023976506819665 ) ) ;
#15834=ORIENTED_EDGE ( 'NONE', *, *, #12879, .T. ) ;
#15837=CARTESIAN_POINT ( 'NONE',  ( 2.121784821875004390, -22.00832469767973620, -13.55690014876572569 ) ) ;
#15840=CARTESIAN_POINT ( 'NONE',  ( 4.000000000000003553, -20.64806422661470720, -9.233329607980554243 ) ) ;
#15841=CARTESIAN_POINT ( 'NONE',  ( 4.243569643749996345, -23.99289896256033572, -5.712440650283179266 ) ) ;
#15842=ORIENTED_EDGE ( 'NONE', *, *, #6941, .F. ) ;
#15856=EDGE_CURVE ( 'NONE', #18310, #14557, #16921, .T. ) ;
#15857=CARTESIAN_POINT ( 'NONE',  ( -4.000000000000000888, -23.98092563605662875, -9.966831079544254735 ) ) ;
#15858=ORIENTED_EDGE ( 'NONE', *, *, #12314, .T. ) ;
#15861=CARTESIAN_POINT ( 'NONE',  ( -10.00496734058828174, -9.915240373983317923, 7.344972601042156768 ) ) ;
#15862=CARTESIAN_POINT ( 'NONE',  ( -5.330712181944246111E-15, -26.01059738957659917, -4.322522525391808479 ) ) ;
#15866=ORIENTED_EDGE ( 'NONE', *, *, #13795, .T. ) ;
#15867=VERTEX_POINT ( 'NONE', #9783 ) ;
#15872=CARTESIAN_POINT ( 'NONE',  ( -3.706921591972381904E-14, -17.47795000513098884, -7.653406576829588026 ) ) ;
#15873=CARTESIAN_POINT ( 'NONE',  ( 4.000000000000003553, -22.97104879383642384, -12.55089538735098387 ) ) ;
#15876=CARTESIAN_POINT ( 'NONE',  ( -4.243569643750000786, -21.54501820828076930, -6.487994741957813005 ) ) ;
#15879=CARTESIAN_POINT ( 'NONE',  ( -5.330712181944246111E-15, -30.94693959492275681, -11.37234980655397187 ) ) ;
#15882=CARTESIAN_POINT ( 'NONE',  ( 2.121784821875004390, -20.20155892317395541, -10.97657120925539154 ) ) ;
#15883=CARTESIAN_POINT ( 'NONE',  ( -7.496011132626526852, -13.00850824371983272, 4.993358875981036782 ) ) ;
#15886=CARTESIAN_POINT ( 'NONE',  ( -7.951672694476823011, -10.00000000000000178, -6.265341990738099831 ) ) ;
#15890=ORIENTED_EDGE ( 'NONE', *, *, #16149, .T. ) ;
#15891=CARTESIAN_POINT ( 'NONE',  ( -5.330712181944245322E-15, -24.72005040778675777, -2.479430425741570243 ) ) ;
#15894=ORIENTED_EDGE ( 'NONE', *, *, #9101, .T. ) ;
#15897=CARTESIAN_POINT ( 'NONE',  ( 4.243569643749996345, -28.86471381881699116, -12.67011332646282895 ) ) ;
#15899=CARTESIAN_POINT ( 'NONE',  ( 0.000000000000000000, 9.254131787996968228, 30.52396275209373044 ) ) ;
#15903=CARTESIAN_POINT ( 'NONE',  ( -2.121784821875005722, -29.96497677686856775, -12.10570662107570961 ) ) ;
#15904=EDGE_CURVE ( 'NONE', #10307, #16888, #16579, .T. ) ;
#15905=EDGE_CURVE ( 'NONE', #13681, #10807, #2925, .T. ) ;
#15907=EDGE_CURVE ( 'NONE', #18076, #14905, #15278, .T. ) ;
#15909=CARTESIAN_POINT ( 'NONE',  ( 4.243569643750000786, -26.32004204090319632, -13.30743551066369257 ) ) ;
#15910=CARTESIAN_POINT ( 'NONE',  ( -1.999999999999996225, -21.76706409162843059, -12.84458598828390130 ) ) ;
#15912=CARTESIAN_POINT ( 'NONE',  ( -5.330712181944245322E-15, -28.33358195679831937, -7.640088304762238103 ) ) ;
#15913=CARTESIAN_POINT ( 'NONE',  ( -5.577813053751546416E-15, -25.19265864305380376, -4.723577975706471754 ) ) ;
#15914=CARTESIAN_POINT ( 'NONE',  ( 4.713407268011036227E-15, -16.19672876699319630, -6.902481651060079493 ) ) ;
#15916=ORIENTED_EDGE ( 'NONE', *, *, #1176, .T. ) ;
#15918=CARTESIAN_POINT ( 'NONE',  ( 4.000000000000003553, -22.00313855819898379, -11.16857631362007020 ) ) ;
#15921=CARTESIAN_POINT ( 'NONE',  ( -5.279047395330986450E-15, -29.82930203384519530, -10.26654236056660352 ) ) ;
#15925=ORIENTED_EDGE ( 'NONE', *, *, #10393, .T. ) ;
#15926=CARTESIAN_POINT ( 'NONE',  ( 4.243569643750003451, -21.48464937031243238, -10.67326921798538031 ) ) ;
#15929=CARTESIAN_POINT ( 'NONE',  ( 4.000000000000003553, -19.61562664118283195, -7.758855928260365076 ) ) ;
#15931=CARTESIAN_POINT ( 'NONE',  ( 2.121784821874994176, -28.37330216599443489, -9.832559698173744422 ) ) ;
#15934=LINE ( 'NONE', #3232, #2077 ) ;
#15937=CARTESIAN_POINT ( 'NONE',  ( -5.330712181944245322E-15, -25.78475166776338412, -3.999981407953017598 ) ) ;
#15938=ORIENTED_EDGE ( 'NONE', *, *, #16603, .F. ) ;
#15939=CARTESIAN_POINT ( 'NONE',  ( 1.999999999999994449, -22.40918270197784778, -1.682672680510768792 ) ) ;
#15943=EDGE_LOOP ( 'NONE', ( #16607, #3293, #3259, #15046, #6030, #499, #4936, #11105, #3401, #5075, #7536, #12100, #16447, #1906, #3070, #657, #10702, #4302, #1477, #576, #11870, #4323, #13584, #3680, #10863, #5193, #16565, #11486, #1848, #6407, #7893, #9115, #16774, #13837, #14964, #14975, #4528, #12220, #1472, #4982, #819, #5074, #2211, #5215, #3445, #18135, #5486, #3819, #2226, #8116, #1827, #1097, #14091, #12645, #13424, #6926, #3247, #2156, #10911, #13243, #2026, #1316, #7945 ) ) ;
#15944=ORIENTED_EDGE ( 'NONE', *, *, #13056, .F. ) ;
#15945=CARTESIAN_POINT ( 'NONE',  ( 8.500000000000019540, 10.00000000000000000, 20.49999999999998934 ) ) ;
#15951=AXIS2_PLACEMENT_3D ( 'NONE', #8921, #316, #6051 ) ;
#15953=VECTOR ( 'NONE', #2882, 1000.000000000000000 ) ;
#15955=CARTESIAN_POINT ( 'NONE',  ( 2.000000000000004441, -18.90635161462267178, -8.759065166385774148 ) ) ;
#15960=CARTESIAN_POINT ( 'NONE',  ( -9.175662590029975973, -10.00000000000000000, -2.949107115053327011 ) ) ;
#15961=CARTESIAN_POINT ( 'NONE',  ( 4.243569643750000786, -21.41596351010179333, -6.303685531992786473 ) ) ;
#15965=CARTESIAN_POINT ( 'NONE',  ( 4.243569643750000786, -27.09437022997710187, -14.41329077045383578 ) ) ;
#15966=VERTEX_POINT ( 'NONE', #17126 ) ;
#15970=CARTESIAN_POINT ( 'NONE',  ( 3.579096709490575479E-14, -25.70887743576973605, -5.460814815566567226 ) ) ;
#15975=CARTESIAN_POINT ( 'NONE',  ( -4.243569643750005227, -23.01423416803636002, -4.314762474715088558 ) ) ;
#15979=CARTESIAN_POINT ( 'NONE',  ( -2.000000000000005773, -29.35662728657488429, -11.60465181595445650 ) ) ;
#15980=CONICAL_SURFACE ( 'NONE', #8539, 2.000000000000001776, 1.029744260000000189 ) ;
#15981=CARTESIAN_POINT ( 'NONE',  ( 4.243569643750000786, -22.48066477007841613, -7.824236514204232940 ) ) ;
#15983=CARTESIAN_POINT ( 'NONE',  ( -7.506644857339464849, -12.68590315496589938, 7.157248747909027209 ) ) ;
#15984=EDGE_CURVE ( 'NONE', #12418, #11008, #4584, .T. ) ;
#15987=VECTOR ( 'NONE', #15265, 1000.000000000000000 ) ;
#15989=VERTEX_POINT ( 'NONE', #12923 ) ;
#15991=CARTESIAN_POINT ( 'NONE',  ( 1.071796769724490339, -22.32902788685678885, -14.58146378416713773 ) ) ;
#15992=( LENGTH_UNIT ( ) NAMED_UNIT ( * ) SI_UNIT ( .MILLI., .METRE. ) );
#15994=VECTOR ( 'NONE', #542, 1000.000000000000000 ) ;
#15996=CARTESIAN_POINT ( 'NONE',  ( 4.243569643750003451, -23.25915147027346563, -13.20752085500445894 ) ) ;
#16002=CARTESIAN_POINT ( 'NONE',  ( 4.243569643749996345, -28.12264930428783671, -11.61033536916394304 ) ) ;
#16004=CARTESIAN_POINT ( 'NONE',  ( -2.000000000000005773, -27.87249825822150839, -9.485095902363450904 ) ) ;
#16005=CARTESIAN_POINT ( 'NONE',  ( -4.243569643750000786, -23.60989337914451625, -9.436942101398194893 ) ) ;
#16009=CARTESIAN_POINT ( 'NONE',  ( 4.243569643750003451, -21.96860448848362779, -11.36442875535422026 ) ) ;
#16015=CARTESIAN_POINT ( 'NONE',  ( 1.533898589781675205E-14, -26.99942441755958811, -7.303906915216807683 ) ) ;
#16018=CARTESIAN_POINT ( 'NONE',  ( 4.000000000000003553, -24.06801372906273428, -14.11752367306045208 ) ) ;
#16019=DIRECTION ( 'NONE',  ( 8.673617379884034239E-17, 0.000000000000000000, 1.000000000000000000 ) ) ;
#16023=CARTESIAN_POINT ( 'NONE',  ( -4.243569643749998122, -21.39861290485976753, -10.55039641134203521 ) ) ;
#16030=CARTESIAN_POINT ( 'NONE',  ( 4.243569643749996345, -27.09021171885596146, -10.13586168944375210 ) ) ;
#16031=CYLINDRICAL_SURFACE ( 'NONE', #6980, 4.000000000000000000 ) ;
#16033=CARTESIAN_POINT ( 'NONE',  ( 4.243569643750003451, -19.41977419944868544, -7.724321858545000197 ) ) ;
#16035=ORIENTED_EDGE ( 'NONE', *, *, #11981, .F. ) ;
#16036=CARTESIAN_POINT ( 'NONE',  ( 3.064181913176683203, -21.66367673124435100, -2.174801284911689336 ) ) ;
#16038=CARTESIAN_POINT ( 'NONE',  ( 4.000000000000003553, -23.29368553998882518, -13.01166841327030710 ) ) ;
#16039=VERTEX_POINT ( 'NONE', #4308 ) ;
#16041=DIRECTION ( 'NONE',  ( -0.000000000000000000, -0.5735764363510414965, -0.8191520442889950182 ) ) ;
#16051=CARTESIAN_POINT ( 'NONE',  ( -4.000000000000000888, -21.91605046519287825, -7.017883720103874623 ) ) ;
#16053=DIRECTION ( 'NONE',  ( -0.000000000000000000, -0.5735764363510414965, -0.8191520442889950182 ) ) ;
#16056=CARTESIAN_POINT ( 'NONE',  ( -2.121784821875005722, -24.51241577880647782, -4.318642500053448963 ) ) ;
#16059=DIRECTION ( 'NONE',  ( 0.000000000000000000, 0.5150380737757255245, 0.8571673013836856869 ) ) ;
#16060=ORIENTED_EDGE ( 'NONE', *, *, #15325, .F. ) ;
#16062=CARTESIAN_POINT ( 'NONE',  ( -1.999999999999996225, -17.05656760739055500, -6.117299823553768334 ) ) ;
#16065=VERTEX_POINT ( 'NONE', #15722 ) ;
#16068=CARTESIAN_POINT ( 'NONE',  ( 4.243569643750003451, -19.38751052490393434, -7.678244556053742897 ) ) ;
#16073=CARTESIAN_POINT ( 'NONE',  ( -2.121784821875005722, -29.70686738051060161, -11.73708820114566009 ) ) ;
#16074=CARTESIAN_POINT ( 'NONE',  ( -4.000000000000000888, -26.04580080692037569, -12.91577843898463840 ) ) ;
#16076=CARTESIAN_POINT ( 'NONE',  ( -4.243569643750005227, -23.56271663529704696, -5.098076617066438665 ) ) ;
#16077=LINE ( 'NONE', #13089, #12461 ) ;
#16078=CARTESIAN_POINT ( 'NONE',  ( -3.412954772041501439, -15.19080604886724473, -9.070274817126582789 ) ) ;
#16080=CARTESIAN_POINT ( 'NONE',  ( 3.999999999999996447, -22.15159911833919182, -3.327964152506997397 ) ) ;
#16082=CARTESIAN_POINT ( 'NONE',  ( 1.533898589781675205E-14, -27.96733465319702105, -8.686225988947720467 ) ) ;
#16083=ORIENTED_EDGE ( 'NONE', *, *, #7600, .F. ) ;
#16085=CARTESIAN_POINT ( 'NONE',  ( -1.071796769724477238, -22.88120077655093354, -1.422474030991951688 ) ) ;
#16086=CARTESIAN_POINT ( 'NONE',  ( 3.999999999999996447, -27.57189644185653066, -11.06895097103799941 ) ) ;
#16092=CARTESIAN_POINT ( 'NONE',  ( -4.243569643750005227, -27.14398450976385746, -10.21265719359585233 ) ) ;
#16094=VECTOR ( 'NONE', #2514, 1000.000000000000000 ) ;
#16097=CARTESIAN_POINT ( 'NONE',  ( 5.002737418183710538, -14.83391033323059993, -6.661572473864424637 ) ) ;
#16098=CIRCLE ( 'NONE', #16386, 7.500000000000000888 ) ;
#16099=CARTESIAN_POINT ( 'NONE',  ( 2.121784821874994176, -28.63141156235240459, -10.20117811810379216 ) ) ;
#16100=( BOUNDED_CURVE ( )  B_SPLINE_CURVE ( 2, ( #17562, #10482, #10193, #14487, #14579, #15873, #12982, #3077, #1883 ),
 .UNSPECIFIED., .F., .T. ) 
 B_SPLINE_CURVE_WITH_KNOTS ( ( 3, 2, 2, 2, 3 ),
 ( 0.3017241379310345306, 0.3045977011494253039, 0.3103448275862069061, 0.3160919540229885083, 0.3189655172413793371 ),
 .UNSPECIFIED. ) 
 CURVE ( )  GEOMETRIC_REPRESENTATION_ITEM ( )  RATIONAL_B_SPLINE_CURVE ( ( 0.9330127018922194093, 0.9330127018922200755, 1.000000000000000000, 0.8660254037844387076, 1.000000000000000000, 0.8660254037844387076, 1.000000000000000000, 0.9330127018922187432, 0.9330127018922194093 ) ) 
 REPRESENTATION_ITEM ( '' )  );
#16101=CARTESIAN_POINT ( 'NONE',  ( -1.071796769724486564, -27.46264256119991742, -7.965450983743535218 ) ) ;
#16102=CARTESIAN_POINT ( 'NONE',  ( 4.243569643750000786, -24.51327626639741553, -10.72710657115335842 ) ) ;
#16103=LINE ( 'NONE', #2011, #13017 ) ;
#16105=CARTESIAN_POINT ( 'NONE',  ( 4.243569643750003451, -20.67805750669378284, -9.521336655703981577 ) ) ;
#16113=CARTESIAN_POINT ( 'NONE',  ( 1.999999999999994449, -28.08758942185315988, -9.792277918971819872 ) ) ;
#16117=CARTESIAN_POINT ( 'NONE',  ( 4.243569643750000786, -22.73877416643638227, -8.192854934134281564 ) ) ;
#16124=CARTESIAN_POINT ( 'NONE',  ( 4.243569643749996345, -28.12264930428783671, -11.61033536916394304 ) ) ;
#16125=DIRECTION ( 'NONE',  ( -0.000000000000000000, -0.000000000000000000, -1.000000000000000000 ) ) ;
#16126=CARTESIAN_POINT ( 'NONE',  ( 7.191589934391299899, -10.00000000000000000, 14.52136967842654158 ) ) ;
#16128=AXIS2_PLACEMENT_3D ( 'NONE', #18162, #10719, #13496 ) ;
#16130=CARTESIAN_POINT ( 'NONE',  ( -2.121784821875005722, -22.99602307520341427, -2.153009282964420290 ) ) ;
#16132=DIRECTION ( 'NONE',  ( 6.162975822039154730E-33, -0.5735764363510414965, -0.8191520442889950182 ) ) ;
#16133=CARTESIAN_POINT ( 'NONE',  ( -4.000000000000000888, -23.52923419313512454, -9.321748845673438311 ) ) ;
#16137=CARTESIAN_POINT ( 'NONE',  ( 2.000000000000004441, -21.29386353163882717, -12.16878555174548104 ) ) ;
#16145=CARTESIAN_POINT ( 'NONE',  ( -1.999999999999996225, -19.63766157097024490, -9.803484022854247470 ) ) ;
#16148=CARTESIAN_POINT ( 'NONE',  ( -1.661723472263481630E-14, -20.51073541163217584, -11.98467301000088803 ) ) ;
#16149=EDGE_CURVE ( 'NONE', #7195, #16065, #6112, .T. ) ;
#16150=CARTESIAN_POINT ( 'NONE',  ( 2.121784821875004390, -17.84631068140748766, -7.612928127393706390 ) ) ;
#16151=ADVANCED_FACE ( 'NONE', ( #7266 ), #235, .F. ) ;
#16152=CARTESIAN_POINT ( 'NONE',  ( 4.243569643750000786, -24.28743054458419692, -10.40456545371456620 ) ) ;
#16154=ORIENTED_EDGE ( 'NONE', *, *, #11437, .F. ) ;
#16155=CARTESIAN_POINT ( 'NONE',  ( 1.801903668194569486, -10.00000000000000178, 23.81845480839541196 ) ) ;
#16160=CARTESIAN_POINT ( 'NONE',  ( 4.730628863548789710E-15, -18.11187661241681823, -10.12794063824400581 ) ) ;
#16164=CARTESIAN_POINT ( 'NONE',  ( -1.999999999999996225, -24.02552130905571204, -16.06999716166505721 ) ) ;
#16165=CARTESIAN_POINT ( 'NONE',  ( 4.243569643750003451, -19.41977419944868544, -7.724321858545000197 ) ) ;
#16166=CARTESIAN_POINT ( 'NONE',  ( 0.000000000000000000, 5.977523610840987267, 32.81826849749789687 ) ) ;
#16169=CARTESIAN_POINT ( 'NONE',  ( -5.577813053751546416E-15, -29.06429958842333505, -10.25285427465718691 ) ) ;
#16176=CARTESIAN_POINT ( 'NONE',  ( 2.121784821874994176, -28.59914788780765704, -10.15510081561253664 ) ) ;
#16178=VECTOR ( 'NONE', #3973, 1000.000000000000000 ) ;
#16179=CARTESIAN_POINT ( 'NONE',  ( -0.2979626678802195783, -10.00000000000000355, -4.943697222985274919 ) ) ;
#16180=CARTESIAN_POINT ( 'NONE',  ( 2.121784821875004390, -23.04076228311161145, -15.03137382848591663 ) ) ;
#16182=EDGE_CURVE ( 'NONE', #218, #2069, #8003, .T. ) ;
#16183=CARTESIAN_POINT ( 'NONE',  ( -4.243569643749998122, -22.65689621210486138, -12.34741120850101836 ) ) ;
#16184=CARTESIAN_POINT ( 'NONE',  ( 3.375445829055900404, -25.20600189401019264, -15.83707978931157534 ) ) ;
#16188=CARTESIAN_POINT ( 'NONE',  ( 3.579096709490575479E-14, -23.64400226490599266, -2.511867456126184894 ) ) ;
#16190=CARTESIAN_POINT ( 'NONE',  ( 4.243569643750000786, -23.22272928460757413, -8.884014471503119736 ) ) ;
#16191=B_SPLINE_CURVE_WITH_KNOTS ( 'NONE', 3,
 ( #2748, #2833, #16941, #8380, #9861, #14042, #6983, #15808, #18335, #12644, #7350, #2919, #7166, #223 ),
 .UNSPECIFIED., .F., .F.,
 ( 4, 2, 2, 2, 2, 2, 4 ),
 ( 0.000000000000000000, 0.002373381915594256590, 0.004746763831188513180, 0.007120145746782769770, 0.009493527662377028095, 0.01424029149356554128, 0.01898705532475405272 ),
 .UNSPECIFIED. ) ;
#16193=DIRECTION ( 'NONE',  ( 0.000000000000000000, 0.8191520442889952403, -0.5735764363510413855 ) ) ;
#16194=CARTESIAN_POINT ( 'NONE',  ( 1.533898589781675205E-14, -27.70922525683905846, -8.317607569017670954 ) ) ;
#16196=ORIENTED_EDGE ( 'NONE', *, *, #950, .F. ) ;
#16198=CARTESIAN_POINT ( 'NONE',  ( -4.000000000000004441, -25.65758508623986245, -8.335031024230248775 ) ) ;
#16200=CARTESIAN_POINT ( 'NONE',  ( 1.071796769724495224, -16.97325791313388521, -6.932631571625408995 ) ) ;
#16202=( BOUNDED_CURVE ( )  B_SPLINE_CURVE ( 1, ( #8998, #10187 ),
 .UNSPECIFIED., .F., .T. ) 
 B_SPLINE_CURVE_WITH_KNOTS ( ( 2, 2 ),
 ( 0.000000000000000000, 1.000000000000000000 ),
 .UNSPECIFIED. ) 
 CURVE ( )  GEOMETRIC_REPRESENTATION_ITEM ( )  RATIONAL_B_SPLINE_CURVE ( ( 0.9401542295229485813, 0.9401542295229485813 ) ) 
 REPRESENTATION_ITEM ( '' )  );
#16204=CARTESIAN_POINT ( 'NONE',  ( -4.243569643749998122, -21.14050350850180138, -10.18177799141198747 ) ) ;
#16210=CARTESIAN_POINT ( 'NONE',  ( 2.121784821875004390, -23.04076228311161145, -15.03137382848591663 ) ) ;
#16211=CARTESIAN_POINT ( 'NONE',  ( 4.299564228933482956E-15, -23.34993877156982833, -16.03947562923141135 ) ) ;
#16212=CARTESIAN_POINT ( 'NONE',  ( 6.268704630795123300, -10.34422234558816633, 0.7521107233528409042 ) ) ;
#16213=CARTESIAN_POINT ( 'NONE',  ( -1.071796769724496334, -21.78975569270318502, -13.81130327499520760 ) ) ;
#16214=CARTESIAN_POINT ( 'NONE',  ( 4.243569643749996345, -22.44424258441252817, -3.500730130702893739 ) ) ;
#16216=CARTESIAN_POINT ( 'NONE',  ( 3.999999999999996447, -25.05532982807127951, -7.474921377726801097 ) ) ;
#16217=CARTESIAN_POINT ( 'NONE',  ( 4.000000000000003553, -21.48691976548304794, -10.43133947375997295 ) ) ;
#16218=VERTEX_POINT ( 'NONE', #17688 ) ;
#16221=CARTESIAN_POINT ( 'NONE',  ( -3.706921591972381904E-14, -18.18775084441045209, -8.667107230630458403 ) ) ;
#16222=CARTESIAN_POINT ( 'NONE',  ( 0.000000000000000000, 5.977523610840987267, 32.81826849749789687 ) ) ;
#16227=ORIENTED_EDGE ( 'NONE', *, *, #10346, .T. ) ;
#16229=CARTESIAN_POINT ( 'NONE',  ( -4.000000000000000888, -22.43226925790881765, -7.755120559963970983 ) ) ;
#16234=CARTESIAN_POINT ( 'NONE',  ( 4.898587196589413815E-16, 2.700915433685006750, 35.11257424290206330 ) ) ;
#16238=CARTESIAN_POINT ( 'NONE',  ( -4.243569643749998122, -18.52714587037736749, -6.449516489620252813 ) ) ;
#16239=CARTESIAN_POINT ( 'NONE',  ( 4.243569643750000786, -23.77121175186825752, -9.667328613854474284 ) ) ;
#16241=ORIENTED_EDGE ( 'NONE', *, *, #7835, .F. ) ;
#16242=CARTESIAN_POINT ( 'NONE',  ( -1.522508701837280043, -9.999999999999175770, 22.87631747054243903 ) ) ;
#16245=CARTESIAN_POINT ( 'NONE',  ( 4.243569643750000786, -26.61041511180591357, -13.72213123308499760 ) ) ;
#16251=CARTESIAN_POINT ( 'NONE',  ( -5.330712181944245322E-15, -25.23626920050269362, -3.216667265601666603 ) ) ;
#16255=CARTESIAN_POINT ( 'NONE',  ( 4.243569643750000786, -26.86852450816387972, -14.09074965301504534 ) ) ;
#16256=ADVANCED_FACE ( 'NONE', ( #17784 ), #13917, .T. ) ;
#16257=CARTESIAN_POINT ( 'NONE',  ( 4.713407268011036227E-15, -22.32682692979000549, -15.65716912339195233 ) ) ;
#16258=EDGE_CURVE ( 'NONE', #10807, #7842, #11793, .T. ) ;
#16259=CARTESIAN_POINT ( 'NONE',  ( -4.243569643749997233, -19.07562833763805088, -7.232830631971606472 ) ) ;
#16261=EDGE_CURVE ( 'NONE', #4334, #177, #17868, .T. ) ;
#16263=DIRECTION ( 'NONE',  ( -0.000000000000000000, -0.5735764363510414965, -0.8191520442889950182 ) ) ;
#16266=ORIENTED_EDGE ( 'NONE', *, *, #8614, .T. ) ;
#16268=LINE ( 'NONE', #6423, #3521 ) ;
#16270=CARTESIAN_POINT ( 'NONE',  ( 4.000000000000000888, -25.91674610874139972, -12.73146922901961098 ) ) ;
#16273=CARTESIAN_POINT ( 'NONE',  ( 2.121784821874994176, -29.11536668052359289, -10.89233765547263211 ) ) ;
#16280=CARTESIAN_POINT ( 'NONE',  ( 2.121784821875004390, -22.26643409403770590, -13.92551856869577342 ) ) ;
#16282=LINE ( 'NONE', #16560, #12032 ) ;
#16286=CARTESIAN_POINT ( 'NONE',  ( 4.243569643750003451, -21.45238569576768484, -10.62719191549412656 ) ) ;
#16291=DIRECTION ( 'NONE',  ( -0.000000000000000000, -0.5735764363510414965, -0.8191520442889950182 ) ) ;
#16295=CARTESIAN_POINT ( 'NONE',  ( 4.000000000000003553, -18.38960700918742219, -6.007918434599401003 ) ) ;
#16297=CARTESIAN_POINT ( 'NONE',  ( 4.243569643749997233, -24.25100835891830542, -6.081059070213227891 ) ) ;
#16301=EDGE_CURVE ( 'NONE', #11633, #10059, #7913, .T. ) ;
#16302=DIRECTION ( 'NONE',  ( 0.000000000000000000, 0.000000000000000000, 1.000000000000000000 ) ) ;
#16304=CARTESIAN_POINT ( 'NONE',  ( -3.537377991931545118, -25.46155756473516263, -15.53479600987054532 ) ) ;
#16306=CARTESIAN_POINT ( 'NONE',  ( 9.909030972036948270, -9.930865375757933933, 8.916665252758585680 ) ) ;
#16308=CARTESIAN_POINT ( 'NONE',  ( -5.330712181944245322E-15, -23.71987649689963362, -1.051034048512634156 ) ) ;
#16311=CARTESIAN_POINT ( 'NONE',  ( 2.000000000000004441, -19.74520715349101607, -9.957075032165194628 ) ) ;
#16315=( BOUNDED_CURVE ( )  B_SPLINE_CURVE ( 2, ( #3093, #9016, #4474, #5863, #14312, #1611, #11696, #11885, #16082 ),
 .UNSPECIFIED., .F., .T. ) 
 B_SPLINE_CURVE_WITH_KNOTS ( ( 3, 2, 2, 2, 3 ),
 ( 0.3189655172413793371, 0.3218390804597701105, 0.3275862068965517127, 0.3333333333333333148, 0.3362068965517241437 ),
 .UNSPECIFIED. ) 
 CURVE ( )  GEOMETRIC_REPRESENTATION_ITEM ( )  RATIONAL_B_SPLINE_CURVE ( ( 0.9330127018922194093, 0.9330127018922200755, 1.000000000000000000, 0.8660254037844387076, 1.000000000000000000, 0.8660254037844387076, 1.000000000000000000, 0.9330127018922187432, 0.9330127018922194093 ) ) 
 REPRESENTATION_ITEM ( '' )  );
#16322=EDGE_CURVE ( 'NONE', #9296, #218, #16103, .T. ) ;
#16323=CARTESIAN_POINT ( 'NONE',  ( -2.000000000000005773, -25.22687694484738685, -5.706757097073694496 ) ) ;
#16326=CARTESIAN_POINT ( 'NONE',  ( 0.000000000000000000, 5.977523610840987267, 32.81826849749789687 ) ) ;
#16329=CARTESIAN_POINT ( 'NONE',  ( -5.330712181944246111E-15, -23.68761282235488252, -1.004956746021377967 ) ) ;
#16330=CARTESIAN_POINT ( 'NONE',  ( -2.121784821875005722, -27.12577341693091171, -8.050904001845182734 ) ) ;
#16331=CARTESIAN_POINT ( 'NONE',  ( -3.706921591972381904E-14, -19.73640722255826319, -10.87881775021074127 ) ) ;
#16332=ORIENTED_EDGE ( 'NONE', *, *, #7503, .F. ) ;
#16333=CARTESIAN_POINT ( 'NONE',  ( 6.428571428571431490, -11.73421655796352248, 14.25837509840157757 ) ) ;
#16335=CARTESIAN_POINT ( 'NONE',  ( 4.243569643750000786, -26.86852450816387972, -14.09074965301504534 ) ) ;
#16336=ORIENTED_EDGE ( 'NONE', *, *, #3559, .T. ) ;
#16339=CARTESIAN_POINT ( 'NONE',  ( -4.243569643750005227, -22.75612477167838676, -3.946144054785039490 ) ) ;
#16342=( BOUNDED_CURVE ( )  B_SPLINE_CURVE ( 2, ( #2543, #13836, #17008, #18308, #9747, #7319, #2894, #7140, #194 ),
 .UNSPECIFIED., .F., .F. ) 
 B_SPLINE_CURVE_WITH_KNOTS ( ( 3, 2, 2, 2, 3 ),
 ( 0.3534482758620690057, 0.3563218390804597790, 0.3620689655172413812, 0.3678160919540229834, 0.3706896551724138122 ),
 .UNSPECIFIED. ) 
 CURVE ( )  GEOMETRIC_REPRESENTATION_ITEM ( )  RATIONAL_B_SPLINE_CURVE ( ( 0.9330127018922194093, 0.9330127018922200755, 1.000000000000000000, 0.8660254037844387076, 1.000000000000000000, 0.8660254037844387076, 1.000000000000000000, 0.9330127018922187432, 0.9330127018922194093 ) ) 
 REPRESENTATION_ITEM ( '' )  );
#16343=CARTESIAN_POINT ( 'NONE',  ( 4.000000000000003553, -25.03592396470017434, -15.49984274679136576 ) ) ;
#16345=CARTESIAN_POINT ( 'NONE',  ( -2.121784821874996396, -18.09366551958387248, -7.966187446493337987 ) ) ;
#16351=CARTESIAN_POINT ( 'NONE',  ( -2.694913683823400241, -15.45745613286698372, -10.86990606519495373 ) ) ;
#16352=ADVANCED_FACE ( 'NONE', ( #18233 ), #6802, .F. ) ;
#16355=VERTEX_POINT ( 'NONE', #1159 ) ;
#16357=AXIS2_PLACEMENT_3D ( 'NONE', #15405, #4068, #6938 ) ;
#16358=CARTESIAN_POINT ( 'NONE',  ( 2.000000000000004441, -17.87391402919079653, -7.284591486665584981 ) ) ;
#16361=ORIENTED_EDGE ( 'NONE', *, *, #13512, .T. ) ;
#16364=( NAMED_UNIT ( * ) SI_UNIT ( $, .STERADIAN. ) SOLID_ANGLE_UNIT ( ) );
#16365=CARTESIAN_POINT ( 'NONE',  ( 2.121784821875004390, -23.26660800492483006, -15.35391494592470885 ) ) ;
#16369=CARTESIAN_POINT ( 'NONE',  ( 0.000000000000000000, 5.977523610840987267, 32.81826849749789687 ) ) ;
#16371=CARTESIAN_POINT ( 'NONE',  ( -2.121784821874996396, -22.48152525766933962, -14.23270058530414950 ) ) ;
#16374=DIRECTION ( 'NONE',  ( 0.000000000000000000, 0.8191520442889952403, -0.5735764363510413855 ) ) ;
#16376=CARTESIAN_POINT ( 'NONE',  ( -2.465190328815646976E-33, -26.97786251599082519, -14.24690051095425858 ) ) ;
#16378=CARTESIAN_POINT ( 'NONE',  ( -4.243569643750005227, -25.07910933890011407, -7.263709834155468670 ) ) ;
#16385=CARTESIAN_POINT ( 'NONE',  ( 1.533898589781675205E-14, -28.48355344591296401, -9.423462828807814162 ) ) ;
#16386=AXIS2_PLACEMENT_3D ( 'NONE', #5941, #12556, #12891 ) ;
#16390=CARTESIAN_POINT ( 'NONE',  ( 4.243569643750000786, -23.25499295915232167, -8.930091773994377036 ) ) ;
#16392=VERTEX_POINT ( 'NONE', #12452 ) ;
#16396=CARTESIAN_POINT ( 'NONE',  ( 0.4841626239896907880, -23.78953207011253923, -16.78102399689576174 ) ) ;
#16400=CARTESIAN_POINT ( 'NONE',  ( 2.000000000000004441, -21.74555497456032427, -12.81386778561629924 ) ) ;
#16401=CARTESIAN_POINT ( 'NONE',  ( -2.121784821874996396, -17.06122793415199723, -6.491713766773147931 ) ) ;
#16402=ORIENTED_EDGE ( 'NONE', *, *, #8455, .F. ) ;
#16403=CARTESIAN_POINT ( 'NONE',  ( 4.299564228933482956E-15, -19.80093457235270549, -10.97097235620001854 ) ) ;
#16404=CARTESIAN_POINT ( 'NONE',  ( -5.279047395330986450E-15, -26.73198927754956600, -5.843121321406028912 ) ) ;
#16413=AXIS2_PLACEMENT_3D ( 'NONE', #16369, #3653, #7905 ) ;
#16416=CARTESIAN_POINT ( 'NONE',  ( -4.000000000000000888, -20.88361287976100300, -5.543410040383684567 ) ) ;
#16417=ORIENTED_EDGE ( 'NONE', *, *, #7137, .T. ) ;
#16418=CARTESIAN_POINT ( 'NONE',  ( -1.999999999999996225, -18.86333338189633579, -8.697628763064102486 ) ) ;
#16421=CARTESIAN_POINT ( 'NONE',  ( 4.000000000000000888, -23.85187093787765278, -9.782521869579230867 ) ) ;
#16422=CARTESIAN_POINT ( 'NONE',  ( -4.243569643750000786, -19.73825243377498850, -3.907665802447479297 ) ) ;
#16423=( BOUNDED_CURVE ( )  B_SPLINE_CURVE ( 3, ( #10011, #17088, #1879, #4458 ),
 .UNSPECIFIED., .F., .F. ) 
 B_SPLINE_CURVE_WITH_KNOTS ( ( 4, 4 ),
 ( -8.881784197001252323E-16, 1.570796326794896558 ),
 .UNSPECIFIED. ) 
 CURVE ( )  GEOMETRIC_REPRESENTATION_ITEM ( )  RATIONAL_B_SPLINE_CURVE ( ( 1.000000000000000000, 0.8047378541243648264, 0.8047378541243648264, 1.000000000000000000 ) ) 
 REPRESENTATION_ITEM ( '' )  );
#16424=CARTESIAN_POINT ( 'NONE',  ( 4.243569643749996345, -26.83210232249799532, -9.767243269513704362 ) ) ;
#16425=PRODUCT ( 'Brass Valve Body', 'Brass Valve Body', '', ( #9231 ) ) ;
#16426=CARTESIAN_POINT ( 'NONE',  ( -2.195159659341646030, -29.79542698874031714, -12.39207419899238083 ) ) ;
#16429=CARTESIAN_POINT ( 'NONE',  ( -4.253155871621290274, -10.96494312749350364, 19.45022984308078406 ) ) ;
#16432=CARTESIAN_POINT ( 'NONE',  ( -5.330712181944245322E-15, -30.43072080220681386, -10.63511296669387818 ) ) ;
#16435=ADVANCED_FACE ( 'NONE', ( #3841 ), #3932, .T. ) ;
#16436=DIRECTION ( 'NONE',  ( -0.3258630558627198526, 0.000000000000000000, -0.9454169814551725004 ) ) ;
#16437=CARTESIAN_POINT ( 'NONE',  ( -5.330712181944245322E-15, -24.46194101142878807, -2.110812005811521619 ) ) ;
#16440=CARTESIAN_POINT ( 'NONE',  ( 4.713407268011036227E-15, -21.03627994800016054, -13.81407702374171365 ) ) ;
#16442=CARTESIAN_POINT ( 'NONE',  ( 4.243569643750003451, -18.64544601037477278, -6.618466598754856101 ) ) ;
#16447=ORIENTED_EDGE ( 'NONE', *, *, #4725, .F. ) ;
#16451=CARTESIAN_POINT ( 'NONE',  ( -5.577813053751546416E-15, -29.25788163498686245, -10.52931808859795559 ) ) ;
#16454=CARTESIAN_POINT ( 'NONE',  ( 4.243569643749996345, -25.76740106252136542, -8.246692287302257895 ) ) ;
#16457=FACE_OUTER_BOUND ( 'NONE', #712, .T. ) ;
#16459=CARTESIAN_POINT ( 'NONE',  ( 4.243569643749996345, -26.83210232249799532, -9.767243269513704362 ) ) ;
#16464=CARTESIAN_POINT ( 'NONE',  ( -2.121784821875005722, -24.77052517516444752, -4.687260919983497587 ) ) ;
#16466=ORIENTED_EDGE ( 'NONE', *, *, #6077, .T. ) ;
#16467=LINE ( 'NONE', #12090, #15727 ) ;
#16472=CARTESIAN_POINT ( 'NONE',  ( 1.071796769724504328, -23.82605761075068429, -2.771869435411045579 ) ) ;
#16480=CARTESIAN_POINT ( 'NONE',  ( -4.243569643750004339, -23.56271663529704696, -5.098076617066439553 ) ) ;
#16488=CARTESIAN_POINT ( 'NONE',  ( 1.761081750400359969, -24.08916239126616787, -16.59049792717877736 ) ) ;
#16489=CARTESIAN_POINT ( 'NONE',  ( 9.350658029750295697, -10.00000000000000178, 13.61865533257045691 ) ) ;
#16490=CARTESIAN_POINT ( 'NONE',  ( 4.150834101209824212, -27.15734369766470380, -14.50322620280942587 ) ) ;
#16491=CARTESIAN_POINT ( 'NONE',  ( 4.243569643750003451, -17.87111782130087434, -5.512611338964712893 ) ) ;
#16494=CARTESIAN_POINT ( 'NONE',  ( -4.000000000000004441, -25.14136629352392660, -7.597794184370155079 ) ) ;
#16497=EDGE_LOOP ( 'NONE', ( #13412, #7694 ) ) ;
#16501=CARTESIAN_POINT ( 'NONE',  ( 2.000000000000004441, -20.71311738912845257, -11.33939410589610652 ) ) ;
#16504=ORIENTED_EDGE ( 'NONE', *, *, #6702, .F. ) ;
#16506=CARTESIAN_POINT ( 'NONE',  ( 4.000000000000000888, -21.01266757793999318, -5.727719250348704882 ) ) ;
#16510=DIRECTION ( 'NONE',  ( -0.000000000000000000, -0.000000000000000000, -1.000000000000000000 ) ) ;
#16512=CARTESIAN_POINT ( 'NONE',  ( 2.121784821875004390, -16.81387309597561242, -6.138454447673516334 ) ) ;
#16513=VECTOR ( 'NONE', #8472, 1000.000000000000000 ) ;
#16514=CARTESIAN_POINT ( 'NONE',  ( -5.330712181944245322E-15, -28.62395502770104017, -8.054784027183542250 ) ) ;
#16519=DIRECTION ( 'NONE',  ( -1.000000000000000000, 0.000000000000000000, 0.000000000000000000 ) ) ;
#16520=CARTESIAN_POINT ( 'NONE',  ( 4.243569643750000786, -26.35230571544794387, -13.35351281315494987 ) ) ;
#16521=ORIENTED_EDGE ( 'NONE', *, *, #7835, .T. ) ;
#16524=CARTESIAN_POINT ( 'NONE',  ( 4.730628863548789710E-15, -15.78889204519509981, -6.810374858873577075 ) ) ;
#16529=CARTESIAN_POINT ( 'NONE',  ( -4.000000000000000888, -25.01336322148850044, -11.44130475926444745 ) ) ;
#16532=CARTESIAN_POINT ( 'NONE',  ( -3.999999999999997335, -23.72386786725210328, -13.62603244648705925 ) ) ;
#16534=( BOUNDED_CURVE ( )  B_SPLINE_CURVE ( 2, ( #7310, #6020, #17825, #13251, #16421, #5087, #3614, #570, #16148 ),
 .UNSPECIFIED., .F., .T. ) 
 B_SPLINE_CURVE_WITH_KNOTS ( ( 3, 2, 2, 2, 3 ),
 ( 0.4396551724137931494, 0.4425287356321839227, 0.4482758620689655249, 0.4540229885057471271, 0.4568965517241379559 ),
 .UNSPECIFIED. ) 
 CURVE ( )  GEOMETRIC_REPRESENTATION_ITEM ( )  RATIONAL_B_SPLINE_CURVE ( ( 0.9330127018922194093, 0.9330127018922200755, 1.000000000000000000, 0.8660254037844387076, 1.000000000000000000, 0.8660254037844387076, 1.000000000000000000, 0.9330127018922187432, 0.9330127018922194093 ) ) 
 REPRESENTATION_ITEM ( '' )  );
#16536=CARTESIAN_POINT ( 'NONE',  ( 4.730628863548789710E-15, -20.43486117963853133, -13.44550641761443543 ) ) ;
#16539=CARTESIAN_POINT ( 'NONE',  ( -6.158835246850665095E-15, -22.83371997885389604, -15.30223878937131587 ) ) ;
#16541=CYLINDRICAL_SURFACE ( 'NONE', #853, 4.000000000000000000 ) ;
#16544=VERTEX_POINT ( 'NONE', #9582 ) ;
#16548=CARTESIAN_POINT ( 'NONE',  ( 1.071796769724485454, -20.78037150870897065, -12.36975326458684954 ) ) ;
#16551=CARTESIAN_POINT ( 'NONE',  ( -4.243569643750000786, -24.90044036093436119, -11.28003420104843357 ) ) ;
#16557=CARTESIAN_POINT ( 'NONE',  ( -5.330712181944245322E-15, -27.84962683862713106, -6.948928767393398154 ) ) ;
#16558=EDGE_CURVE ( 'NONE', #1458, #3584, #13698, .T. ) ;
#16560=CARTESIAN_POINT ( 'NONE',  ( 4.898587196589413815E-16, 2.700915433685006750, 35.11257424290206330 ) ) ;
#16564=CARTESIAN_POINT ( 'NONE',  ( -2.121784821874996396, -18.31951124139709464, -8.288728563932130200 ) ) ;
#16565=ORIENTED_EDGE ( 'NONE', *, *, #207, .F. ) ;
#16566=CARTESIAN_POINT ( 'NONE',  ( 1.999999999999994449, -28.08758942185315988, -9.792277918971819872 ) ) ;
#16569=CARTESIAN_POINT ( 'NONE',  ( 4.000000000000003553, -18.58318905575096025, -6.284382248540171467 ) ) ;
#16573=CARTESIAN_POINT ( 'NONE',  ( -3.706921591972381904E-14, -18.18775084441045209, -8.667107230630458403 ) ) ;
#16576=CARTESIAN_POINT ( 'NONE',  ( -2.121784821874996396, -17.83555612322590278, -7.597569026563290251 ) ) ;
#16579=CIRCLE ( 'NONE', #9754, 6.000000000000000000 ) ;
#16581=CARTESIAN_POINT ( 'NONE',  ( -2.121784821874996396, -23.73980856491443703, -16.02971538246313443 ) ) ;
#16582=CARTESIAN_POINT ( 'NONE',  ( -1.071796769724486786, -19.20866172912349867, -10.12511907569473379 ) ) ;
#16584=CARTESIAN_POINT ( 'NONE',  ( 4.243569643750000786, -25.80382324818726048, -12.57019867080359710 ) ) ;
#16586=VERTEX_POINT ( 'NONE', #120 ) ;
#16588=CARTESIAN_POINT ( 'NONE',  ( -1.999999999999996225, -18.66975133533280484, -8.421164949123328469 ) ) ;
#16602=CARTESIAN_POINT ( 'NONE',  ( -4.243569643750000786, -25.96514162091098399, -12.80058518325988182 ) ) ;
#16603=EDGE_CURVE ( 'NONE', #13013, #5876, #4445, .T. ) ;
#16606=CARTESIAN_POINT ( 'NONE',  ( -4.000000000000000888, -20.62550348340303685, -5.174791620453635943 ) ) ;
#16607=ORIENTED_EDGE ( 'NONE', *, *, #16895, .F. ) ;
#16609=CARTESIAN_POINT ( 'NONE',  ( -3.999999999999997335, -22.17521148910429574, -11.41432192690677283 ) ) ;
#16611=CARTESIAN_POINT ( 'NONE',  ( 8.500000000000019540, 10.00000000000000000, -20.49999999999998934 ) ) ;
#16613=CARTESIAN_POINT ( 'NONE',  ( 4.243569643750003451, -18.09696354311409294, -5.835152456403505106 ) ) ;
#16614=CARTESIAN_POINT ( 'NONE',  ( 4.730628863548789710E-15, -18.14414028696156933, -10.17401794073526311 ) ) ;
#16618=CARTESIAN_POINT ( 'NONE',  ( 3.999999999999996447, -25.82965801714518506, -8.580776637516944305 ) ) ;
#16620=LINE ( 'NONE', #15035, #9262 ) ;
#16625=CARTESIAN_POINT ( 'NONE',  ( -4.000000000000004441, -28.75489784253548819, -12.75845206339082161 ) ) ;
#16630=CARTESIAN_POINT ( 'NONE',  ( 4.000000000000000888, -25.14241791966749417, -11.62561396922946777 ) ) ;
#16631=ORIENTED_EDGE ( 'NONE', *, *, #6702, .T. ) ;
#16632=CARTESIAN_POINT ( 'NONE',  ( -1.071796769724496334, -28.81771689278419757, -9.900697689383058275 ) ) ;
#16635=CARTESIAN_POINT ( 'NONE',  ( -5.330712181944246111E-15, -28.59169135315629617, -8.008706724692286727 ) ) ;
#16638=CARTESIAN_POINT ( 'NONE',  ( -3.706921591972381904E-14, -19.54282517599473579, -10.60235393626997080 ) ) ;
#16639=CARTESIAN_POINT ( 'NONE',  ( -1.071796769724477238, -26.49473232556249158, -6.583131910012619770 ) ) ;
#16641=ORIENTED_EDGE ( 'NONE', *, *, #4289, .T. ) ;
#16644=CARTESIAN_POINT ( 'NONE',  ( 1.071796769724494114, -23.42599282208309930, -16.14809206987660062 ) ) ;
#16645=CARTESIAN_POINT ( 'NONE',  ( 7.401749373187970882, -13.34905268700159020, 2.825469154945078554 ) ) ;
#16648=CARTESIAN_POINT ( 'NONE',  ( 2.121784821875004390, -20.94362343770310986, -12.03634916655427922 ) ) ;
#16652=DIRECTION ( 'NONE',  ( 0.000000000000000000, -0.5735764363510413855, -0.8191520442889951292 ) ) ;
#16653=CARTESIAN_POINT ( 'NONE',  ( 4.243569643750000786, -23.77121175186825752, -9.667328613854474284 ) ) ;
#16654=FACE_OUTER_BOUND ( 'NONE', #13027, .T. ) ;
#16657=DIRECTION ( 'NONE',  ( 0.000000000000000000, 0.000000000000000000, 1.000000000000000000 ) ) ;
#16658=CARTESIAN_POINT ( 'NONE',  ( 4.243569643750003451, -19.90372931761987019, -8.415481395913838369 ) ) ;
#16659=CARTESIAN_POINT ( 'NONE',  ( 0.000000000000000000, 5.977523610840987267, 32.81826849749789687 ) ) ;
#16662=EDGE_CURVE ( 'NONE', #9284, #177, #17520, .T. ) ;
#16668=CARTESIAN_POINT ( 'NONE',  ( -4.243569643749998122, -19.84995652671195643, -8.338685891761750568 ) ) ;
#16673=CARTESIAN_POINT ( 'NONE',  ( -4.016207988404787876, -26.68874843910498740, -14.64799399452802398 ) ) ;
#16674=CARTESIAN_POINT ( 'NONE',  ( 4.299564228933482956E-15, -23.09182937521185863, -15.67085720930136006 ) ) ;
#16675=CARTESIAN_POINT ( 'NONE',  ( -3.999999999999997335, -19.85222692188257554, -8.096756147536344983 ) ) ;
#16676=CARTESIAN_POINT ( 'NONE',  ( 2.121784821874994176, -29.37347607688156259, -11.26095607540267807 ) ) ;
#16677=ORIENTED_EDGE ( 'NONE', *, *, #10691, .T. ) ;
#16680=CARTESIAN_POINT ( 'NONE',  ( 3.999999999999996447, -22.99045465720752901, -4.525974018286417433 ) ) ;
#16684=CARTESIAN_POINT ( 'NONE',  ( -3.999999999999997335, -19.27148077937220449, -7.267364701686970463 ) ) ;
#16689=CARTESIAN_POINT ( 'NONE',  ( -5.330712181944246111E-15, -29.39828321677494216, -9.160639286973685458 ) ) ;
#16691=CARTESIAN_POINT ( 'NONE',  ( -2.000000000000005773, -23.16200177398363991, -2.757809737633313940 ) ) ;
#16702=CARTESIAN_POINT ( 'NONE',  ( -4.243569643750005227, -25.11137301344485451, -7.309787136646725081 ) ) ;
#16706=CARTESIAN_POINT ( 'NONE',  ( 4.713407268011036227E-15, -20.06836971236272760, -12.43175795001079642 ) ) ;
#16714=CARTESIAN_POINT ( 'NONE',  ( -4.243569643750005227, -22.23990597896245447, -3.208907214924944462 ) ) ;
#16716=ADVANCED_FACE ( 'NONE', ( #407 ), #10024, .F. ) ;
#16718=CARTESIAN_POINT ( 'NONE',  ( -4.000000000000000888, -25.52958201420443984, -12.17854159912454293 ) ) ;
#16719=VERTEX_POINT ( 'NONE', #2824 ) ;
#16721=CARTESIAN_POINT ( 'NONE',  ( 4.243569643750000786, -20.15768020285669593, -4.506670734833804204 ) ) ;
#16725=CARTESIAN_POINT ( 'NONE',  ( -2.121784821875005722, -25.28674396788038337, -5.424497759843593059 ) ) ;
#16726=CARTESIAN_POINT ( 'NONE',  ( -3.999999999999997335, -24.17555931017360393, -14.27111468035787922 ) ) ;
#16737=CARTESIAN_POINT ( 'NONE',  ( -4.243569643750005227, -26.88587511340589131, -9.844038773665802822 ) ) ;
#16744=CARTESIAN_POINT ( 'NONE',  ( -5.330712181944245322E-15, -28.36584563134306691, -7.686165607253494514 ) ) ;
#16747=APPLICATION_CONTEXT ( 'automotive_design' ) ;
#16750=CARTESIAN_POINT ( 'NONE',  ( -2.121784821874996396, -19.35194882682896633, -9.763202243652322920 ) ) ;
#16751=CARTESIAN_POINT ( 'NONE',  ( -3.706921591972381904E-14, -18.76849698692083379, -9.496498676479825818 ) ) ;
#16752=DIRECTION ( 'NONE',  ( -0.000000000000000000, 1.000000000000000000, -0.000000000000000000 ) ) ;
#16758=DIRECTION ( 'NONE',  ( -6.162975822039154730E-33, 0.5735764363510414965, 0.8191520442889950182 ) ) ;
#16760=CARTESIAN_POINT ( 'NONE',  ( 4.730628863548789710E-15, -17.11170270152969053, -8.699544261015072166 ) ) ;
#16765=CARTESIAN_POINT ( 'NONE',  ( 2.121784821875004390, -23.52471740128279620, -15.72253336585475658 ) ) ;
#16767=CARTESIAN_POINT ( 'NONE',  ( -3.999999999999997335, -20.56202776116204234, -9.110456801337205590 ) ) ;
#16768=CARTESIAN_POINT ( 'NONE',  ( -8.500000000000005329, 0.000000000000000000, 20.49999999999999645 ) ) ;
#16769=CARTESIAN_POINT ( 'NONE',  ( 4.730628863548789710E-15, -22.24162695414431212, -16.02583535712476959 ) ) ;
#16771=CARTESIAN_POINT ( 'NONE',  ( -4.000000000000004441, -25.33494834008745755, -7.874257998310924656 ) ) ;
#16772=CARTESIAN_POINT ( 'NONE',  ( -4.000000000000004441, -23.59270991537611550, -5.386083664789867775 ) ) ;
#16774=ORIENTED_EDGE ( 'NONE', *, *, #13088, .F. ) ;
#16782=CARTESIAN_POINT ( 'NONE',  ( 2.121784821874994176, -28.37330216599443489, -9.832559698173744422 ) ) ;
#16785=CARTESIAN_POINT ( 'NONE',  ( -4.243569643749997233, -24.23781626479742712, -14.60519903057256208 ) ) ;
#16786=EDGE_CURVE ( 'NONE', #5987, #10898, #5684, .T. ) ;
#16787=ORIENTED_EDGE ( 'NONE', *, *, #14842, .F. ) ;
#16790=DIRECTION ( 'NONE',  ( 0.000000000000000000, 0.8191520442889952403, -0.5735764363510413855 ) ) ;
#16792=DIRECTION ( 'NONE',  ( -0.000000000000000000, 1.000000000000000000, -0.000000000000000000 ) ) ;
#16793=CARTESIAN_POINT ( 'NONE',  ( -4.243569643749997233, -21.39861290485977463, -10.55039641134203521 ) ) ;
#16798=CARTESIAN_POINT ( 'NONE',  ( 1.999999999999994449, -27.82948002549519018, -9.423659499041770360 ) ) ;
#16804=CARTESIAN_POINT ( 'NONE',  ( -4.000000000000000888, -25.85221876035684474, -12.63931462504386793 ) ) ;
#16808=CARTESIAN_POINT ( 'NONE',  ( -3.999999999999997335, -22.62690293202579284, -12.05940416077758925 ) ) ;
#16809=( BOUNDED_SURFACE ( )  B_SPLINE_SURFACE ( 3, 2, ( 
 ( #3592, #16126, #10814 ),
 ( #16489, #8029, #4977 ),
 ( #17805, #10632, #2303 ),
 ( #7658, #815, #2128 ),
 ( #16306, #3416, #13417 ),
 ( #14927, #13686, #17627 ),
 ( #1003, #3767, #6643 ),
 ( #12201, #641, #7757 ),
 ( #4888, #7847, #12109 ),
 ( #6551, #2220, #17889 ),
 ( #5160, #6280, #2397 ),
 ( #6460, #16212, #731 ),
 ( #9418, #5067, #15095 ),
 ( #14736, #10537, #7936 ),
 ( #10722, #12291, #9152 ),
 ( #17981, #13594, #6374 ) ),
 .UNSPECIFIED., .F., .F., .T. ) 
 B_SPLINE_SURFACE_WITH_KNOTS ( ( 4, 2, 2, 2, 2, 2, 2, 4 ),
 ( 3, 3 ),
 ( 0.000000000000000000, 0.004776775202955720404, 0.007165162804433580605, 0.009553550405911440807, 0.01194193800738930014, 0.01433032560886716121, 0.01671871321034502228, 0.01910710081182288161 ),
 ( 0.000000000000000000, 1.000000000000000000 ),
 .UNSPECIFIED. ) 
 GEOMETRIC_REPRESENTATION_ITEM ( )  RATIONAL_B_SPLINE_SURFACE ( (
 ( 1.000000000000000000, 0.8431867568967624793, 1.000000000000000000),
 ( 1.000000000000000000, 0.8377920060143945191, 1.000000000000000000),
 ( 1.000000000000000000, 0.8290876956143414800, 1.000000000000000000),
 ( 1.000000000000000000, 0.8092161897602034859, 1.000000000000000000),
 ( 1.000000000000000000, 0.8014575563008032866, 1.000000000000000000),
 ( 1.000000000000000000, 0.7833253045188315333, 1.000000000000000000),
 ( 1.000000000000000000, 0.7729073097594592046, 1.000000000000000000),
 ( 1.000000000000000000, 0.7492617761142137400, 1.000000000000000000),
 ( 1.000000000000000000, 0.7360775662804031061, 1.000000000000000000),
 ( 1.000000000000000000, 0.7066113664073706557, 1.000000000000000000),
 ( 1.000000000000000000, 0.6903329448040008698, 1.000000000000000000),
 ( 1.000000000000000000, 0.6541098336270502189, 1.000000000000000000),
 ( 1.000000000000000000, 0.6341722888203963349, 1.000000000000000000),
 ( 1.000000000000000000, 0.5897142078662076514, 1.000000000000000000),
 ( 1.000000000000000000, 0.5651944592878379581, 1.000000000000000000),
 ( 1.000000000000000000, 0.5376207706124462860, 1.000000000000000000) ) ) 
 REPRESENTATION_ITEM ( '' )  SURFACE ( )  );
#16811=CARTESIAN_POINT ( 'NONE',  ( 2.121784821875004390, -17.10424616687832966, -6.553150170094818705 ) ) ;
#16814=CARTESIAN_POINT ( 'NONE',  ( 4.730628863548789710E-15, -19.14431419784868993, -11.60241431796419853 ) ) ;
#16816=CARTESIAN_POINT ( 'NONE',  ( 2.000000000000004441, -18.13202342554876267, -7.653209906595630940 ) ) ;
#16817=CARTESIAN_POINT ( 'NONE',  ( -14.99999999999999645, -4.000000000000000000, -30.00000000000000000 ) ) ;
#16823=DIRECTION ( 'NONE',  ( -0.000000000000000000, -0.000000000000000000, -1.000000000000000000 ) ) ;
#16824=CARTESIAN_POINT ( 'NONE',  ( 0.000000000000000000, 5.977523610840987267, 32.81826849749789687 ) ) ;
#16828=EDGE_CURVE ( 'NONE', #5641, #9296, #15600, .T. ) ;
#16829=AXIS2_PLACEMENT_3D ( 'NONE', #16768, #15545, #2932 ) ;
#16830=CARTESIAN_POINT ( 'NONE',  ( 2.121784821875004390, -21.20173283406107956, -12.40496758648432518 ) ) ;
#16834=CARTESIAN_POINT ( 'NONE',  ( 1.475796370471763337E-14, -22.05939178977998694, -14.19638352958117267 ) ) ;
#16837=CARTESIAN_POINT ( 'NONE',  ( 2.121784821874994176, -27.59897397692052934, -8.726704438383601214 ) ) ;
#16841=DIRECTION ( 'NONE',  ( -0.000000000000000000, 1.000000000000000000, -0.000000000000000000 ) ) ;
#16842=CARTESIAN_POINT ( 'NONE',  ( 2.121784821874994176, -24.98561633879609545, -4.994442936591867443 ) ) ;
#16843=DIRECTION ( 'NONE',  ( -0.000000000000000000, -0.000000000000000000, -1.000000000000000000 ) ) ;
#16851=CARTESIAN_POINT ( 'NONE',  ( 2.121784821874994176, -24.75977061698287329, -4.671901819153075230 ) ) ;
#16855=CARTESIAN_POINT ( 'NONE',  ( 0.000000000000000000, 5.977523610840987267, 32.81826849749789687 ) ) ;
#16860=DIRECTION ( 'NONE',  ( 0.5735764363510414965, -0.6710100716628397688, 0.4698463103929523821 ) ) ;
#16861=CARTESIAN_POINT ( 'NONE',  ( -2.121784821875005722, -28.64216612053397526, -10.21653721893421363 ) ) ;
#16864=CARTESIAN_POINT ( 'NONE',  ( -3.999999999999997335, -20.36844571459851139, -8.833992987396438679 ) ) ;
#16872=ORIENTED_EDGE ( 'NONE', *, *, #15, .F. ) ;
#16873=CARTESIAN_POINT ( 'NONE',  ( -2.121784821874996396, -22.22341586131136992, -13.86408216537410354 ) ) ;
#16876=EDGE_LOOP ( 'NONE', ( #5734, #2291, #4539, #14509 ) ) ;
#16883=CARTESIAN_POINT ( 'NONE',  ( 4.243569643750000786, -23.25499295915232167, -8.930091773994377036 ) ) ;
#16888=VERTEX_POINT ( 'NONE', #7529 ) ;
#16889=CARTESIAN_POINT ( 'NONE',  ( -3.999999999999997335, -22.69143028182022803, -12.15155876676686830 ) ) ;
#16890=FACE_OUTER_BOUND ( 'NONE', #12640, .T. ) ;
#16891=CARTESIAN_POINT ( 'NONE',  ( -4.000000000000000888, -25.78769141056240954, -12.54716001905459066 ) ) ;
#16895=EDGE_CURVE ( 'NONE', #15867, #8360, #8589, .T. ) ;
#16896=CARTESIAN_POINT ( 'NONE',  ( 4.000000000000000888, -25.72316406217786522, -12.45500541507884051 ) ) ;
#16899=CARTESIAN_POINT ( 'NONE',  ( 4.000000000000003553, -21.68050181204658244, -10.70780328770074696 ) ) ;
#16902=CARTESIAN_POINT ( 'NONE',  ( -2.121784821875005722, -23.51224186791935011, -2.890246122824515318 ) ) ;
#16904=CARTESIAN_POINT ( 'NONE',  ( -1.661723472263481630E-14, -20.57526276142661459, -12.07682761599016175 ) ) ;
#16905=CARTESIAN_POINT ( 'NONE',  ( 2.121784821875004390, -20.16929524862920431, -10.93049390676413601 ) ) ;
#16907=LINE ( 'NONE', #4183, #7172 ) ;
#16908=LINE ( 'NONE', #9565, #5288 ) ;
#16910=ORIENTED_EDGE ( 'NONE', *, *, #1795, .F. ) ;
#16912=CARTESIAN_POINT ( 'NONE',  ( -2.000000000000005773, -24.71065815213145100, -4.969520257213599024 ) ) ;
#16913=CARTESIAN_POINT ( 'NONE',  ( -5.577813053751546416E-15, -29.32240898478130120, -10.62147269458723464 ) ) ;
#16915=CARTESIAN_POINT ( 'NONE',  ( 3.999999999999996447, -24.79722043171331336, -7.106302957796752473 ) ) ;
#16919=CARTESIAN_POINT ( 'NONE',  ( -2.121784821875005722, -26.06107215695429247, -6.530353019633736267 ) ) ;
#16921=( BOUNDED_CURVE ( )  B_SPLINE_CURVE ( 1, ( #8121, #3952 ),
 .UNSPECIFIED., .F., .T. ) 
 B_SPLINE_CURVE_WITH_KNOTS ( ( 2, 2 ),
 ( 0.000000000000000000, 1.000000000000000000 ),
 .UNSPECIFIED. ) 
 CURVE ( )  GEOMETRIC_REPRESENTATION_ITEM ( )  RATIONAL_B_SPLINE_CURVE ( ( 0.9401540804572323662, 0.9401540804572323662 ) ) 
 REPRESENTATION_ITEM ( '' )  );
#16923=CARTESIAN_POINT ( 'NONE',  ( 3.772879157352770907, -10.00000000000000178, -12.59063537424807677 ) ) ;
#16924=DIRECTION ( 'NONE',  ( -0.000000000000000000, -0.5735764363510414965, -0.8191520442889950182 ) ) ;
#16925=CARTESIAN_POINT ( 'NONE',  ( -4.243569643749997233, -22.17294109393367307, -11.65625167113217664 ) ) ;
#16928=EDGE_CURVE ( 'NONE', #8838, #6628, #2240, .T. ) ;
#16929=CARTESIAN_POINT ( 'NONE',  ( 5.810221930991194676E-16, -23.67257551772224033, -16.50024865515073458 ) ) ;
#16930=DIRECTION ( 'NONE',  ( 0.000000000000000000, 0.8191520442889952403, -0.5735764363510413855 ) ) ;
#16931=CARTESIAN_POINT ( 'NONE',  ( -2.000000000000005773, -23.74274791649401095, -3.587201183482685352 ) ) ;
#16932=CARTESIAN_POINT ( 'NONE',  ( 4.730628863548789710E-15, -16.30511083791103744, -7.547611698733671659 ) ) ;
#16936=ORIENTED_EDGE ( 'NONE', *, *, #3559, .F. ) ;
#16938=CARTESIAN_POINT ( 'NONE',  ( 2.121784821875004390, -24.04093619399873560, -16.45977020571485028 ) ) ;
#16940=AXIS2_PLACEMENT_3D ( 'NONE', #9024, #13557, #6428 ) ;
#16941=CARTESIAN_POINT ( 'NONE',  ( -9.324442068587902810, -9.992495910828282035, -2.158041910186991874 ) ) ;
#16943=CARTESIAN_POINT ( 'NONE',  ( 4.243569643750000786, -19.89957080649872623, -4.138052314903757356 ) ) ;
#16946=CARTESIAN_POINT ( 'NONE',  ( -2.121784821875005722, -29.93271310232382021, -12.05962931858445231 ) ) ;
#16951=CARTESIAN_POINT ( 'NONE',  ( 4.730628863548789710E-15, -20.69297057599650813, -13.81412483754448495 ) ) ;
#16953=CARTESIAN_POINT ( 'NONE',  ( 1.533898589781675205E-14, -26.93489706776514581, -7.211752309227528634 ) ) ;
#16954=CARTESIAN_POINT ( 'NONE',  ( 2.000000000000004441, -17.42222258626929943, -6.639509252794765892 ) ) ;
#16956=ORIENTED_EDGE ( 'NONE', *, *, #6652, .F. ) ;
#16957=CARTESIAN_POINT ( 'NONE',  ( -3.999999999999997335, -20.36844571459851139, -8.833992987396436902 ) ) ;
#16963=ORIENTED_EDGE ( 'NONE', *, *, #14072, .F. ) ;
#16964=CARTESIAN_POINT ( 'NONE',  ( 4.243569643750003451, -23.54952454117618288, -13.62221657742576220 ) ) ;
#16968=VERTEX_POINT ( 'NONE', #9289 ) ;
#16972=DIRECTION ( 'NONE',  ( 0.000000000000000000, 0.000000000000000000, 1.000000000000000000 ) ) ;
#16974=CARTESIAN_POINT ( 'NONE',  ( 4.243569643750003451, -20.96843057759649653, -9.936032378125284836 ) ) ;
#16976=ORIENTED_EDGE ( 'NONE', *, *, #3538, .F. ) ;
#16979=CARTESIAN_POINT ( 'NONE',  ( -2.000000000000005773, -26.84006067278963670, -8.010622222643258183 ) ) ;
#16984=CARTESIAN_POINT ( 'NONE',  ( 4.000000000000000888, -26.23938285489380462, -13.19224225493893599 ) ) ;
#16986=CIRCLE ( 'NONE', #14914, 2.999999999999999556 ) ;
#16989=CARTESIAN_POINT ( 'NONE',  ( -3.999999999999997335, -21.33635595023594789, -10.21631206112735235 ) ) ;
#16991=ADVANCED_FACE ( 'NONE', ( #496 ), #4847, .F. ) ;
#16995=CARTESIAN_POINT ( 'NONE',  ( 9.911006336631391633, -9.930557276593896532, 8.884713581541163308 ) ) ;
#16996=CARTESIAN_POINT ( 'NONE',  ( 2.121784821875004390, -20.42740464498717401, -11.29911232669418197 ) ) ;
#16997=EDGE_CURVE ( 'NONE', #317, #4607, #6703, .T. ) ;
#17002=FACE_OUTER_BOUND ( 'NONE', #15613, .T. ) ;
#17004=VERTEX_POINT ( 'NONE', #10772 ) ;
#17008=CARTESIAN_POINT ( 'NONE',  ( -1.999999999999996225, -21.70253674183399184, -12.75243138229462758 ) ) ;
#17009=CARTESIAN_POINT ( 'NONE',  ( -4.000000000000000888, -26.88465634578871999, -14.11378830476406065 ) ) ;
#17012=CARTESIAN_POINT ( 'NONE',  ( -4.243569643750005227, -25.33721873525807666, -7.632328254085517294 ) ) ;
#17016=CARTESIAN_POINT ( 'NONE',  ( 1.999999999999994449, -27.82948002549519018, -9.423659499041770360 ) ) ;
#17018=CARTESIAN_POINT ( 'NONE',  ( -4.243569643750005227, -24.07893542801298281, -5.835313456926535025 ) ) ;
#17019=CARTESIAN_POINT ( 'NONE',  ( -14.99999999999999645, -4.000000000000000000, 30.00000000000000000 ) ) ;
#17021=FACE_OUTER_BOUND ( 'NONE', #18091, .T. ) ;
#17022=( BOUNDED_CURVE ( )  B_SPLINE_CURVE ( 2, ( #10336, #17614, #13211, #4592, #714, #15918, #3219, #14721, #9137 ),
 .UNSPECIFIED., .F., .T. ) 
 B_SPLINE_CURVE_WITH_KNOTS ( ( 3, 2, 2, 2, 3 ),
 ( 0.4051724137931034808, 0.4080459770114942541, 0.4137931034482758563, 0.4195402298850574585, 0.4224137931034482873 ),
 .UNSPECIFIED. ) 
 CURVE ( )  GEOMETRIC_REPRESENTATION_ITEM ( )  RATIONAL_B_SPLINE_CURVE ( ( 0.9330127018922194093, 0.9330127018922200755, 1.000000000000000000, 0.8660254037844387076, 1.000000000000000000, 0.8660254037844387076, 1.000000000000000000, 0.9330127018922187432, 0.9330127018922194093 ) ) 
 REPRESENTATION_ITEM ( '' )  );
#17023=CARTESIAN_POINT ( 'NONE',  ( -4.243569643749997233, -18.78525526673533719, -6.818134909550300549 ) ) ;
#17026=ORIENTED_EDGE ( 'NONE', *, *, #1626, .T. ) ;
#17028=CARTESIAN_POINT ( 'NONE',  ( -4.243569643750005227, -28.95075028426964181, -12.79298613310618471 ) ) ;
#17030=FACE_OUTER_BOUND ( 'NONE', #17426, .T. ) ;
#17034=CARTESIAN_POINT ( 'NONE',  ( 4.243569643749997233, -22.44424258441252817, -3.500730130702893295 ) ) ;
#17036=CARTESIAN_POINT ( 'NONE',  ( -4.243569643750004339, -27.40209390612183071, -10.58127561352589829 ) ) ;
#17039=LINE ( 'NONE', #12566, #8218 ) ;
#17040=CARTESIAN_POINT ( 'NONE',  ( -4.243569643749997233, -22.39878681574689523, -11.97879278857096885 ) ) ;
#17042=CARTESIAN_POINT ( 'NONE',  ( 3.579096709490575479E-14, -26.67678767140717966, -6.843133889297480899 ) ) ;
#17043=CARTESIAN_POINT ( 'NONE',  ( -4.000000000000004441, -21.78594414087033471, -2.805754725279534956 ) ) ;
#17045=ORIENTED_EDGE ( 'NONE', *, *, #13613, .F. ) ;
#17048=CARTESIAN_POINT ( 'NONE',  ( -4.000000000000000888, -23.01301540041918869, -8.584512005813342839 ) ) ;
#17052=CARTESIAN_POINT ( 'NONE',  ( 2.121784821874994176, -27.59897397692052934, -8.726704438383601214 ) ) ;
#17057=CARTESIAN_POINT ( 'NONE',  ( 4.299564228933482956E-15, -22.57561058249592278, -14.93362036944126814 ) ) ;
#17058=DIRECTION ( 'NONE',  ( -1.000000000000000000, 0.000000000000000000, 0.000000000000000000 ) ) ;
#17060=CARTESIAN_POINT ( 'NONE',  ( 2.000000000000004441, -23.29421135270813537, -15.02557830519658388 ) ) ;
#17061=CARTESIAN_POINT ( 'NONE',  ( 4.243569643749996345, -23.21857077348643017, -4.606585390493037835 ) ) ;
#17063=LINE ( 'NONE', #1656, #10274 ) ;
#17064=ORIENTED_EDGE ( 'NONE', *, *, #1516, .T. ) ;
#17065=VERTEX_POINT ( 'NONE', #9563 ) ;
#17069=CARTESIAN_POINT ( 'NONE',  ( -2.000000000000005773, -28.64682644729541749, -10.59095116215359234 ) ) ;
#17074=CARTESIAN_POINT ( 'NONE',  ( -5.279047395330986450E-15, -26.92557132411310050, -6.119585135346799376 ) ) ;
#17080=CARTESIAN_POINT ( 'NONE',  ( 9.000000000000005329, -10.00000000000000000, -3.713574246709344884 ) ) ;
#17081=CARTESIAN_POINT ( 'NONE',  ( 2.121784821874994176, -25.50183513151203130, -5.731679776451962915 ) ) ;
#17082=AXIS2_PLACEMENT_3D ( 'NONE', #2010, #11811, #13302 ) ;
#17086=ORIENTED_EDGE ( 'NONE', *, *, #13924, .F. ) ;
#17088=CARTESIAN_POINT ( 'NONE',  ( -2.343145750507621194, -3.999999999999994671, 25.54267522293723758 ) ) ;
#17094=CARTESIAN_POINT ( 'NONE',  ( -4.243569643750000786, -22.31934639735467840, -7.593850001747957990 ) ) ;
#17101=EDGE_CURVE ( 'NONE', #851, #15989, #2822, .T. ) ;
#17102=CARTESIAN_POINT ( 'NONE',  ( 2.121784821875004390, -19.16912133774208016, -9.502097529535200593 ) ) ;
#17107=CARTESIAN_POINT ( 'NONE',  ( 4.243569643750003451, -18.35507293947206264, -6.203770876333551954 ) ) ;
#17110=ORIENTED_EDGE ( 'NONE', *, *, #14072, .T. ) ;
#17115=CARTESIAN_POINT ( 'NONE',  ( 0.000000000000000000, 5.977523610840987267, 32.81826849749789687 ) ) ;
#17116=VERTEX_POINT ( 'NONE', #16638 ) ;
#17117=CARTESIAN_POINT ( 'NONE',  ( -2.121784821874996396, -17.31933733050996338, -6.860332186703194779 ) ) ;
#17120=CARTESIAN_POINT ( 'NONE',  ( 4.730628863548789710E-15, -22.79010942140500262, -16.80914949947612413 ) ) ;
#17123=CARTESIAN_POINT ( 'NONE',  ( 4.243569643749997233, -27.31605744066918007, -10.45840280688254431 ) ) ;
#17124=( BOUNDED_CURVE ( )  B_SPLINE_CURVE ( 2, ( #2725, #12439, #6960, #14018, #1329, #4009, #16912, #12618, #5398 ),
 .UNSPECIFIED., .F., .T. ) 
 B_SPLINE_CURVE_WITH_KNOTS ( ( 3, 2, 2, 2, 3 ),
 ( 0.6982758620689655249, 0.7011494252873563537, 0.7068965517241379004, 0.7126436781609195581, 0.7155172413793103869 ),
 .UNSPECIFIED. ) 
 CURVE ( )  GEOMETRIC_REPRESENTATION_ITEM ( )  RATIONAL_B_SPLINE_CURVE ( ( 0.9330127018922194093, 0.9330127018922194093, 1.000000000000000000, 0.8660254037844387076, 1.000000000000000000, 0.8660254037844387076, 1.000000000000000000, 0.9330127018922180770, 0.9330127018922194093 ) ) 
 REPRESENTATION_ITEM ( '' )  );
#17125=CARTESIAN_POINT ( 'NONE',  ( 0.000000000000000000, 5.977523610840987267, 32.81826849749789687 ) ) ;
#17126=CARTESIAN_POINT ( 'NONE',  ( -5.577813053751546416E-15, -24.09569370782749331, -3.156949689997003095 ) ) ;
#17128=CARTESIAN_POINT ( 'NONE',  ( -4.243569643749997233, -23.17311500482080433, -13.08464804836111206 ) ) ;
#17130=CARTESIAN_POINT ( 'NONE',  ( -5.279047395330986450E-15, -23.89278591761191350, -1.788318702175504038 ) ) ;
#17139=ORIENTED_EDGE ( 'NONE', *, *, #13200, .F. ) ;
#17140=CARTESIAN_POINT ( 'NONE',  ( -4.243569643750000786, -23.64215705368926379, -9.483019403889452192 ) ) ;
#17145=VECTOR ( 'NONE', #10660, 1000.000000000000000 ) ;
#17146=CARTESIAN_POINT ( 'NONE',  ( 2.000000000000004441, -17.16411318991132617, -6.270890832864717268 ) ) ;
#17148=CARTESIAN_POINT ( 'NONE',  ( 4.000000000000000888, -21.27077697429796288, -6.096337670278750842 ) ) ;
#17149=FACE_OUTER_BOUND ( 'NONE', #691, .T. ) ;
#17152=CARTESIAN_POINT ( 'NONE',  ( -2.121784821875005722, -23.77035126427731981, -3.258864542754563942 ) ) ;
#17154=EDGE_CURVE ( 'NONE', #8879, #13448, #5998, .T. ) ;
#17156=FACE_OUTER_BOUND ( 'NONE', #105, .T. ) ;
#17161=EDGE_CURVE ( 'NONE', #14266, #4345, #10392, .T. ) ;
#17166=EDGE_LOOP ( 'NONE', ( #15858, #13094, #995, #17996 ) ) ;
#17168=CARTESIAN_POINT ( 'NONE',  ( -2.000000000000005773, -25.74309573756332270, -6.443993936933789968 ) ) ;
#17169=VERTEX_POINT ( 'NONE', #13231 ) ;
#17175=CARTESIAN_POINT ( 'NONE',  ( -6.772465634063925322, -14.05063737647557964, -1.433670420094913522 ) ) ;
#17178=CARTESIAN_POINT ( 'NONE',  ( -4.243569643749998122, -19.81769285216720888, -8.292608589270493269 ) ) ;
#17181=CARTESIAN_POINT ( 'NONE',  ( -8.500000000000005329, 0.000000000000000000, 22.50000000000000000 ) ) ;
#17188=ORIENTED_EDGE ( 'NONE', *, *, #15651, .T. ) ;
#17190=CARTESIAN_POINT ( 'NONE',  ( -4.000000000000000888, -26.36843755307278414, -13.37655146490396341 ) ) ;
#17191=CARTESIAN_POINT ( 'NONE',  ( 4.243569643749996345, -24.47685408073152402, -6.403600187652020992 ) ) ;
#17195=CARTESIAN_POINT ( 'NONE',  ( -3.999999999999997335, -19.33600812916663614, -7.359519307676247735 ) ) ;
#17197=CARTESIAN_POINT ( 'NONE',  ( 4.730628863548789710E-15, -18.66035907967750163, -10.91125478059535681 ) ) ;
#17204=CARTESIAN_POINT ( 'NONE',  ( 2.121784821875004390, -18.10442007776545736, -7.981546547323755014 ) ) ;
#17206=( NAMED_UNIT ( * ) PLANE_ANGLE_UNIT ( ) SI_UNIT ( $, .RADIAN. ) );
#17207=ORIENTED_EDGE ( 'NONE', *, *, #3197, .T. ) ;
#17209=CARTESIAN_POINT ( 'NONE',  ( -4.243569643750005227, -28.43453149155370241, -12.05574929324608924 ) ) ;
#17210=LINE ( 'NONE', #3101, #4203 ) ;
#17212=LINE ( 'NONE', #13104, #13133 ) ;
#17215=CARTESIAN_POINT ( 'NONE',  ( -4.243569643749998122, -17.78508135584820948, -5.389738532321367792 ) ) ;
#17218=CARTESIAN_POINT ( 'NONE',  ( 2.121784821875004390, -23.81509047218551700, -16.13722908827605806 ) ) ;
#17219=CARTESIAN_POINT ( 'NONE',  ( 1.533898589781675205E-14, -26.93489706776514581, -7.211752309227528634 ) ) ;
#17220=CARTESIAN_POINT ( 'NONE',  ( 2.121784821874994176, -29.11536668052359289, -10.89233765547263211 ) ) ;
#17221=CARTESIAN_POINT ( 'NONE',  ( 3.064180744904201337, 3.871363374536846536, 34.29301777163557574 ) ) ;
#17223=EDGE_CURVE ( 'NONE', #1671, #12707, #7894, .T. ) ;
#17225=CARTESIAN_POINT ( 'NONE',  ( -4.243569643750005227, -27.14398450976385746, -10.21265719359585233 ) ) ;
#17227=CARTESIAN_POINT ( 'NONE',  ( -4.000000000000004441, -22.56027232994424025, -3.911609985069676387 ) ) ;
#17228=VECTOR ( 'NONE', #9225, 1000.000000000000000 ) ;
#17232=CARTESIAN_POINT ( 'NONE',  ( -1.071796769724496334, -20.56373606070777882, -12.06036578133424264 ) ) ;
#17236=ORIENTED_EDGE ( 'NONE', *, *, #7729, .F. ) ;
#17237=CARTESIAN_POINT ( 'NONE',  ( -4.243569643750004339, -25.88570120251876361, -8.415642396436870953 ) ) ;
#17240=ORIENTED_EDGE ( 'NONE', *, *, #15547, .T. ) ;
#17244=CARTESIAN_POINT ( 'NONE',  ( -2.121784821874996396, -22.73963465402730577, -14.60131900523419901 ) ) ;
#17245=CARTESIAN_POINT ( 'NONE',  ( 2.000000000000004441, -18.39013282190673237, -8.021828326525680453 ) ) ;
#17248=CARTESIAN_POINT ( 'NONE',  ( -5.330712181944245322E-15, -25.26853287504744472, -3.262744568092923014 ) ) ;
#17251=CARTESIAN_POINT ( 'NONE',  ( 3.276608177155980961, -25.09847727441901455, -15.56286022430290039 ) ) ;
#17255=VERTEX_POINT ( 'NONE', #14740 ) ;
#17256=CYLINDRICAL_SURFACE ( 'NONE', #10729, 4.000000000000000000 ) ;
#17261=ADVANCED_FACE ( 'NONE', ( #4706 ), #2888, .F. ) ;
#17262=ORIENTED_EDGE ( 'NONE', *, *, #8240, .T. ) ;
#17264=CARTESIAN_POINT ( 'NONE',  ( 4.000000000000000888, -22.81943335244577398, -8.308048189859038146 ) ) ;
#17266=CONICAL_SURFACE ( 'NONE', #18158, 2.000000000000001776, 1.029744260000000189 ) ;
#17267=CARTESIAN_POINT ( 'NONE',  ( 0.000000000000000000, 9.254131787996968228, 30.52396275209373044 ) ) ;
#17268=VECTOR ( 'NONE', #3145, 1000.000000000000000 ) ;
#17270=CARTESIAN_POINT ( 'NONE',  ( -7.143653376925515275, -13.70104873486882902, 0.6914076786229403915 ) ) ;
#17271=CARTESIAN_POINT ( 'NONE',  ( -4.243569643750000786, -21.80312760463873900, -6.856613161887861629 ) ) ;
#17287=CARTESIAN_POINT ( 'NONE',  ( 4.243569643750003451, -20.67805750669378284, -9.521336655703981577 ) ) ;
#17289=EDGE_CURVE ( 'NONE', #5876, #13013, #18100, .T. ) ;
#17292=CARTESIAN_POINT ( 'NONE',  ( -2.121784821874996396, -24.03018163581715072, -16.44441110488443769 ) ) ;
#17294=CARTESIAN_POINT ( 'NONE',  ( -2.000000000000005773, -29.87284607929082370, -12.34188865581455374 ) ) ;
#17295=CARTESIAN_POINT ( 'NONE',  ( 4.243569643750003451, -20.96843057759649653, -9.936032378125284836 ) ) ;
#17296=FACE_OUTER_BOUND ( 'NONE', #666, .T. ) ;
#17299=CARTESIAN_POINT ( 'NONE',  ( -6.660876705454564117, -10.00000000000000178, -8.457461752748960393 ) ) ;
#17300=CARTESIAN_POINT ( 'NONE',  ( 8.500000000000019540, 10.00000000000000000, -20.49999999999998934 ) ) ;
#17303=CARTESIAN_POINT ( 'NONE',  ( -5.330712181944245322E-15, -24.46194101142878807, -2.110812005811521619 ) ) ;
#17314=CARTESIAN_POINT ( 'NONE',  ( -2.121784821875005722, -29.19064858779466221, -10.99985136128556462 ) ) ;
#17316=EDGE_CURVE ( 'NONE', #9984, #8381, #9791, .T. ) ;
#17318=CARTESIAN_POINT ( 'NONE',  ( 4.243569643750003451, -24.03347965934736763, -14.31337611479460037 ) ) ;
#17319=DIRECTION ( 'NONE',  ( 0.000000000000000000, 0.5735764363510414965, 0.8191520442889950182 ) ) ;
#17321=CARTESIAN_POINT ( 'NONE',  ( -8.500000000000005329, 0.000000000000000000, 20.49999999999999645 ) ) ;
#17322=CARTESIAN_POINT ( 'NONE',  ( 4.243569643750000786, -25.02949505911335137, -11.46434341101345389 ) ) ;
#17323=CARTESIAN_POINT ( 'NONE',  ( 4.299564228933482956E-15, -18.51038759056286054, -9.127880256549779858 ) ) ;
#17324=CARTESIAN_POINT ( 'NONE',  ( 4.000000000000000888, -20.04475734230255668, -4.345400176617791210 ) ) ;
#17333=EDGE_CURVE ( 'NONE', #15033, #5353, #17407, .T. ) ;
#17335=CARTESIAN_POINT ( 'NONE',  ( 4.243569643750000786, -23.51310235551028782, -9.298710193924424772 ) ) ;
#17337=EDGE_CURVE ( 'NONE', #6382, #9005, #3327, .T. ) ;
#17340=CARTESIAN_POINT ( 'NONE',  ( -5.577813053751546416E-15, -24.87002189690140241, -4.262804949787145858 ) ) ;
#17341=CARTESIAN_POINT ( 'NONE',  ( 3.579096709490575479E-14, -25.70887743576973605, -5.460814815566567226 ) ) ;
#17342=CARTESIAN_POINT ( 'NONE',  ( 4.243569643750000786, -25.31986813001606862, -11.87903913343475892 ) ) ;
#17343=CARTESIAN_POINT ( 'NONE',  ( 3.999999999999996447, -23.18403670377106707, -4.802437832227187897 ) ) ;
#17345=CARTESIAN_POINT ( 'NONE',  ( 1.071796769724495224, -19.23171513056116666, -10.15804274500656312 ) ) ;
#17346=CARTESIAN_POINT ( 'NONE',  ( -2.121784821874996396, -17.83555612322590278, -7.597569026563290251 ) ) ;
#17347=ORIENTED_EDGE ( 'NONE', *, *, #14184, .F. ) ;
#17350=DIRECTION ( 'NONE',  ( -0.000000000000000000, -0.5735764363510414965, -0.8191520442889950182 ) ) ;
#17352=ORIENTED_EDGE ( 'NONE', *, *, #2817, .T. ) ;
#17353=DIRECTION ( 'NONE',  ( 0.000000000000000000, 0.8191520442889952403, -0.5735764363510413855 ) ) ;
#17360=CARTESIAN_POINT ( 'NONE',  ( 4.000000000000000888, -22.04510516337187198, -7.202192930068894938 ) ) ;
#17361=ORIENTED_EDGE ( 'NONE', *, *, #6478, .T. ) ;
#17364=CARTESIAN_POINT ( 'NONE',  ( 9.356317142028521161, -10.00000000000000000, 13.59402740589572645 ) ) ;
#17365=CARTESIAN_POINT ( 'NONE',  ( -5.330712181944246111E-15, -25.75248799321863657, -3.953904105461760743 ) ) ;
#17371=CARTESIAN_POINT ( 'NONE',  ( 0.000000000000000000, 9.254131787996968228, 30.52396275209373044 ) ) ;
#17377=CARTESIAN_POINT ( 'NONE',  ( -2.121784821874996396, -19.09383943047100018, -9.394583823722271632 ) ) ;
#17380=CARTESIAN_POINT ( 'NONE',  ( -2.121784821874996396, -23.77207223945918457, -16.07579268495438996 ) ) ;
#17381=CARTESIAN_POINT ( 'NONE',  ( 4.713407268011036227E-15, -23.10115511886391104, -16.76302438318209553 ) ) ;
#17382=CARTESIAN_POINT ( 'NONE',  ( 2.121784821874994176, -26.05031759877271469, -6.514993918803313910 ) ) ;
#17384=DIRECTION ( 'NONE',  ( -0.000000000000000000, -0.5735764363510414965, -0.8191520442889950182 ) ) ;
#17385=CARTESIAN_POINT ( 'NONE',  ( -7.003832385457668508, -10.00000000000000178, -7.945690313592825404 ) ) ;
#17392=CARTESIAN_POINT ( 'NONE',  ( -2.121784821874996396, -16.77085486324927999, -6.077018044351843784 ) ) ;
#17393=LINE ( 'NONE', #3285, #12483 ) ;
#17394=CARTESIAN_POINT ( 'NONE',  ( 4.000000000000000888, -20.56097613501849608, -5.082637016477885794 ) ) ;
#17399=CARTESIAN_POINT ( 'NONE',  ( -4.243569643749997233, -23.43122440117877048, -13.45326646829115980 ) ) ;
#17401=EDGE_CURVE ( 'NONE', #13289, #14065, #930, .T. ) ;
#17403=CARTESIAN_POINT ( 'NONE',  ( 0.000000000000000000, 5.977523610840987267, 32.81826849749789687 ) ) ;
#17406=CARTESIAN_POINT ( 'NONE',  ( -5.330712181944245322E-15, -30.94693959492275681, -11.37234980655397010 ) ) ;
#17407=( BOUNDED_CURVE ( )  B_SPLINE_CURVE ( 2, ( #10, #101, #15939, #11742, #16036 ),
 .UNSPECIFIED., .F., .T. ) 
 B_SPLINE_CURVE_WITH_KNOTS ( ( 3, 2, 3 ),
 ( 0.9913793103448276245, 0.9942528735632183423, 0.9961881922148684287 ),
 .UNSPECIFIED. ) 
 CURVE ( )  GEOMETRIC_REPRESENTATION_ITEM ( )  RATIONAL_B_SPLINE_CURVE ( ( 0.9330127018922194093, 0.9330127018922206306, 1.000000000000000000, 0.9548846649268323272, 0.9401540970596700131 ) ) 
 REPRESENTATION_ITEM ( '' )  );
#17408=EDGE_CURVE ( 'NONE', #3333, #12967, #9513, .T. ) ;
#17410=CARTESIAN_POINT ( 'NONE',  ( -2.121784821874996396, -22.70737097948255823, -14.55524170274294171 ) ) ;
#17411=DIRECTION ( 'NONE',  ( 0.000000000000000000, 0.8191520442889952403, -0.5735764363510413855 ) ) ;
#17412=CARTESIAN_POINT ( 'NONE',  ( -1.071796769724486564, -27.78527930735232232, -8.426224009662862002 ) ) ;
#17413=CYLINDRICAL_SURFACE ( 'NONE', #10879, 4.000000000000000000 ) ;
#17414=CARTESIAN_POINT ( 'NONE',  ( -4.243569643750000786, -23.60989337914451625, -9.436942101398194893 ) ) ;
#17416=CARTESIAN_POINT ( 'NONE',  ( 1.999999999999994449, -22.40918270197784778, -1.682672680510768792 ) ) ;
#17422=CARTESIAN_POINT ( 'NONE',  ( -5.279047395330986450E-15, -29.31308324112925945, -9.529305520706506272 ) ) ;
#17426=EDGE_LOOP ( 'NONE', ( #15659, #1211, #600, #6141, #9749, #4138 ) ) ;
#17427=CARTESIAN_POINT ( 'NONE',  ( 2.121784821875004390, -20.97588711224786095, -12.08242646904553474 ) ) ;
#17429=ORIENTED_EDGE ( 'NONE', *, *, #1700, .F. ) ;
#17431=CARTESIAN_POINT ( 'NONE',  ( -8.500000000000005329, 0.000000000000000000, -22.50000000000000000 ) ) ;
#17432=CARTESIAN_POINT ( 'NONE',  ( 4.243569643749996345, -27.34832111521392761, -10.50448010937380161 ) ) ;
#17435=CARTESIAN_POINT ( 'NONE',  ( -8.500000000000005329, 10.00000000000000000, -18.49999999999999645 ) ) ;
#17437=CARTESIAN_POINT ( 'NONE',  ( 1.071796769724494780, -26.98789771684074168, -7.287445080560893018 ) ) ;
#17438=CARTESIAN_POINT ( 'NONE',  ( 2.121784821875004390, -18.13668375231020846, -8.027623849815011425 ) ) ;
#17440=CARTESIAN_POINT ( 'NONE',  ( 1.533898589781675205E-14, -26.74131502120161841, -6.935288495286759058 ) ) ;
#17442=DIRECTION ( 'NONE',  ( -0.000000000000000000, -0.5735764363510414965, -0.8191520442889950182 ) ) ;
#17445=CYLINDRICAL_SURFACE ( 'NONE', #1868, 4.000000000000000000 ) ;
#17450=ORIENTED_EDGE ( 'NONE', *, *, #13056, .T. ) ;
#17454=CARTESIAN_POINT ( 'NONE',  ( 2.000000000000004441, -19.68067980369657377, -9.864920426175917356 ) ) ;
#17455=ORIENTED_EDGE ( 'NONE', *, *, #12426, .T. ) ;
#17458=CARTESIAN_POINT ( 'NONE',  ( 0.000000000000000000, 9.254131787996968228, 30.52396275209373044 ) ) ;
#17459=CARTESIAN_POINT ( 'NONE',  ( -4.243569643749998122, -19.04336466309330689, -7.186753329480350061 ) ) ;
#17466=CARTESIAN_POINT ( 'NONE',  ( 6.681132651088302232, -10.00000000000000178, 19.92483346546711687 ) ) ;
#17470=VERTEX_POINT ( 'NONE', #7942 ) ;
#17472=CARTESIAN_POINT ( 'NONE',  ( -3.999999999999997335, -24.49819605632600883, -14.73188770627719890 ) ) ;
#17473=CARTESIAN_POINT ( 'NONE',  ( -2.121784821874996396, -17.80329244868115168, -7.551491724072033840 ) ) ;
#17476=CARTESIAN_POINT ( 'NONE',  ( 4.243569643750000786, -27.12663390452184942, -14.45936807294509308 ) ) ;
#17477=VECTOR ( 'NONE', #2110, 1000.000000000000000 ) ;
#17478=CARTESIAN_POINT ( 'NONE',  ( 2.000000000000004441, -23.29421135270813537, -15.02557830519658388 ) ) ;
#17480=CARTESIAN_POINT ( 'NONE',  ( 4.243569643749996345, -23.47668016984439632, -4.975203810423082906 ) ) ;
#17481=AXIS2_PLACEMENT_3D ( 'NONE', #16326, #9261, #17823 ) ;
#17482=CARTESIAN_POINT ( 'NONE',  ( -4.000000000000003553, 6.938893903907228378E-15, 24.28148006742132026 ) ) ;
#17484=DIRECTION ( 'NONE',  ( -0.000000000000000000, -0.5735764363510414965, -0.8191520442889950182 ) ) ;
#17485=VECTOR ( 'NONE', #8728, 1000.000000000000000 ) ;
#17487=ORIENTED_EDGE ( 'NONE', *, *, #17577, .T. ) ;
#17488=ORIENTED_EDGE ( 'NONE', *, *, #17337, .F. ) ;
#17490=CARTESIAN_POINT ( 'NONE',  ( 1.071796769724485232, -28.98824553791006764, -10.14423783401199586 ) ) ;
#17491=CARTESIAN_POINT ( 'NONE',  ( 1.999999999999994449, -23.44162028740971948, -3.157146360230959292 ) ) ;
#17493=VECTOR ( 'NONE', #8471, 1000.000000000000000 ) ;
#17496=CARTESIAN_POINT ( 'NONE',  ( 4.730628863548789710E-15, -21.46729876507041013, -14.91998009733462816 ) ) ;
#17499=CARTESIAN_POINT ( 'NONE',  ( 4.778136680858137808, -10.00000000000000000, -10.60429372729831243 ) ) ;
#17500=ADVANCED_FACE ( 'NONE', ( #12023 ), #14932, .F. ) ;
#17503=CARTESIAN_POINT ( 'NONE',  ( 4.243569643750003451, -23.80763393753414903, -13.99083499735581171 ) ) ;
#17506=AXIS2_PLACEMENT_3D ( 'NONE', #2648, #12634, #10882 ) ;
#17508=CARTESIAN_POINT ( 'NONE',  ( -2.121784821874996396, -21.93304279040865623, -13.44938644295279850 ) ) ;
#17510=CARTESIAN_POINT ( 'NONE',  ( -3.999999999999997335, -18.30357054373476799, -5.885045627956057679 ) ) ;
#17511=DIRECTION ( 'NONE',  ( 0.000000000000000000, 0.000000000000000000, 1.000000000000000000 ) ) ;
#17512=CARTESIAN_POINT ( 'NONE',  ( 4.243569643750003451, -21.71049509212565454, -10.99581033542417252 ) ) ;
#17514=CARTESIAN_POINT ( 'NONE',  ( 15.00000000000000355, 10.00000000000000000, 30.00000000000000000 ) ) ;
#17516=EDGE_LOOP ( 'NONE', ( #11855, #15894, #15298, #1490 ) ) ;
#17518=CARTESIAN_POINT ( 'NONE',  ( 3.999999999999996447, -26.34587680986112801, -9.318013477377039777 ) ) ;
#17520=CIRCLE ( 'NONE', #5926, 2.000000000000001776 ) ;
#17521=CARTESIAN_POINT ( 'NONE',  ( -2.000000000000005773, -28.13060765457947809, -9.853714322293496863 ) ) ;
#17524=( BOUNDED_CURVE ( )  B_SPLINE_CURVE ( 2, ( #16451, #13469, #12256, #2183, #16270, #18038, #7993, #6692, #3561 ),
 .UNSPECIFIED., .F., .T. ) 
 B_SPLINE_CURVE_WITH_KNOTS ( ( 3, 2, 2, 2, 3 ),
 ( 0.1637931034482758563, 0.1666666666666666574, 0.1724137931034482873, 0.1781609195402298895, 0.1810344827586206906 ),
 .UNSPECIFIED. ) 
 CURVE ( )  GEOMETRIC_REPRESENTATION_ITEM ( )  RATIONAL_B_SPLINE_CURVE ( ( 0.9330127018922194093, 0.9330127018922194093, 1.000000000000000000, 0.8660254037844387076, 1.000000000000000000, 0.8660254037844387076, 1.000000000000000000, 0.9330127018922194093, 0.9330127018922194093 ) ) 
 REPRESENTATION_ITEM ( '' )  );
#17526=CARTESIAN_POINT ( 'NONE',  ( -4.243569643750004339, -25.36948240980282421, -7.678405556576772817 ) ) ;
#17532=CARTESIAN_POINT ( 'NONE',  ( -4.243569643750005227, -27.43435758066657471, -10.62735291601715382 ) ) ;
#17533=AXIS2_PLACEMENT_3D ( 'NONE', #9131, #2200, #16193 ) ;
#17535=CARTESIAN_POINT ( 'NONE',  ( 1.533898589781675205E-14, -26.99942441755958811, -7.303906915216807683 ) ) ;
#17536=CARTESIAN_POINT ( 'NONE',  ( 2.769793372871041104, -22.38185876178289746, -1.928163851144596430 ) ) ;
#17538=CARTESIAN_POINT ( 'NONE',  ( 2.000000000000004441, -20.77764473892288777, -11.43154871188538557 ) ) ;
#17539=CARTESIAN_POINT ( 'NONE',  ( 1.475796370471763337E-14, -21.86580974321645598, -13.91991971564040220 ) ) ;
#17542=CARTESIAN_POINT ( 'NONE',  ( 4.299564228933482956E-15, -20.83337215778458074, -12.44544603592020771 ) ) ;
#17551=CARTESIAN_POINT ( 'NONE',  ( -4.000000000000000888, -22.17415986155084795, -7.386502140033922359 ) ) ;
#17555=CARTESIAN_POINT ( 'NONE',  ( 1.071796769724485232, -28.73013614155210149, -9.775619414081942793 ) ) ;
#17556=CARTESIAN_POINT ( 'NONE',  ( -2.121784821874996396, -18.83573003411303048, -9.025965403792225672 ) ) ;
#17557=CARTESIAN_POINT ( 'NONE',  ( -4.243569643749997233, -22.43105049029164277, -12.02487009106222615 ) ) ;
#17558=CARTESIAN_POINT ( 'NONE',  ( -1.999999999999996225, -20.15388036368618074, -10.54072086271434117 ) ) ;
#17559=VERTEX_POINT ( 'NONE', #12205 ) ;
#17560=CARTESIAN_POINT ( 'NONE',  ( 5.954418220269343642, -10.00000000000000178, 20.87519200589467872 ) ) ;
#17561=CARTESIAN_POINT ( 'NONE',  ( 1.999999999999994449, -24.99027666555753413, -5.368856879811245264 ) ) ;
#17562=CARTESIAN_POINT ( 'NONE',  ( 1.533898589781675205E-14, -28.22544404955499786, -9.054844408877768203 ) ) ;
#17566=CARTESIAN_POINT ( 'NONE',  ( 2.121784821874994176, -24.98561633879609545, -4.994442936591867443 ) ) ;
#17572=CARTESIAN_POINT ( 'NONE',  ( 2.121784821875004390, -24.07319986854348670, -16.50584750820610580 ) ) ;
#17573=CARTESIAN_POINT ( 'NONE',  ( -5.279047395330986450E-15, -29.76477468405075300, -10.17438775457732625 ) ) ;
#17575=CARTESIAN_POINT ( 'NONE',  ( -4.243569643750000786, -23.38404765733129764, -9.114400983959404456 ) ) ;
#17576=CARTESIAN_POINT ( 'NONE',  ( 4.243569643750003451, -19.16166480309071574, -7.355703438614951573 ) ) ;
#17577=EDGE_CURVE ( 'NONE', #10853, #244, #4703, .T. ) ;
#17578=CARTESIAN_POINT ( 'NONE',  ( -6.618784548698717352, -14.16206772970377159, -2.127281972413720634 ) ) ;
#17584=VERTEX_POINT ( 'NONE', #2762 ) ;
#17587=CARTESIAN_POINT ( 'NONE',  ( 1.071796769724485232, -24.08416700710866110, -3.140487855341086654 ) ) ;
#17593=CARTESIAN_POINT ( 'NONE',  ( 2.121784821875004390, -23.00849860856686036, -14.98529652599465933 ) ) ;
#17596=CARTESIAN_POINT ( 'NONE',  ( 0.6435590302261994244, -15.45066141473231980, -10.82404826198633430 ) ) ;
#17598=VECTOR ( 'NONE', #6493, 1000.000000000000000 ) ;
#17599=CARTESIAN_POINT ( 'NONE',  ( -4.243569643749997233, -23.20537867936554832, -13.13072535085237114 ) ) ;
#17601=CARTESIAN_POINT ( 'NONE',  ( 4.243569643749997233, -26.54172925159527097, -9.352547547092401103 ) ) ;
#17605=CARTESIAN_POINT ( 'NONE',  ( -5.330712181944245322E-15, -27.04303497500847797, -5.796996205112000311 ) ) ;
#17607=CARTESIAN_POINT ( 'NONE',  ( -8.500000000000005329, 10.00000000000000000, -22.50000000000000000 ) ) ;
#17608=CIRCLE ( 'NONE', #9578, 4.000000000000000888 ) ;
#17613=EDGE_CURVE ( 'NONE', #18256, #8069, #14186, .T. ) ;
#17614=CARTESIAN_POINT ( 'NONE',  ( 1.071796769724494780, -27.24600711319871493, -7.656063500490938978 ) ) ;
#17616=CARTESIAN_POINT ( 'NONE',  ( 4.000000000000000888, -20.30286673866052283, -4.714018596547838946 ) ) ;
#17619=CARTESIAN_POINT ( 'NONE',  ( -5.330712181944246111E-15, -27.07529864955322552, -5.843073507603255834 ) ) ;
#17625=CARTESIAN_POINT ( 'NONE',  ( 4.243569643750003451, -23.03330574846024703, -12.88497973756566672 ) ) ;
#17626=CARTESIAN_POINT ( 'NONE',  ( -1.999999999999996225, -22.54139228070233614, -13.95044124807404451 ) ) ;
#17627=CARTESIAN_POINT ( 'NONE',  ( 7.484523392482447690, -12.68578631963116621, 7.186755514441455439 ) ) ;
#17629=CARTESIAN_POINT ( 'NONE',  ( -5.330712181944245322E-15, -24.23609528961556947, -1.788270888372730960 ) ) ;
#17631=EDGE_LOOP ( 'NONE', ( #796, #7765, #10939, #5625 ) ) ;
#17632=DIRECTION ( 'NONE',  ( -0.000000000000000000, -0.000000000000000000, -1.000000000000000000 ) ) ;
#17633=CARTESIAN_POINT ( 'NONE',  ( -3.999999999999997335, -20.88466450731445079, -9.571229827256534151 ) ) ;
#17637=( BOUNDED_CURVE ( )  B_SPLINE_CURVE ( 2, ( #15554, #17232, #10054, #3029, #7276, #16198, #6072, #3489, #16015 ),
 .UNSPECIFIED., .F., .T. ) 
 B_SPLINE_CURVE_WITH_KNOTS ( ( 3, 2, 2, 2, 3 ),
 ( 0.4224137931034482873, 0.4252873563218390607, 0.4310344827586206629, 0.4367816091954023205, 0.4396551724137931494 ),
 .UNSPECIFIED. ) 
 CURVE ( )  GEOMETRIC_REPRESENTATION_ITEM ( )  RATIONAL_B_SPLINE_CURVE ( ( 0.9330127018922194093, 0.9330127018922200755, 1.000000000000000000, 0.8660254037844387076, 1.000000000000000000, 0.8660254037844387076, 1.000000000000000000, 0.9330127018922187432, 0.9330127018922194093 ) ) 
 REPRESENTATION_ITEM ( '' )  );
#17646=CARTESIAN_POINT ( 'NONE',  ( 4.000000000000003553, -20.13184543389876779, -8.496092768120460548 ) ) ;
#17647=ORIENTED_EDGE ( 'NONE', *, *, #6077, .F. ) ;
#17651=CARTESIAN_POINT ( 'NONE',  ( 2.121784821874994176, -23.17885056429031465, -2.414113997081532847 ) ) ;
#17652=CARTESIAN_POINT ( 'NONE',  ( -4.243569643750005227, -26.40191999523469946, -9.152879236296964649 ) ) ;
#17653=CARTESIAN_POINT ( 'NONE',  ( -2.000000000000005773, -25.74309573756332270, -6.443993936933789968 ) ) ;
#17655=CARTESIAN_POINT ( 'NONE',  ( -6.097036691290805166, -11.55344374157283660, 15.47841750116366377 ) ) ;
#17658=CARTESIAN_POINT ( 'NONE',  ( 2.121784821874994176, -29.66384914778427628, -11.67565179782398310 ) ) ;
#17662=CARTESIAN_POINT ( 'NONE',  ( 4.243569643750000786, -21.67407290645975948, -6.672303951922835097 ) ) ;
#17665=CARTESIAN_POINT ( 'NONE',  ( -2.121784821874996396, -23.25585344674324162, -15.33855584509429271 ) ) ;
#17666=CARTESIAN_POINT ( 'NONE',  ( 3.999999999999996447, -28.08811523457247006, -11.80618781089809488 ) ) ;
#17667=CARTESIAN_POINT ( 'NONE',  ( 2.121784821875004390, -17.87857435595223876, -7.659005429884962801 ) ) ;
#17670=CARTESIAN_POINT ( 'NONE',  ( 4.000000000000003553, -18.32507965939299055, -5.915763828610125508 ) ) ;
#17671=CARTESIAN_POINT ( 'NONE',  ( 3.250762944584260072, -21.87258937905581746, -2.200190645090608133 ) ) ;
#17673=VERTEX_POINT ( 'NONE', #5348 ) ;
#17674=CARTESIAN_POINT ( 'NONE',  ( 3.250762944584260516, -21.87258937905581746, -2.200190645090608133 ) ) ;
#17677=CARTESIAN_POINT ( 'NONE',  ( 6.428571428571431490, -11.73421655796352425, 14.25837509840157935 ) ) ;
#17680=CARTESIAN_POINT ( 'NONE',  ( -4.243569643749997233, -23.68933379753673663, -13.82188488822120931 ) ) ;
#17684=VECTOR ( 'NONE', #11803, 1000.000000000000000 ) ;
#17685=CARTESIAN_POINT ( 'NONE',  ( 1.281796014811036999, -15.42359483004404730, -10.64137488400890597 ) ) ;
#17686=CARTESIAN_POINT ( 'NONE',  ( 4.243569643750003451, -24.06574333389212228, -14.35945341728585767 ) ) ;
#17688=CARTESIAN_POINT ( 'NONE',  ( 4.005420803925811235, -27.01550616763517709, -14.30066121701663029 ) ) ;
#17690=AXIS2_PLACEMENT_3D ( 'NONE', #3298, #1920, #7547 ) ;
#17691=CARTESIAN_POINT ( 'NONE',  ( 4.243569643749996345, -24.99307287344746342, -7.140837027512114688 ) ) ;
#17693=LINE ( 'NONE', #17607, #17228 ) ;
#17699=CARTESIAN_POINT ( 'NONE',  ( -4.000000000000000888, -26.62654694943075029, -13.74516988483401114 ) ) ;
#17703=ORIENTED_EDGE ( 'NONE', *, *, #4223, .T. ) ;
#17704=CARTESIAN_POINT ( 'NONE',  ( -5.330712181944246111E-15, -26.30097046047931997, -4.737218247813112626 ) ) ;
#17710=CARTESIAN_POINT ( 'NONE',  ( -3.446515024960077778, -28.75821711830315408, -13.15225657165725082 ) ) ;
#17713=CARTESIAN_POINT ( 'NONE',  ( -1.071796769724477238, -24.94607594741468048, -4.371421390432334242 ) ) ;
#17714=CARTESIAN_POINT ( 'NONE',  ( 2.121784821875004390, -16.84613677052036351, -6.184531750164772745 ) ) ;
#17716=CARTESIAN_POINT ( 'NONE',  ( 0.000000000000000000, 5.977523610840987267, 32.81826849749789687 ) ) ;
#17717=CARTESIAN_POINT ( 'NONE',  ( -3.999999999999997335, -21.40088330003038664, -10.30846666711663140 ) ) ;
#17728=CARTESIAN_POINT ( 'NONE',  ( 4.000000000000003553, -20.38995483025674105, -8.864711188050506507 ) ) ;
#17732=FACE_OUTER_BOUND ( 'NONE', #2581, .T. ) ;
#17734=CIRCLE ( 'NONE', #14151, 0.4000000000000006883 ) ;
#17737=ADVANCED_FACE ( 'NONE', ( #1094 ), #11001, .F. ) ;
#17738=CARTESIAN_POINT ( 'NONE',  ( -4.243569643749998122, -18.78525526673533719, -6.818134909550301437 ) ) ;
#17739=( BOUNDED_CURVE ( )  B_SPLINE_CURVE ( 2, ( #17340, #12013, #3318, #727, #6184, #15929, #11644, #13038, #1839 ),
 .UNSPECIFIED., .F., .F. ) 
 B_SPLINE_CURVE_WITH_KNOTS ( ( 3, 2, 2, 2, 3 ),
 ( 0.7500000000000000000, 0.7528735632183908288, 0.7586206896551723755, 0.7643678160919540332, 0.7672413793103448620 ),
 .UNSPECIFIED. ) 
 CURVE ( )  GEOMETRIC_REPRESENTATION_ITEM ( )  RATIONAL_B_SPLINE_CURVE ( ( 0.9330127018922194093, 0.9330127018922194093, 1.000000000000000000, 0.8660254037844387076, 1.000000000000000000, 0.8660254037844387076, 1.000000000000000000, 0.9330127018922180770, 0.9330127018922194093 ) ) 
 REPRESENTATION_ITEM ( '' )  );
#17740=CARTESIAN_POINT ( 'NONE',  ( 4.243569643750000786, -24.80364933730013277, -11.14180229357466345 ) ) ;
#17744=CARTESIAN_POINT ( 'NONE',  ( 4.386042834387938960, -10.00000000000000178, 22.42214358049745826 ) ) ;
#17747=CARTESIAN_POINT ( 'NONE',  ( -3.706921591972381904E-14, -19.54282517599473579, -10.60235393626997080 ) ) ;
#17748=ORIENTED_EDGE ( 'NONE', *, *, #4953, .T. ) ;
#17752=CARTESIAN_POINT ( 'NONE',  ( 4.730628863548789710E-15, -16.04700144155306774, -7.178993278803624811 ) ) ;
#17756=CARTESIAN_POINT ( 'NONE',  ( 1.999999999999994449, -28.53928086477465698, -10.43736015284263807 ) ) ;
#17758=CARTESIAN_POINT ( 'NONE',  ( -4.243569643750005227, -22.78838844622314497, -3.992221357276296345 ) ) ;
#17762=B_SPLINE_CURVE_WITH_KNOTS ( 'NONE', 1,
 ( #16490, #10997 ),
 .UNSPECIFIED., .F., .F.,
 ( 2, 2 ),
 ( 0.6192647773654433863, 1.000000000000000000 ),
 .UNSPECIFIED. ) ;
#17768=CARTESIAN_POINT ( 'NONE',  ( 4.730628863548789710E-15, -15.78889204519509981, -6.810374858873577075 ) ) ;
#17769=DIRECTION ( 'NONE',  ( 1.000000000000000000, 0.000000000000000000, 0.000000000000000000 ) ) ;
#17770=CARTESIAN_POINT ( 'NONE',  ( 4.000000000000000888, -24.10998033423561893, -10.15114028950927683 ) ) ;
#17774=CARTESIAN_POINT ( 'NONE',  ( 4.243569643750000786, -25.80382324818726048, -12.57019867080359710 ) ) ;
#17780=CARTESIAN_POINT ( 'NONE',  ( 1.794514420735380256, -10.00000000000000178, -12.33839425357223618 ) ) ;
#17781=CARTESIAN_POINT ( 'NONE',  ( 4.243569643750000786, -25.06175873365810247, -11.51042071350471119 ) ) ;
#17784=FACE_OUTER_BOUND ( 'NONE', #12668, .T. ) ;
#17786=CARTESIAN_POINT ( 'NONE',  ( 4.243569643750003451, -21.19427629940971869, -10.25857349556407527 ) ) ;
#17788=CARTESIAN_POINT ( 'NONE',  ( -8.500000000000005329, 0.000000000000000000, 18.49999999999999645 ) ) ;
#17791=SHAPE_REPRESENTATION ( 'Brass Valve Body', ( #16940 ), #12175 ) ;
#17797=CARTESIAN_POINT ( 'NONE',  ( 2.121784821875004390, -20.20155892317395541, -10.97657120925539154 ) ) ;
#17804=DIRECTION ( 'NONE',  ( 0.000000000000000000, 1.000000000000000000, 0.000000000000000000 ) ) ;
#17805=CARTESIAN_POINT ( 'NONE',  ( 9.604546805300321566, -9.971739665363084981, 12.06860958386529781 ) ) ;
#17806=CARTESIAN_POINT ( 'NONE',  ( 4.898587196589412829E-16, 10.00000000000000000, -4.000000000000000000 ) ) ;
#17807=CARTESIAN_POINT ( 'NONE',  ( 3.250762944584260516, -21.90485305360056145, -2.246267947581864100 ) ) ;
#17808=VERTEX_POINT ( 'NONE', #10236 ) ;
#17810=CARTESIAN_POINT ( 'NONE',  ( -2.000000000000005773, -25.29140429464182560, -5.798911703062972656 ) ) ;
#17814=EDGE_LOOP ( 'NONE', ( #12962, #12938, #13047, #16227, #14203, #4443, #125, #3240, #4216 ) ) ;
#17815=FACE_OUTER_BOUND ( 'NONE', #12977, .T. ) ;
#17819=ORIENTED_EDGE ( 'NONE', *, *, #12711, .T. ) ;
#17821=CARTESIAN_POINT ( 'NONE',  ( 2.000000000000004441, -17.87391402919079653, -7.284591486665584981 ) ) ;
#17823=DIRECTION ( 'NONE',  ( 0.000000000000000000, 0.8191520442889952403, -0.5735764363510413855 ) ) ;
#17825=CARTESIAN_POINT ( 'NONE',  ( 1.999999999999994449, -26.73251509026887618, -7.857031213332303921 ) ) ;
#17826=CARTESIAN_POINT ( 'NONE',  ( -2.121784821875005722, -23.47997819337460257, -2.844168820333258907 ) ) ;
#17827=CARTESIAN_POINT ( 'NONE',  ( -4.243569643749997233, -21.91483169757570693, -11.28763325120213068 ) ) ;
#17828=CARTESIAN_POINT ( 'NONE',  ( -0.7766474010173821663, -30.24966125638259840, -12.04527715262853604 ) ) ;
#17830=CARTESIAN_POINT ( 'NONE',  ( -2.000000000000005773, -22.64578298126770051, -2.020572897773216692 ) ) ;
#17831=EDGE_CURVE ( 'NONE', #6378, #3053, #6607, .T. ) ;
#17832=CARTESIAN_POINT ( 'NONE',  ( 9.000000000000003553, -4.000000000000000000, 30.00000000000000000 ) ) ;
#17833=CARTESIAN_POINT ( 'NONE',  ( -4.243569643749997233, -24.49592566115538972, -14.97381745050260804 ) ) ;
#17837=CARTESIAN_POINT ( 'NONE',  ( 2.121784821875004390, -17.07198249233357856, -6.507072867603563182 ) ) ;
#17841=CARTESIAN_POINT ( 'NONE',  ( 4.000000000000003553, -23.48726758655236324, -13.28813222721107934 ) ) ;
#17843=CARTESIAN_POINT ( 'NONE',  ( 4.243569643750000786, -21.44822718464654088, -6.349762834484042884 ) ) ;
#17846=DIRECTION ( 'NONE',  ( 0.000000000000000000, 0.8191520442889952403, -0.5735764363510413855 ) ) ;
#17847=DIRECTION ( 'NONE',  ( -0.000000000000000000, -0.5735764363510414965, -0.8191520442889950182 ) ) ;
#17849=ORIENTED_EDGE ( 'NONE', *, *, #18191, .F. ) ;
#17851=EDGE_CURVE ( 'NONE', #6628, #2835, #1519, .T. ) ;
#17852=EDGE_CURVE ( 'NONE', #10853, #1671, #1823, .T. ) ;
#17854=CARTESIAN_POINT ( 'NONE',  ( 2.000000000000004441, -23.87495749521851351, -15.85496975104595840 ) ) ;
#17856=ORIENTED_EDGE ( 'NONE', *, *, #5856, .T. ) ;
#17860=CARTESIAN_POINT ( 'NONE',  ( -4.243569643749997233, -22.14067741938892908, -11.61017436864092112 ) ) ;
#17863=CARTESIAN_POINT ( 'NONE',  ( 1.622307724309302010E-14, -9.999999999999998224, -3.075850967158335614 ) ) ;
#17865=CARTESIAN_POINT ( 'NONE',  ( 4.243569643749996345, -27.60643051157189731, -10.87309852930384935 ) ) ;
#17868=LINE ( 'NONE', #2283, #9763 ) ;
#17870=CARTESIAN_POINT ( 'NONE',  ( -4.243569643750005227, -24.04667175346823527, -5.789236154435278614 ) ) ;
#17873=CARTESIAN_POINT ( 'NONE',  ( -8.500000000000005329, 0.000000000000000000, 22.50000000000000000 ) ) ;
#17880=ORIENTED_EDGE ( 'NONE', *, *, #5369, .T. ) ;
#17881=CARTESIAN_POINT ( 'NONE',  ( 4.243569643749997233, -22.96046137712846047, -4.237966970562988323 ) ) ;
#17888=AXIS2_PLACEMENT_3D ( 'NONE', #2683, #1289, #6920 ) ;
#17889=CARTESIAN_POINT ( 'NONE',  ( 7.381366913268024632, -13.34886440523947648, 2.833380585799200269 ) ) ;
#17890=CARTESIAN_POINT ( 'NONE',  ( 2.121784821875004390, -17.62046495959427261, -7.290387009954915953 ) ) ;
#17893=CARTESIAN_POINT ( 'NONE',  ( 4.000000000000000888, -23.65828889131411827, -9.506058055638460402 ) ) ;
#17896=VERTEX_POINT ( 'NONE', #1633 ) ;
#17897=CARTESIAN_POINT ( 'NONE',  ( 3.999999999999996447, -28.15264258436690525, -11.89834241688737393 ) ) ;
#17901=CARTESIAN_POINT ( 'NONE',  ( 1.071796769724494780, -26.92337036704631004, -7.195290474571613970 ) ) ;
#17907=CARTESIAN_POINT ( 'NONE',  ( -3.999999999999997335, -19.52959017573017064, -7.635983121617017311 ) ) ;
#17908=VERTEX_POINT ( 'NONE', #523 ) ;
#17913=CARTESIAN_POINT ( 'NONE',  ( -4.243569643750004339, -22.23990597896245447, -3.208907214924944462 ) ) ;
#17914=CARTESIAN_POINT ( 'NONE',  ( -2.121784821874996396, -21.44908767223746437, -12.75822690558396033 ) ) ;
#17916=CARTESIAN_POINT ( 'NONE',  ( 0.000000000000000000, 5.977523610840987267, 32.81826849749789687 ) ) ;
#17918=CARTESIAN_POINT ( 'NONE',  ( 4.898587196589417759E-16, -3.999999999999993339, 25.54267522293723758 ) ) ;
#17920=CARTESIAN_POINT ( 'NONE',  ( -2.121784821875005722, -29.44875798415262835, -11.36846978121561236 ) ) ;
#17925=CARTESIAN_POINT ( 'NONE',  ( 4.243569643750003451, -18.09696354311409294, -5.835152456403505106 ) ) ;
#17929=CARTESIAN_POINT ( 'NONE',  ( 1.999999999999994449, -28.02306207205872113, -9.700123312982540824 ) ) ;
#17931=CARTESIAN_POINT ( 'NONE',  ( -2.121784821875005722, -22.73791367884544812, -1.784390863034371666 ) ) ;
#17934=CARTESIAN_POINT ( 'NONE',  ( 4.243569643750003451, -21.96860448848362779, -11.36442875535422026 ) ) ;
#17936=CARTESIAN_POINT ( 'NONE',  ( 1.071796769724494780, -27.69769855612021558, -8.301145734361757178 ) ) ;
#17941=CARTESIAN_POINT ( 'NONE',  ( 1.999999999999994449, -24.47405787284159828, -4.631620039951150680 ) ) ;
#17942=CARTESIAN_POINT ( 'NONE',  ( 7.343428405759329536, -12.39714631489042418, 9.301343483023684300 ) ) ;
#17946=CARTESIAN_POINT ( 'NONE',  ( -4.243569643749997233, -21.62445862667299323, -10.87293752878082742 ) ) ;
#17950=DIRECTION ( 'NONE',  ( 0.000000000000000000, -0.5735764363510567065, -0.8191520442889842490 ) ) ;
#17951=CARTESIAN_POINT ( 'NONE',  ( 2.121784821875004390, -21.23399650860583066, -12.45104488897558248 ) ) ;
#17952=ADVANCED_FACE ( 'NONE', ( #4407 ), #10048, .F. ) ;
#17956=ADVANCED_FACE ( 'NONE', ( #14906 ), #620, .F. ) ;
#17959=CARTESIAN_POINT ( 'NONE',  ( -5.330712181944245322E-15, -26.26870678593457242, -4.691140945321855327 ) ) ;
#17961=ORIENTED_EDGE ( 'NONE', *, *, #15547, .F. ) ;
#17962=FACE_BOUND ( 'NONE', #11730, .T. ) ;
#17963=DIRECTION ( 'NONE',  ( -0.000000000000000000, -0.5735764363510414965, -0.8191520442889950182 ) ) ;
#17968=CARTESIAN_POINT ( 'NONE',  ( -3.999999999999997335, -23.40123112109970194, -13.16525942056773424 ) ) ;
#17971=ADVANCED_FACE ( 'NONE', ( #5048 ), #9399, .F. ) ;
#17973=CARTESIAN_POINT ( 'NONE',  ( -4.243569643750004339, -23.82082603165501666, -5.466695036996486401 ) ) ;
#17980=CARTESIAN_POINT ( 'NONE',  ( 1.005564577543283766, -23.86805906247938935, -16.73400458965339865 ) ) ;
#17981=CARTESIAN_POINT ( 'NONE',  ( 9.000000000000005329, -10.00000000000000178, -3.713574246709346216 ) ) ;
#17982=CARTESIAN_POINT ( 'NONE',  ( 4.000000000000000888, -24.62619912695155477, -10.88837712936937230 ) ) ;
#17983=CARTESIAN_POINT ( 'NONE',  ( 4.730628863548789710E-15, -21.72540816142837983, -15.28859851726467589 ) ) ;
#17984=ORIENTED_EDGE ( 'NONE', *, *, #12476, .T. ) ;
#17986=CARTESIAN_POINT ( 'NONE',  ( 4.713407268011036227E-15, -17.48727574878303770, -8.745573750710319061 ) ) ;
#17988=VERTEX_POINT ( 'NONE', #7737 ) ;
#17990=CARTESIAN_POINT ( 'NONE',  ( -4.000000000000004441, -23.01196377286574091, -4.556692218940494143 ) ) ;
#17996=ORIENTED_EDGE ( 'NONE', *, *, #5856, .F. ) ;
#17997=CARTESIAN_POINT ( 'NONE',  ( -4.243569643750000786, -25.70703222455301784, -12.43196676332983408 ) ) ;
#17999=CARTESIAN_POINT ( 'NONE',  ( 3.999999999999996447, -22.15159911833918827, -3.327964152506997397 ) ) ;
#18000=ORIENTED_EDGE ( 'NONE', *, *, #947, .T. ) ;
#18003=( BOUNDED_CURVE ( )  B_SPLINE_CURVE ( 2, ( #1433, #12451, #8541, #9761, #16929 ),
 .UNSPECIFIED., .F., .T. ) 
 B_SPLINE_CURVE_WITH_KNOTS ( ( 3, 2, 3 ),
 ( 0.004713559543201377953, 0.005747126436781609116, 0.008620689655172418878 ),
 .UNSPECIFIED. ) 
 CURVE ( )  GEOMETRIC_REPRESENTATION_ITEM ( )  RATIONAL_B_SPLINE_CURVE ( ( 0.9604780343359251571, 0.9759059229421220838, 1.000000000000000000, 0.9330127018922191873, 0.9330127018922192983 ) ) 
 REPRESENTATION_ITEM ( '' )  );
#18005=CARTESIAN_POINT ( 'NONE',  ( -4.243569643750000786, -20.51258062284889760, -5.013521062237622949 ) ) ;
#18007=CARTESIAN_POINT ( 'NONE',  ( -5.330712181944245322E-15, -26.55907985683728967, -5.105836667743160362 ) ) ;
#18010=CARTESIAN_POINT ( 'NONE',  ( -1.999999999999996225, -21.50895469527046444, -12.47596756835385534 ) ) ;
#18015=CARTESIAN_POINT ( 'NONE',  ( -4.000000000000000888, -26.88465634578871999, -14.11378830476406065 ) ) ;
#18020=CARTESIAN_POINT ( 'NONE',  ( 4.713407268011036227E-15, -21.55249874071609995, -14.55131386360180734 ) ) ;
#18022=CARTESIAN_POINT ( 'NONE',  ( 2.121784821874994176, -23.21111423883506220, -2.460191299572788814 ) ) ;
#18024=DIRECTION ( 'NONE',  ( -0.000000000000000000, 1.000000000000000000, -0.000000000000000000 ) ) ;
#18025=CARTESIAN_POINT ( 'NONE',  ( -4.243569643750000786, -24.38422156821842535, -10.54279736118833988 ) ) ;
#18028=CARTESIAN_POINT ( 'NONE',  ( -3.999999999999997335, -18.75526198665626154, -6.530127861826874103 ) ) ;
#18031=VECTOR ( 'NONE', #2972, 1000.000000000000000 ) ;
#18038=CARTESIAN_POINT ( 'NONE',  ( 4.000000000000003553, -24.00348637926830264, -14.02536906707117659 ) ) ;
#18041=CARTESIAN_POINT ( 'NONE',  ( -4.243569643750005227, -26.11154692433198576, -8.738183513875661390 ) ) ;
#18048=CARTESIAN_POINT ( 'NONE',  ( 4.243569643749996345, -26.57399292614002562, -9.398624849583658403 ) ) ;
#18054=CARTESIAN_POINT ( 'NONE',  ( 3.579096709490575479E-14, -25.90245948233327056, -5.737278629507336802 ) ) ;
#18055=CARTESIAN_POINT ( 'NONE',  ( -2.121784821874996396, -19.61005822318693248, -10.13182066358236888 ) ) ;
#18056=FACE_OUTER_BOUND ( 'NONE', #10084, .T. ) ;
#18066=CARTESIAN_POINT ( 'NONE',  ( 4.243569643750000786, -21.96444597736247673, -7.086999674344137468 ) ) ;
#18070=AXIS2_PLACEMENT_3D ( 'NONE', #13348, #6303, #11857 ) ;
#18071=CARTESIAN_POINT ( 'NONE',  ( 4.243569643750000786, -26.57815143726116602, -13.67605393059374208 ) ) ;
#18072=CARTESIAN_POINT ( 'NONE',  ( -4.036928234951689731, -26.90731100780323715, -14.49060178547057021 ) ) ;
#18073=CARTESIAN_POINT ( 'NONE',  ( 1.071796769724495224, -23.10335607593069440, -15.68731904395727739 ) ) ;
#18075=CARTESIAN_POINT ( 'NONE',  ( 2.121784821874994176, -29.11536668052359289, -10.89233765547263211 ) ) ;
#18076=VERTEX_POINT ( 'NONE', #3484 ) ;
#18077=CARTESIAN_POINT ( 'NONE',  ( -4.000000000000000888, -23.72281623969865905, -9.598212659614208775 ) ) ;
#18079=CARTESIAN_POINT ( 'NONE',  ( -2.000000000000005773, -24.00085731285198065, -3.955819603412733976 ) ) ;
#18082=CARTESIAN_POINT ( 'NONE',  ( 4.000000000000003553, -23.55179493634679844, -13.38028683320035661 ) ) ;
#18084=AXIS2_PLACEMENT_3D ( 'NONE', #11065, #4114, #16930 ) ;
#18087=CARTESIAN_POINT ( 'NONE',  ( -1.071796769724496334, -23.59100161583038613, -2.436174684792825396 ) ) ;
#18091=EDGE_LOOP ( 'NONE', ( #14910, #7051, #1837, #12775 ) ) ;
#18092=CARTESIAN_POINT ( 'NONE',  ( 4.243569643750003451, -23.03330574846025058, -12.88497973756566672 ) ) ;
#18094=CARTESIAN_POINT ( 'NONE',  ( 1.999999999999994449, -23.37709293761528784, -3.064991754241682465 ) ) ;
#18095=ORIENTED_EDGE ( 'NONE', *, *, #813, .F. ) ;
#18098=LINE ( 'NONE', #9804, #16094 ) ;
#18100=CIRCLE ( 'NONE', #8889, 4.400000000000002132 ) ;
#18103=CARTESIAN_POINT ( 'NONE',  ( 2.121784821874994176, -25.53409880605677884, -5.777757078943218438 ) ) ;
#18106=CARTESIAN_POINT ( 'NONE',  ( 4.000000000000003553, -22.00313855819898734, -11.16857631362007020 ) ) ;
#18108=FACE_OUTER_BOUND ( 'NONE', #7392, .T. ) ;
#18109=ORIENTED_EDGE ( 'NONE', *, *, #8299, .F. ) ;
#18112=CARTESIAN_POINT ( 'NONE',  ( 4.243569643750000786, -20.64163532102788778, -5.197830272202643265 ) ) ;
#18117=CARTESIAN_POINT ( 'NONE',  ( -1.999999999999996225, -21.44442734547602569, -12.38381296236458162 ) ) ;
#18118=( BOUNDED_CURVE ( )  B_SPLINE_CURVE ( 2, ( #10778, #12346, #2455, #1057, #17770, #13746, #7898, #16548, #5121 ),
 .UNSPECIFIED., .F., .T. ) 
 B_SPLINE_CURVE_WITH_KNOTS ( ( 3, 2, 2, 2, 3 ),
 ( 0.4051724137931034808, 0.4080459770114942541, 0.4137931034482758563, 0.4195402298850574585, 0.4224137931034482873 ),
 .UNSPECIFIED. ) 
 CURVE ( )  GEOMETRIC_REPRESENTATION_ITEM ( )  RATIONAL_B_SPLINE_CURVE ( ( 0.9330127018922194093, 0.9330127018922200755, 1.000000000000000000, 0.8660254037844387076, 1.000000000000000000, 0.8660254037844387076, 1.000000000000000000, 0.9330127018922187432, 0.9330127018922194093 ) ) 
 REPRESENTATION_ITEM ( '' )  );
#18119=VERTEX_POINT ( 'NONE', #11911 ) ;
#18120=CARTESIAN_POINT ( 'NONE',  ( 4.243569643750003451, -18.38733661401680308, -6.249848178824808365 ) ) ;
#18122=DIRECTION ( 'NONE',  ( -0.000000000000000000, -0.5735764363510414965, -0.8191520442889950182 ) ) ;
#18123=CARTESIAN_POINT ( 'NONE',  ( -2.121784821874996396, -19.35194882682896633, -9.763202243652322920 ) ) ;
#18124=CARTESIAN_POINT ( 'NONE',  ( 4.299564228933482956E-15, -23.09182937521185863, -15.67085720930136006 ) ) ;
#18126=CARTESIAN_POINT ( 'NONE',  ( -5.577813053751546416E-15, -24.67643985033786791, -3.986341135846375838 ) ) ;
#18128=ORIENTED_EDGE ( 'NONE', *, *, #342, .F. ) ;
#18129=ORIENTED_EDGE ( 'NONE', *, *, #13411, .T. ) ;
#18131=CARTESIAN_POINT ( 'NONE',  ( 5.810221930991194676E-16, -23.67257551772223678, -16.50024865515073458 ) ) ;
#18132=EDGE_CURVE ( 'NONE', #14859, #4548, #17693, .T. ) ;
#18133=CARTESIAN_POINT ( 'NONE',  ( 1.071796769724487675, -30.08521047313637453, -11.71086611972146407 ) ) ;
#18135=ORIENTED_EDGE ( 'NONE', *, *, #11135, .F. ) ;
#18137=CARTESIAN_POINT ( 'NONE',  ( -4.243569643750000786, -24.64233096457639505, -10.91141578111838584 ) ) ;
#18143=CARTESIAN_POINT ( 'NONE',  ( 0.000000000000000000, -2.372474330222551941, 20.89323558166710626 ) ) ;
#18145=CARTESIAN_POINT ( 'NONE',  ( -4.243569643749997233, -21.65672230121773723, -10.91901483127208294 ) ) ;
#18149=CARTESIAN_POINT ( 'NONE',  ( -2.121784821874996396, -18.57762063775506078, -8.657346983862177936 ) ) ;
#18150=CARTESIAN_POINT ( 'NONE',  ( -1.071796769724494114, -30.04373652477960732, -11.65163518304401613 ) ) ;
#18151=DIRECTION ( 'NONE',  ( 0.8191520442889951292, 0.4698463103929522156, -0.3289899283371602867 ) ) ;
#18158=AXIS2_PLACEMENT_3D ( 'NONE', #8757, #12846, #1638 ) ;
#18159=CARTESIAN_POINT ( 'NONE',  ( 2.121784821875004390, -18.65290254502614431, -8.764860689675106897 ) ) ;
#18162=CARTESIAN_POINT ( 'NONE',  ( 8.500000000000019540, 10.00000000000000000, -20.49999999999998934 ) ) ;
#18164=CARTESIAN_POINT ( 'NONE',  ( -8.500000000000005329, 0.000000000000000000, -20.49999999999999645 ) ) ;
#18167=CARTESIAN_POINT ( 'NONE',  ( -4.243569643750000786, -26.19098734272420614, -13.12312630069867225 ) ) ;
#18171=CARTESIAN_POINT ( 'NONE',  ( -2.000000000000005773, -24.51707610556791650, -4.693056443272829448 ) ) ;
#18179=VERTEX_POINT ( 'NONE', #3575 ) ;
#18180=CARTESIAN_POINT ( 'NONE',  ( 4.730628863548789710E-15, -21.24145304325719152, -14.59743897989583594 ) ) ;
#18182=CARTESIAN_POINT ( 'NONE',  ( 3.999999999999996447, -22.66781791105512767, -4.065200992367092425 ) ) ;
#18183=ORIENTED_EDGE ( 'NONE', *, *, #10523, .T. ) ;
#18188=EDGE_CURVE ( 'NONE', #14057, #13289, #16467, .T. ) ;
#18191=EDGE_CURVE ( 'NONE', #5758, #4066, #14068, .T. ) ;
#18192=CARTESIAN_POINT ( 'NONE',  ( 2.121784821875004390, -19.94344952681598926, -10.60795278932534558 ) ) ;
#18196=EDGE_LOOP ( 'NONE', ( #8474, #6923, #16083, #5798, #690 ) ) ;
#18197=CARTESIAN_POINT ( 'NONE',  ( 2.000000000000004441, -22.06819172071273272, -13.27464081153562425 ) ) ;
#18203=EDGE_CURVE ( 'NONE', #17988, #5572, #16077, .T. ) ;
#18206=CARTESIAN_POINT ( 'NONE',  ( 1.999999999999994449, -29.37813640364300127, -11.63537001862205855 ) ) ;
#18209=CARTESIAN_POINT ( 'NONE',  ( 1.999999999999994449, -28.28117146841668728, -10.06874173291258856 ) ) ;
#18211=CARTESIAN_POINT ( 'NONE',  ( -5.330712181944245322E-15, -23.71987649689963362, -1.051034048512634156 ) ) ;
#18214=CARTESIAN_POINT ( 'NONE',  ( 4.243569643749997233, -24.47685408073152402, -6.403600187652020104 ) ) ;
#18216=CARTESIAN_POINT ( 'NONE',  ( 1.999999999999994449, -25.18385871212106863, -5.645320693752015728 ) ) ;
#18217=DIRECTION ( 'NONE',  ( 0.000000000000000000, 0.000000000000000000, 1.000000000000000000 ) ) ;
#18219=VERTEX_POINT ( 'NONE', #3180 ) ;
#18221=CARTESIAN_POINT ( 'NONE',  ( 0.000000000000000000, 5.977523610840987267, 32.81826849749789687 ) ) ;
#18222=CARTESIAN_POINT ( 'NONE',  ( 1.071796769724504328, -24.92302254597699118, -4.338497721120512907 ) ) ;
#18225=CARTESIAN_POINT ( 'NONE',  ( 2.121784821874994176, -27.56671030237578179, -8.680627135892345692 ) ) ;
#18227=( BOUNDED_CURVE ( )  B_SPLINE_CURVE ( 2, ( #15683, #10006, #2978, #11767, #102, #13162, #10090, #472, #10379 ),
 .UNSPECIFIED., .F., .F. ) 
 B_SPLINE_CURVE_WITH_KNOTS ( ( 3, 2, 2, 2, 3 ),
 ( 0.9568965517241379004, 0.9597701149425287293, 0.9655172413793103869, 0.9712643678160919336, 0.9741379310344827624 ),
 .UNSPECIFIED. ) 
 CURVE ( )  GEOMETRIC_REPRESENTATION_ITEM ( )  RATIONAL_B_SPLINE_CURVE ( ( 0.9330127018922194093, 0.9330127018922194093, 1.000000000000000000, 0.8660254037844387076, 1.000000000000000000, 0.8660254037844387076, 1.000000000000000000, 0.9330127018922194093, 0.9330127018922194093 ) ) 
 REPRESENTATION_ITEM ( '' )  );
#18230=DIRECTION ( 'NONE',  ( 0.000000000000000000, 0.8191520442889952403, -0.5735764363510411634 ) ) ;
#18231=CARTESIAN_POINT ( 'NONE',  ( -4.243569643750000786, -23.90026645004723704, -9.851637823819498152 ) ) ;
#18232=DIRECTION ( 'NONE',  ( 0.000000000000000000, 0.000000000000000000, 1.000000000000000000 ) ) ;
#18233=FACE_OUTER_BOUND ( 'NONE', #4358, .T. ) ;
#18234=CARTESIAN_POINT ( 'NONE',  ( -1.071796769724486786, -17.72453270077011922, -8.005563162103721098 ) ) ;
#18235=CARTESIAN_POINT ( 'NONE',  ( 4.243569643750003451, -20.41994811033581314, -9.152718235773933841 ) ) ;
#18237=CARTESIAN_POINT ( 'NONE',  ( -5.577813053751546416E-15, -25.19265864305380376, -4.723577975706471754 ) ) ;
#18239=CARTESIAN_POINT ( 'NONE',  ( -1.071796769724505882, -18.95055233276553608, -9.756500655764678953 ) ) ;
#18245=ORIENTED_EDGE ( 'NONE', *, *, #12602, .T. ) ;
#18246=CARTESIAN_POINT ( 'NONE',  ( 4.243569643749997233, -23.21857077348643372, -4.606585390493036947 ) ) ;
#18248=( BOUNDED_CURVE ( )  B_SPLINE_CURVE ( 2, ( #4279, #10096, #15778, #12981, #12620, #4191, #8440, #14109, #1420 ),
 .UNSPECIFIED., .F., .T. ) 
 B_SPLINE_CURVE_WITH_KNOTS ( ( 3, 2, 2, 2, 3 ),
 ( 0.7844827586206897241, 0.7873563218390804419, 0.7931034482758620996, 0.7988505747126436463, 0.8017241379310344751 ),
 .UNSPECIFIED. ) 
 CURVE ( )  GEOMETRIC_REPRESENTATION_ITEM ( )  RATIONAL_B_SPLINE_CURVE ( ( 0.9330127018922194093, 0.9330127018922206306, 1.000000000000000000, 0.8660254037844387076, 1.000000000000000000, 0.8660254037844387076, 1.000000000000000000, 0.9330127018922194093, 0.9330127018922194093 ) ) 
 REPRESENTATION_ITEM ( '' )  );
#18250=CARTESIAN_POINT ( 'NONE',  ( -5.330712181944246111E-15, -30.91467592037800927, -11.32627250406271457 ) ) ;
#18252=LINE ( 'NONE', #10996, #17493 ) ;
#18255=CARTESIAN_POINT ( 'NONE',  ( -2.121784821874996396, -23.22358977219849407, -15.29247854260303718 ) ) ;
#18256=VERTEX_POINT ( 'NONE', #8721 ) ;
#18258=CARTESIAN_POINT ( 'NONE',  ( -4.000000000000000888, -21.46435902227137760, -6.372801486233056423 ) ) ;
#18264=CARTESIAN_POINT ( 'NONE',  ( 4.000000000000003553, -21.68050181204657889, -10.70780328770074696 ) ) ;
#18267=CARTESIAN_POINT ( 'NONE',  ( 2.121784821875004390, -22.00832469767973620, -13.55690014876572569 ) ) ;
#18271=CARTESIAN_POINT ( 'NONE',  ( 0.000000000000000000, 4.000000000000007105, 4.000000000000000000 ) ) ;
#18272=CARTESIAN_POINT ( 'NONE',  ( 0.000000000000000000, 10.00000000000000000, 0.000000000000000000 ) ) ;
#18274=CARTESIAN_POINT ( 'NONE',  ( 2.121784821874994176, -25.27598940969881269, -5.409138659013170702 ) ) ;
#18275=ORIENTED_EDGE ( 'NONE', *, *, #9603, .F. ) ;
#18277=ORIENTED_EDGE ( 'NONE', *, *, #2644, .F. ) ;
#18279=CARTESIAN_POINT ( 'NONE',  ( 4.713407268011036227E-15, -20.84269790143662959, -13.53761320980093785 ) ) ;
#18281=CYLINDRICAL_SURFACE ( 'NONE', #7468, 2.000000000000001776 ) ;
#18285=CARTESIAN_POINT ( 'NONE',  ( 1.999999999999994449, -28.60380821456909572, -10.52951475883191357 ) ) ;
#18287=EDGE_CURVE ( 'NONE', #985, #8838, #3148, .T. ) ;
#18289=EDGE_CURVE ( 'NONE', #11559, #1834, #6134, .T. ) ;
#18291=CARTESIAN_POINT ( 'NONE',  ( 4.000000000000000888, -23.33565214516171338, -9.045285029719133618 ) ) ;
#18292=ORIENTED_EDGE ( 'NONE', *, *, #14355, .F. ) ;
#18294=CARTESIAN_POINT ( 'NONE',  ( -5.330712181944245322E-15, -23.97798589325759977, -1.419652468442682558 ) ) ;
#18295=VECTOR ( 'NONE', #12062, 1000.000000000000000 ) ;
#18297=DIRECTION ( 'NONE',  ( 0.000000000000000000, 0.8191520442889952403, -0.5735764363510413855 ) ) ;
#18298=ADVANCED_FACE ( 'NONE', ( #1989 ), #5949, .F. ) ;
#18299=CARTESIAN_POINT ( 'NONE',  ( 4.243569643750000786, -23.22272928460757413, -8.884014471503119736 ) ) ;
#18301=CARTESIAN_POINT ( 'NONE',  ( -5.577813053751546416E-15, -23.38589286854802296, -2.143249036196138047 ) ) ;
#18307=CARTESIAN_POINT ( 'NONE',  ( -4.000000000000004441, -27.98056965346157554, -11.65259680360068018 ) ) ;
#18308=CARTESIAN_POINT ( 'NONE',  ( -3.999999999999997335, -22.62690293202579284, -12.05940416077759103 ) ) ;
#18309=CARTESIAN_POINT ( 'NONE',  ( 1.071796769724485232, -26.21356952776684679, -6.181589820770747146 ) ) ;
#18310=VERTEX_POINT ( 'NONE', #7613 ) ;
#18314=CARTESIAN_POINT ( 'NONE',  ( -2.121784821874996396, -20.12627701590287543, -10.86905750344246435 ) ) ;
#18317=LINE ( 'NONE', #11235, #4018 ) ;
#18319=CARTESIAN_POINT ( 'NONE',  ( -2.121784821874996396, -20.67475948316355883, -11.65237164579381535 ) ) ;
#18325=( BOUNDED_CURVE ( )  B_SPLINE_CURVE ( 2, ( #11455, #7010, #5728, #17343, #17148, #2952, #17245, #12679, #5904 ),
 .UNSPECIFIED., .F., .F. ) 
 B_SPLINE_CURVE_WITH_KNOTS ( ( 3, 2, 2, 2, 3 ),
 ( 0.7844827586206897241, 0.7873563218390804419, 0.7931034482758620996, 0.7988505747126436463, 0.8017241379310344751 ),
 .UNSPECIFIED. ) 
 CURVE ( )  GEOMETRIC_REPRESENTATION_ITEM ( )  RATIONAL_B_SPLINE_CURVE ( ( 0.9330127018922194093, 0.9330127018922206306, 1.000000000000000000, 0.8660254037844387076, 1.000000000000000000, 0.8660254037844387076, 1.000000000000000000, 0.9330127018922194093, 0.9330127018922194093 ) ) 
 REPRESENTATION_ITEM ( '' )  );
#18326=CARTESIAN_POINT ( 'NONE',  ( -4.243569643750000786, -20.77069001920686375, -5.382139482167671574 ) ) ;
#18327=CYLINDRICAL_SURFACE ( 'NONE', #8558, 4.000000000000000000 ) ;
#18329=ORIENTED_EDGE ( 'NONE', *, *, #11981, .T. ) ;
#18332=CARTESIAN_POINT ( 'NONE',  ( 4.243569643750003451, -24.54969845206331058, -15.05061295465469762 ) ) ;
#18335=CARTESIAN_POINT ( 'NONE',  ( -9.996898113758209803, -9.916603943890297757, 4.932537101542136426 ) ) ;
#18341=CARTESIAN_POINT ( 'NONE',  ( -2.121784821874996396, -23.99791796127240318, -16.39833380239318217 ) ) ;
#18343=DIRECTION ( 'NONE',  ( -0.000000000000000000, 1.000000000000000000, -0.000000000000000000 ) ) ;
#18346=CARTESIAN_POINT ( 'NONE',  ( 4.898587196589413815E-16, 2.700915433685006750, 35.11257424290206330 ) ) ;
#18347=CARTESIAN_POINT ( 'NONE',  ( -2.121784821874996396, -22.96548037584052793, -14.92386012267298945 ) ) ;
#18348=ORIENTED_EDGE ( 'NONE', *, *, #11410, .T. ) ;
#18350=CARTESIAN_POINT ( 'NONE',  ( -4.000000000000000888, -22.23868721134528670, -7.478656746023200519 ) ) ;
#18352=VERTEX_POINT ( 'NONE', #7241 ) ;
#18355=LINE ( 'NONE', #15733, #14009 ) ;
#18357=ADVANCED_FACE ( 'NONE', ( #12900 ), #7527, .F. ) ;
#18358=ORIENTED_EDGE ( 'NONE', *, *, #684, .T. ) ;
#18359=CARTESIAN_POINT ( 'NONE',  ( -4.243569643749998122, -23.72159747208148772, -13.86796219071246483 ) ) ;
#18363=ADVANCED_FACE ( 'NONE', ( #17296 ), #208, .F. ) ;
#18365=CARTESIAN_POINT ( 'NONE',  ( 2.343145750507617642, 4.000000000000004441, 3.999999999999997335 ) ) ;
#18383=COLOUR_RGB('Dark Blue',0.08,0.2,0.34);
#18384=FILL_AREA_STYLE_COLOUR('',#18383);
#18385=FILL_AREA_STYLE('',(#18384));
#18386=SURFACE_STYLE_FILL_AREA(#18385);
#18387=SURFACE_SIDE_STYLE('',(#18386));
#18388=SURFACE_STYLE_USAGE(.BOTH.,#18387);
#18389=PRESENTATION_STYLE_ASSIGNMENT((#18388));
ENDSEC;
END-ISO-10303-21;
